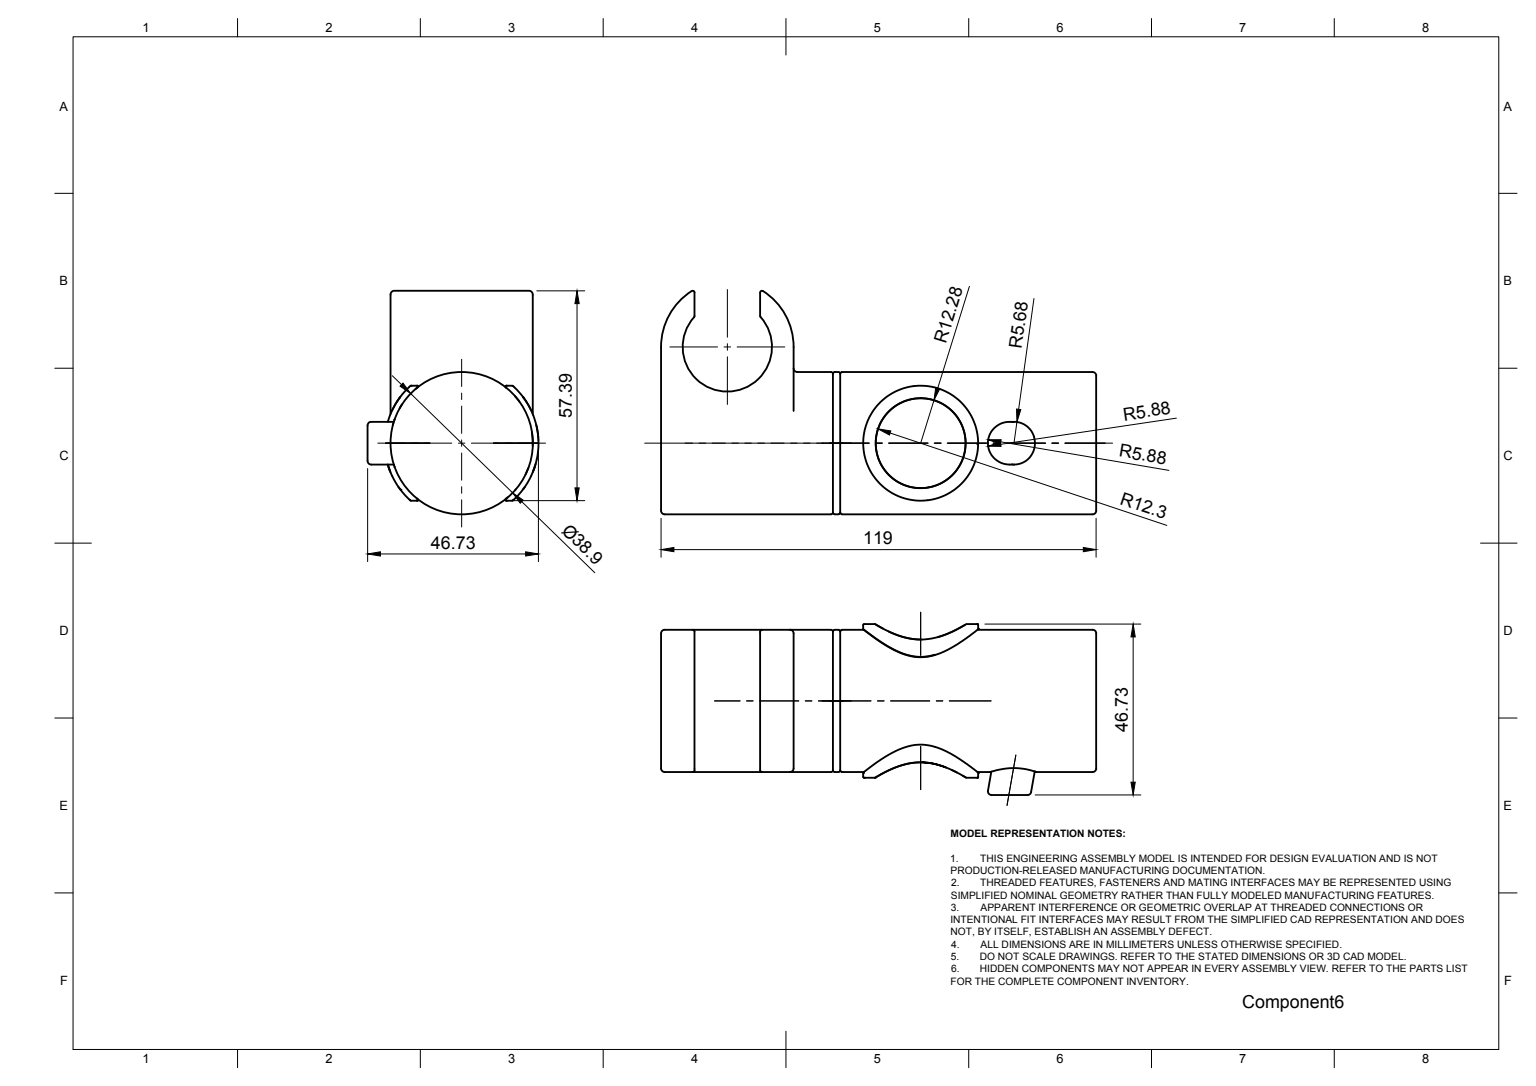
ISO-10303-21;
HEADER;
/* Generated by software containing ST-Developer
 * from STEP Tools, Inc. (www.steptools.com) 
 */

FILE_DESCRIPTION(
/* description */ ('STEP AP214'),
/* implementation_level */ '2;1');

FILE_NAME(
/* name */ 'Component6.step',
/* time_stamp */ '2026-10-06T11:02:40-07:00',
/* author */ (''),
/* organization */ (''),
/* preprocessor_version */ 'ST-DEVELOPER v20.2',
/* originating_system */ 'Autodesk Translation Framework v15.15.0.0',
/* authorisation */ '');

FILE_SCHEMA (('AUTOMOTIVE_DESIGN { 1 0 10303 214 3 1 1 }'));
ENDSEC;

DATA;
#10=MECHANICAL_DESIGN_GEOMETRIC_PRESENTATION_REPRESENTATION('',(#2941),#130910);
#43=(
BOUNDED_CURVE()
B_SPLINE_CURVE(3,(#103309,#103310,#103311,#103312,#103313,#103314,#103315,
#103316,#103317,#103318,#103319,#103320,#103321,#103322,#103323,#103324,
#103325,#103326),.UNSPECIFIED.,.F.,.F.)
B_SPLINE_CURVE_WITH_KNOTS((4,2,2,2,2,2,2,2,4),(0.,0.392699081698724,0.785398163397448,
1.17809724509617,1.5707963267949,1.96349540849362,2.35619449019234,2.74889357189107,
3.14159265358979),.UNSPECIFIED.)
CURVE()
GEOMETRIC_REPRESENTATION_ITEM()
RATIONAL_B_SPLINE_CURVE((1.,1.,1.,1.,1.,1.,1.,1.,1.,1.,1.,1.,1.,1.,1.,1.,
1.,1.))
REPRESENTATION_ITEM('')
);
#44=(
BOUNDED_CURVE()
B_SPLINE_CURVE(3,(#103476,#103477,#103478,#103479,#103480,#103481,#103482,
#103483,#103484,#103485,#103486,#103487,#103488,#103489,#103490,#103491,
#103492,#103493),.UNSPECIFIED.,.F.,.F.)
B_SPLINE_CURVE_WITH_KNOTS((4,2,2,2,2,2,2,2,4),(3.14159265358979,3.53429173528852,
3.92699081698724,4.31968989868597,4.71238898038469,5.10508806208341,5.49778714378214,
5.89048622548086,6.28318530717959),.UNSPECIFIED.)
CURVE()
GEOMETRIC_REPRESENTATION_ITEM()
RATIONAL_B_SPLINE_CURVE((1.,1.,1.,1.,1.,1.,1.,1.,1.,1.,1.,1.,1.,1.,1.,1.,
1.,1.))
REPRESENTATION_ITEM('')
);
#66=SPHERICAL_SURFACE('',#48870,0.5);
#67=SPHERICAL_SURFACE('',#48880,0.5);
#68=SPHERICAL_SURFACE('',#48882,0.5);
#69=SPHERICAL_SURFACE('',#48888,0.5);
#724=FACE_BOUND('',#15265,.T.);
#725=FACE_BOUND('',#15266,.T.);
#726=FACE_BOUND('',#15267,.T.);
#727=FACE_BOUND('',#15278,.T.);
#728=FACE_BOUND('',#15280,.T.);
#729=FACE_BOUND('',#15289,.T.);
#730=FACE_BOUND('',#15291,.T.);
#1660=(
BOUNDED_SURFACE()
B_SPLINE_SURFACE(3,2,((#97421,#97422,#97423),(#97424,#97425,#97426),(#97427,
#97428,#97429),(#97430,#97431,#97432),(#97433,#97434,#97435),(#97436,#97437,
#97438),(#97439,#97440,#97441),(#97442,#97443,#97444),(#97445,#97446,#97447),
(#97448,#97449,#97450),(#97451,#97452,#97453),(#97454,#97455,#97456),(#97457,
#97458,#97459),(#97460,#97461,#97462),(#97463,#97464,#97465),(#97466,#97467,
#97468),(#97469,#97470,#97471),(#97472,#97473,#97474),(#97475,#97476,#97477),
(#97478,#97479,#97480),(#97481,#97482,#97483),(#97484,#97485,#97486),(#97487,
#97488,#97489),(#97490,#97491,#97492),(#97493,#97494,#97495),(#97496,#97497,
#97498),(#97499,#97500,#97501),(#97502,#97503,#97504),(#97505,#97506,#97507),
(#97508,#97509,#97510),(#97511,#97512,#97513),(#97514,#97515,#97516),(#97517,
#97518,#97519),(#97520,#97521,#97522),(#97523,#97524,#97525),(#97526,#97527,
#97528),(#97529,#97530,#97531),(#97532,#97533,#97534),(#97535,#97536,#97537),
(#97538,#97539,#97540),(#97541,#97542,#97543),(#97544,#97545,#97546),(#97547,
#97548,#97549),(#97550,#97551,#97552),(#97553,#97554,#97555),(#97556,#97557,
#97558),(#97559,#97560,#97561),(#97562,#97563,#97564),(#97565,#97566,#97567),
(#97568,#97569,#97570),(#97571,#97572,#97573),(#97574,#97575,#97576),(#97577,
#97578,#97579),(#97580,#97581,#97582),(#97583,#97584,#97585),(#97586,#97587,
#97588),(#97589,#97590,#97591),(#97592,#97593,#97594),(#97595,#97596,#97597),
(#97598,#97599,#97600)),.UNSPECIFIED.,.F.,.F.,.F.)
B_SPLINE_SURFACE_WITH_KNOTS((4,2,2,2,2,2,2,2,2,2,2,2,2,2,2,2,2,2,2,2,2,
2,2,2,2,2,2,2,2,4),(3,3),(-0.00058262743669386,0.00319856320703094,0.00399820400878867,
0.00479784481054641,0.00639712641406187,0.00719676721581961,0.00799640801757734,
0.00959568962109281,0.0111949712246083,0.0127942528281237,0.0159928160351547,
0.0175920976386702,0.0191913792421856,0.0223899424492166,0.023989224052732,
0.0255885056562475,0.027187787259763,0.0279874280615207,0.0287870688632784,
0.0319856320703094,0.0335849136738248,0.0351841952773403,0.0367834768808558,
0.0383827584843712,0.0399820400878867,0.0415813216914022,0.0447798848984331,
0.0463791665019486,0.047978448105464,0.0517596387491888),(0.,1.00058262743669),
 .UNSPECIFIED.)
GEOMETRIC_REPRESENTATION_ITEM()
RATIONAL_B_SPLINE_SURFACE(((1.,0.372615622620617,1.00073106270323),(1.,
0.349888963005402,1.0007575450541),(1.,0.33336913321619,1.00077679486627),
(1.,0.327705676201969,1.00078339423716),(1.,0.327251477944985,1.00078392349389),
(1.,0.327438578938257,1.00078370547354),(1.,0.328073122498965,1.00078296606857),
(1.,0.331521383799571,1.00077894796528),(1.,0.335886927429418,1.00077386099429),
(1.,0.345028662937665,1.00076320854244),(1.,0.348522443164058,1.00075913739801),
(1.,0.356175477316151,1.00075021966266),(1.,0.360329629032238,1.00074537901713),
(1.,0.373578575616019,1.00072994061756),(1.,0.383450575672534,1.00071843722138),
(1.,0.404468341585455,1.00069394616722),(1.,0.415617057266219,1.00068095507195),
(1.,0.438646408868145,1.00065412000776),(1.,0.450439636237964,1.00064037789209),
(1.,0.485738524418637,1.00059924569062),(1.,0.509290450787533,1.00057180169364),
(1.,0.543406923368721,1.0005320473077),(1.,0.554585702870248,1.00051902118041),
(1.,0.576402400431413,1.00049359916725),(1.,0.586915261405066,1.00048134900477),
(1.,0.616896247011513,1.00044641351518),(1.,0.634916789357006,1.00042541499039),
(1.,0.658271057878159,1.00039820131519),(1.,0.665440397537911,1.00038984720721),
(1.,0.678364602785122,1.00037478721406),(1.,0.684003905064955,1.00036821598959),
(1.,0.693490447304963,1.00035716175002),(1.,0.697353099044676,1.00035266077625),
(1.,0.701751933579305,1.00034753501288),(1.,0.702985302217132,1.00034609782406),
(1.,0.704968511748717,1.00034378687949),(1.,0.705717903905829,1.00034291364662),
(1.,0.708180950178283,1.00034004356995),(1.,0.706146530160687,1.00034241418779),
(1.,0.69729017361677,1.00035273410042),(1.,0.693336856914947,1.00035734072197),
(1.,0.683762701080569,1.00036849705371),(1.,0.678128040418911,1.00037506286951),
(1.,0.665292401063798,1.00039001966082),(1.,0.658088068918505,1.00039841454396),
(1.,0.642209400675926,1.00041691723951),(1.,0.633656376746873,1.00042688369233),
(1.,0.615478575266067,1.00044806546409),(1.,0.605853070392858,1.00045928163056),
(1.,0.585652603574339,1.00048282032296),(1.,0.575043134289062,1.00049518305875),
(1.,0.542192039840224,1.00053346295665),(1.,0.519160353863195,1.00056030074098),
(1.,0.483909414581263,1.00060137706977),(1.,0.472043707472279,1.0006152036428),
(1.,0.448330324994361,1.0006428357773),(1.,0.43649600801918,1.00065662577283),
(1.,0.398029999848111,1.00070144847631),(1.,0.372846379395456,1.00073079381277),
(1.,0.353825408000619,1.00075295809239)))
REPRESENTATION_ITEM('')
SURFACE()
);
#1661=(
BOUNDED_SURFACE()
B_SPLINE_SURFACE(3,2,((#97849,#97850,#97851),(#97852,#97853,#97854),(#97855,
#97856,#97857),(#97858,#97859,#97860),(#97861,#97862,#97863),(#97864,#97865,
#97866),(#97867,#97868,#97869),(#97870,#97871,#97872),(#97873,#97874,#97875),
(#97876,#97877,#97878),(#97879,#97880,#97881),(#97882,#97883,#97884),(#97885,
#97886,#97887),(#97888,#97889,#97890),(#97891,#97892,#97893),(#97894,#97895,
#97896),(#97897,#97898,#97899),(#97900,#97901,#97902),(#97903,#97904,#97905),
(#97906,#97907,#97908),(#97909,#97910,#97911),(#97912,#97913,#97914),(#97915,
#97916,#97917),(#97918,#97919,#97920),(#97921,#97922,#97923),(#97924,#97925,
#97926),(#97927,#97928,#97929),(#97930,#97931,#97932),(#97933,#97934,#97935),
(#97936,#97937,#97938),(#97939,#97940,#97941),(#97942,#97943,#97944),(#97945,
#97946,#97947),(#97948,#97949,#97950),(#97951,#97952,#97953),(#97954,#97955,
#97956),(#97957,#97958,#97959),(#97960,#97961,#97962),(#97963,#97964,#97965),
(#97966,#97967,#97968),(#97969,#97970,#97971),(#97972,#97973,#97974),(#97975,
#97976,#97977),(#97978,#97979,#97980),(#97981,#97982,#97983),(#97984,#97985,
#97986),(#97987,#97988,#97989),(#97990,#97991,#97992),(#97993,#97994,#97995),
(#97996,#97997,#97998),(#97999,#98000,#98001),(#98002,#98003,#98004)),
 .UNSPECIFIED.,.F.,.F.,.F.)
B_SPLINE_SURFACE_WITH_KNOTS((4,2,2,2,2,2,2,2,2,2,2,2,2,2,2,2,2,2,2,2,2,
2,2,2,2,4),(3,3),(0.,0.00315886476497431,0.00473829714746146,0.00631772952994861,
0.00789716191243577,0.00947659429492292,0.0126354590598972,0.0142148914423844,
0.0157943238248715,0.0189531885898458,0.0221120533548201,0.0236914857373073,
0.0252709181197944,0.0268503505022816,0.0284297828847688,0.0315886476497431,
0.0331680800322302,0.0347475124147174,0.0363269447972045,0.0379063771796917,
0.041065241944666,0.0426446743271531,0.0442241067096403,0.0473829714746146,
0.0489624038571017,0.0509081571689574),(-0.000366320929394054,1.),
 .UNSPECIFIED.)
GEOMETRIC_REPRESENTATION_ITEM()
RATIONAL_B_SPLINE_SURFACE(((1.00005042977931,0.931167215319011,1.),(1.00004802363142,
0.934451422823265,1.),(1.00004766638974,0.934939030352376,1.),(1.00005016915153,
0.931522952280194,1.),(1.00005152792892,0.92966832525533,1.),(1.00005514272126,
0.924734410684191,1.),(1.00005739708062,0.921657382894737,1.),(1.00006270960761,
0.914406190616929,1.),(1.00006578664498,0.910206270369143,1.),(1.00007258454286,
0.900927660639692,1.),(1.00007629268405,0.89586633205052,1.),(1.0000882084061,
0.879602284474657,1.),(1.00009720731593,0.867319462069032,1.),(1.00011185421907,
0.847327561573564,1.),(1.00011692583641,0.840405192509689,1.),(1.00012717668813,
0.826413565365098,1.),(1.00013237821318,0.819313882232296,1.),(1.00014804138246,
0.797934856318314,1.),(1.00015859373613,0.783531702112416,1.),(1.00017861952009,
0.756198041441388,1.),(1.00018776819113,0.743710806479728,1.),(1.00019903767144,
0.728328829354908,1.),(1.00020239085733,0.723751987553838,1.),(1.00020800234017,
0.716092743446008,1.),(1.00021021837205,0.713068029719533,1.),(1.00021337561237,
0.708758638603594,1.),(1.00021431665381,0.707474189140747,1.),(1.00021485246247,
0.70674285137928,1.),(1.0002144426404,0.707302227096993,1.),(1.00021115809343,
0.711785382037871,1.),(1.00020631623579,0.718394146723749,1.),(1.00019606386371,
0.732387849048684,1.),(1.0001921234338,0.737766233939451,1.),(1.0001836019673,
0.74939738277055,1.),(1.00017901501663,0.755658218975225,1.),(1.00016939628292,
0.768787053474939,1.),(1.00016436417741,0.775655491921232,1.),(1.00015402891774,
0.789762329443024,1.),(1.00014872894768,0.796996382481174,1.),(1.00013293409498,
0.818555146164889,1.),(1.00012245640244,0.832856393646782,1.),(1.00010747739276,
0.853301594132862,1.),(1.0001025893796,0.859973357550685,1.),(1.00009330215817,
0.872649703192738,1.),(1.00008888539535,0.878678246012862,1.),(1.00007641546784,
0.895698741577217,1.),(1.00006912991505,0.905642962900587,1.),(1.00006026267051,
0.917746072269067,1.),(1.00005766031332,0.921298090426901,1.),(1.00005289421335,
0.927803451699111,1.),(1.00005093853036,0.930472809118457,1.),(1.00004972550474,
0.932128496152477,1.)))
REPRESENTATION_ITEM('')
SURFACE()
);
#1662=(
BOUNDED_SURFACE()
B_SPLINE_SURFACE(3,2,((#98299,#98300,#98301),(#98302,#98303,#98304),(#98305,
#98306,#98307),(#98308,#98309,#98310),(#98311,#98312,#98313),(#98314,#98315,
#98316),(#98317,#98318,#98319),(#98320,#98321,#98322),(#98323,#98324,#98325),
(#98326,#98327,#98328),(#98329,#98330,#98331),(#98332,#98333,#98334),(#98335,
#98336,#98337),(#98338,#98339,#98340),(#98341,#98342,#98343),(#98344,#98345,
#98346),(#98347,#98348,#98349),(#98350,#98351,#98352),(#98353,#98354,#98355),
(#98356,#98357,#98358),(#98359,#98360,#98361),(#98362,#98363,#98364),(#98365,
#98366,#98367),(#98368,#98369,#98370),(#98371,#98372,#98373),(#98374,#98375,
#98376),(#98377,#98378,#98379),(#98380,#98381,#98382),(#98383,#98384,#98385),
(#98386,#98387,#98388),(#98389,#98390,#98391),(#98392,#98393,#98394),(#98395,
#98396,#98397),(#98398,#98399,#98400),(#98401,#98402,#98403),(#98404,#98405,
#98406),(#98407,#98408,#98409),(#98410,#98411,#98412),(#98413,#98414,#98415),
(#98416,#98417,#98418),(#98419,#98420,#98421),(#98422,#98423,#98424),(#98425,
#98426,#98427),(#98428,#98429,#98430),(#98431,#98432,#98433),(#98434,#98435,
#98436),(#98437,#98438,#98439),(#98440,#98441,#98442),(#98443,#98444,#98445),
(#98446,#98447,#98448)),.UNSPECIFIED.,.F.,.F.,.F.)
B_SPLINE_SURFACE_WITH_KNOTS((4,2,2,2,2,2,2,2,2,2,2,2,2,2,2,2,2,2,2,2,2,
2,2,2,4),(3,3),(0.,0.0025187116162184,0.00377806742432761,0.00503742323243681,
0.00629677904054601,0.00755613484865521,0.0100748464648736,0.0113342022729828,
0.012593558081092,0.0151122696973104,0.0163716255054196,0.0176309813135288,
0.018890337121638,0.0201496929297472,0.0226684045459656,0.0239277603540748,
0.025187116162184,0.0264464719702932,0.0277058277784024,0.0302245393946208,
0.0327432510108392,0.0352619626270576,0.0365213184351669,0.0377806742432761,
0.0402993858594945),(0.,1.),.UNSPECIFIED.)
GEOMETRIC_REPRESENTATION_ITEM()
RATIONAL_B_SPLINE_SURFACE(((1.,0.444837807664136,1.),(1.,0.443889729175589,
1.),(1.,0.447748071183855,1.),(1.,0.459453142902776,1.),(1.,0.464367346379585,
1.),(1.,0.475717163519536,1.),(1.,0.48211295799902,1.),(1.,0.495944712524718,
1.),(1.,0.503380981743553,1.),(1.,0.518962657925113,1.),(1.,0.527139185789211,
1.),(1.,0.551895636149689,1.),(1.,0.568781778812327,1.),(1.,0.593444445481799,
1.),(1.,0.601597343431266,1.),(1.,0.61732836948322,1.),(1.,0.624889681210996,
1.),(1.,0.646485984307859,1.),(1.,0.659441840352202,1.),(1.,0.675982223306384,
1.),(1.,0.68102172685123,1.),(1.,0.689763664719054,1.),(1.,0.693504359158594,
1.),(1.,0.69968025928586,1.),(1.,0.702115682658639,1.),(1.,0.705612781075522,
1.),(1.,0.706675637348199,1.),(1.,0.707648224727786,1.),(1.,0.705356532405246,
1.),(1.,0.697802511437167,1.),(1.,0.69458157237586,1.),(1.,0.686829651284654,
1.),(1.,0.682347030399091,1.),(1.,0.672289714801745,1.),(1.,0.666714572428337,
1.),(1.,0.654569105179005,1.),(1.,0.647967838573232,1.),(1.,0.627025457575446,
1.),(1.,0.611679454062546,1.),(1.,0.579351199094756,1.),(1.,0.56222647842645,
1.),(1.,0.529022354961919,1.),(1.,0.512804015742491,1.),(1.,0.490778638607675,
1.),(1.,0.48379298434534,1.),(1.,0.471266214350623,1.),(1.,0.46570913806108,
1.),(1.,0.451670624760032,1.),(1.,0.445830006853561,1.),(1.,0.444857616465186,
1.)))
REPRESENTATION_ITEM('')
SURFACE()
);
#1663=(
BOUNDED_SURFACE()
B_SPLINE_SURFACE(3,2,((#99274,#99275,#99276),(#99277,#99278,#99279),(#99280,
#99281,#99282),(#99283,#99284,#99285),(#99286,#99287,#99288),(#99289,#99290,
#99291),(#99292,#99293,#99294),(#99295,#99296,#99297),(#99298,#99299,#99300),
(#99301,#99302,#99303),(#99304,#99305,#99306),(#99307,#99308,#99309),(#99310,
#99311,#99312),(#99313,#99314,#99315),(#99316,#99317,#99318),(#99319,#99320,
#99321),(#99322,#99323,#99324),(#99325,#99326,#99327),(#99328,#99329,#99330),
(#99331,#99332,#99333),(#99334,#99335,#99336),(#99337,#99338,#99339),(#99340,
#99341,#99342),(#99343,#99344,#99345),(#99346,#99347,#99348),(#99349,#99350,
#99351),(#99352,#99353,#99354),(#99355,#99356,#99357),(#99358,#99359,#99360),
(#99361,#99362,#99363),(#99364,#99365,#99366),(#99367,#99368,#99369),(#99370,
#99371,#99372),(#99373,#99374,#99375),(#99376,#99377,#99378),(#99379,#99380,
#99381),(#99382,#99383,#99384),(#99385,#99386,#99387),(#99388,#99389,#99390),
(#99391,#99392,#99393),(#99394,#99395,#99396),(#99397,#99398,#99399),(#99400,
#99401,#99402),(#99403,#99404,#99405),(#99406,#99407,#99408),(#99409,#99410,
#99411)),.UNSPECIFIED.,.F.,.F.,.F.)
B_SPLINE_SURFACE_WITH_KNOTS((4,2,2,2,2,2,2,2,2,2,2,2,2,2,2,2,2,2,2,2,2,
2,4),(3,3),(0.,0.00125459591840773,0.0018818938776116,0.00250919183681547,
0.0037637877552232,0.00439108571442707,0.00501838367363094,0.00564568163283481,
0.00627297959203867,0.00752757551044641,0.00878217142885414,0.0100367673472619,
0.0106640653064657,0.0112913632656696,0.0125459591840773,0.0138005551024851,
0.0144278530616889,0.0150551510208928,0.0163097469393006,0.0169370448985044,
0.0175643428577083,0.018818938776116,0.0200735346945238),(0.,1.),
 .UNSPECIFIED.)
GEOMETRIC_REPRESENTATION_ITEM()
RATIONAL_B_SPLINE_SURFACE(((1.,0.753501700966988,1.),(1.,0.758919966590289,
1.),(1.,0.762624474007346,1.),(1.,0.765493967892479,1.),(1.,0.766001864196328,
1.),(1.,0.766081899420437,1.),(1.,0.765645177532698,1.),(1.,0.762965796826428,
1.),(1.,0.75937217675435,1.),(1.,0.751475581705692,1.),(1.,0.748410443135639,
1.),(1.,0.741628592661977,1.),(1.,0.737899758372927,1.),(1.,0.729842420453465,
1.),(1.,0.725513701271151,1.),(1.,0.716322621401233,1.),(1.,0.71144077787533,
1.),(1.,0.696381444937169,1.),(1.,0.685722488457871,1.),(1.,0.663879284854164,
1.),(1.,0.652645530876282,1.),(1.,0.631293420609983,1.),(1.,0.621067849093089,
1.),(1.,0.607073245214128,1.),(1.,0.602619800288969,1.),(1.,0.594464909703987,
1.),(1.,0.590739984910806,1.),(1.,0.580731511515441,1.),(1.,0.575617470391927,
1.),(1.,0.569031517938587,1.),(1.,0.567674325666079,1.),(1.,0.568262977064503,
1.),(1.,0.568891116188093,1.),(1.,0.570935397635918,1.),(1.,0.572362568136071,
1.),(1.,0.577560685048605,1.),(1.,0.582247188120323,1.),(1.,0.59023516464793,
1.),(1.,0.593074756205356,1.),(1.,0.598856135494127,1.),(1.,0.601790038290455,
1.),(1.,0.610522818926502,1.),(1.,0.616249874441583,1.),(1.,0.626614400505202,
1.),(1.,0.631088239307343,1.),(1.,0.634563057406884,1.)))
REPRESENTATION_ITEM('')
SURFACE()
);
#1664=(
BOUNDED_SURFACE()
B_SPLINE_SURFACE(3,2,((#99754,#99755,#99756),(#99757,#99758,#99759),(#99760,
#99761,#99762),(#99763,#99764,#99765),(#99766,#99767,#99768),(#99769,#99770,
#99771),(#99772,#99773,#99774),(#99775,#99776,#99777),(#99778,#99779,#99780),
(#99781,#99782,#99783),(#99784,#99785,#99786),(#99787,#99788,#99789),(#99790,
#99791,#99792),(#99793,#99794,#99795),(#99796,#99797,#99798),(#99799,#99800,
#99801),(#99802,#99803,#99804),(#99805,#99806,#99807),(#99808,#99809,#99810),
(#99811,#99812,#99813),(#99814,#99815,#99816),(#99817,#99818,#99819),(#99820,
#99821,#99822),(#99823,#99824,#99825),(#99826,#99827,#99828),(#99829,#99830,
#99831),(#99832,#99833,#99834),(#99835,#99836,#99837),(#99838,#99839,#99840),
(#99841,#99842,#99843),(#99844,#99845,#99846),(#99847,#99848,#99849),(#99850,
#99851,#99852),(#99853,#99854,#99855),(#99856,#99857,#99858),(#99859,#99860,
#99861),(#99862,#99863,#99864),(#99865,#99866,#99867),(#99868,#99869,#99870),
(#99871,#99872,#99873),(#99874,#99875,#99876),(#99877,#99878,#99879),(#99880,
#99881,#99882),(#99883,#99884,#99885),(#99886,#99887,#99888),(#99889,#99890,
#99891),(#99892,#99893,#99894),(#99895,#99896,#99897),(#99898,#99899,#99900),
(#99901,#99902,#99903),(#99904,#99905,#99906),(#99907,#99908,#99909),(#99910,
#99911,#99912),(#99913,#99914,#99915)),.UNSPECIFIED.,.F.,.F.,.F.)
B_SPLINE_SURFACE_WITH_KNOTS((4,2,2,2,2,2,2,2,2,2,2,2,2,2,2,2,2,2,2,2,2,
2,2,2,2,2,4),(3,3),(-7.78153428745613E-5,0.00257554787859691,0.00386332181789536,
0.00515109575719382,0.00643886969649227,0.00772664363579073,0.0103021915143876,
0.0115899654536861,0.0128777393929845,0.0154532872715815,0.0167410612108799,
0.0180288351501784,0.0193166090894768,0.0206043830287753,0.0231799309073722,
0.0244677048466706,0.0257554787859691,0.0270432527252676,0.028331026664566,
0.0309065745431629,0.0321943484824614,0.0334821224217598,0.0347698963610583,
0.0360576703003567,0.0386332181789536,0.0399209921182521,0.0412865814003949),
(-5.57615391788296E-5,1.00007781534287),.UNSPECIFIED.)
GEOMETRIC_REPRESENTATION_ITEM()
RATIONAL_B_SPLINE_SURFACE(((1.00006499666788,0.417145519460541,1.00009070498426),
(1.00006613373744,0.406948903154154,1.00009229180215),(1.00006666002296,
0.402229463167758,1.00009302625088),(1.00006643124968,0.404280976494946,
1.00009270699026),(1.00006619616633,0.406389075066969,1.00009237892372),
(1.00006542207527,0.413330699283567,1.00009129865423),(1.00006489161556,
0.418087571101604,1.00009055838029),(1.00006360370812,0.429636818858515,
1.00008876106317),(1.00006284644101,0.436427575124811,1.00008770427205),
(1.00006116075035,0.451543924676617,1.00008535183539),(1.00006022957763,
0.459894171148586,1.00008405235327),(1.00005731845811,0.485999494820791,
1.0000799897904),(1.00005520865809,0.504919024658453,1.00007704549518),
(1.00005200598796,0.533638814326789,1.00007257606387),(1.00005092886496,
0.543297862838644,1.00007107290335),(1.00004879117353,0.562467507505169,
1.00006808968476),(1.00004774201681,0.571875769700711,1.00006662555212),
(1.00004468046442,0.599330092951599,1.00006235305522),(1.00004275366152,
0.616608604952205,1.0000596641385),(1.00004012772931,0.640156525218429,
1.00005599956388),(1.00003929341804,0.647638171228524,1.00005483525511),
(1.00003776153149,0.661375289848644,1.00005269745713),(1.00003706001501,
0.667666105061143,1.00005171846784),(1.00003579596344,0.679001426435143,
1.00004995444238),(1.00003523337831,0.684046381465567,1.00004916933635),
(1.00003426031965,0.692772237972241,1.00004781140104),(1.00003384837915,
0.696466294543873,1.00004723652454),(1.00003288787868,0.705079536093434,
1.0000458961146),(1.00003260121688,0.707650161916355,1.00004549606865),
(1.00003271698939,0.706611977550149,1.00004565763299),(1.0000328491286,
0.705427025561222,1.00004584203759),(1.0000332924415,0.701451638594737,
1.00004646069529),(1.00003360204356,0.6986752970103,1.00004689275514),(1.00003438648853,
0.691640824637982,1.00004798747386),(1.00003486136748,0.687382370582247,
1.00004865018302),(1.00003596953549,0.677444927484954,1.00005019666787),
(1.0000366053434,0.671743350745739,1.00005108395868),(1.00003869257694,
0.653026184786068,1.00005399676162),(1.00004033354564,0.638310877237478,
1.00005628678732),(1.00004309135935,0.613580315885842,1.00006013540692),
(1.00004405946053,0.604898915345222,1.0000614864239),(1.00004604481265,
0.587095366038472,1.00006425704798),(1.00004706626934,0.577935502541562,
1.00006568252433),(1.00004914915559,0.559257320686793,1.00006858926048),
(1.00005021068348,0.549738120586547,1.00007007065751),(1.00005235335541,
0.530523813480548,1.00007306082655),(1.00005343979317,0.520781235371959,
1.00007457698611),(1.00005663467271,0.492131307351429,1.00007903554542),
(1.00005869139382,0.4736877601911,1.00008190576725),(1.00006143077889,0.449122456788815,
1.00008572866908),(1.00006228506745,0.44146166545061,1.00008692085681),
(1.00006386334166,0.427308567599321,1.0000891233903),(1.00006457824779,
0.420897681437532,1.00009012106528),(1.00006512941961,0.415955074725545,
1.00009089024365)))
REPRESENTATION_ITEM('')
SURFACE()
);
#1665=(
BOUNDED_SURFACE()
B_SPLINE_SURFACE(3,2,((#100046,#100047,#100048),(#100049,#100050,#100051),
(#100052,#100053,#100054),(#100055,#100056,#100057),(#100058,#100059,#100060),
(#100061,#100062,#100063),(#100064,#100065,#100066),(#100067,#100068,#100069),
(#100070,#100071,#100072),(#100073,#100074,#100075),(#100076,#100077,#100078),
(#100079,#100080,#100081),(#100082,#100083,#100084),(#100085,#100086,#100087),
(#100088,#100089,#100090),(#100091,#100092,#100093),(#100094,#100095,#100096),
(#100097,#100098,#100099),(#100100,#100101,#100102),(#100103,#100104,#100105),
(#100106,#100107,#100108),(#100109,#100110,#100111),(#100112,#100113,#100114),
(#100115,#100116,#100117),(#100118,#100119,#100120),(#100121,#100122,#100123),
(#100124,#100125,#100126),(#100127,#100128,#100129),(#100130,#100131,#100132),
(#100133,#100134,#100135),(#100136,#100137,#100138),(#100139,#100140,#100141),
(#100142,#100143,#100144),(#100145,#100146,#100147),(#100148,#100149,#100150),
(#100151,#100152,#100153),(#100154,#100155,#100156),(#100157,#100158,#100159),
(#100160,#100161,#100162),(#100163,#100164,#100165),(#100166,#100167,#100168),
(#100169,#100170,#100171),(#100172,#100173,#100174),(#100175,#100176,#100177),
(#100178,#100179,#100180),(#100181,#100182,#100183),(#100184,#100185,#100186),
(#100187,#100188,#100189),(#100190,#100191,#100192),(#100193,#100194,#100195),
(#100196,#100197,#100198),(#100199,#100200,#100201),(#100202,#100203,#100204),
(#100205,#100206,#100207)),.UNSPECIFIED.,.F.,.F.,.F.)
B_SPLINE_SURFACE_WITH_KNOTS((4,2,2,2,2,2,2,2,2,2,2,2,2,2,2,2,2,2,2,2,2,
2,2,2,2,2,4),(3,3),(-7.78153430528562E-5,0.00257554787859691,0.00386332181789536,
0.00515109575719382,0.00643886969649227,0.00772664363579073,0.0103021915143876,
0.0115899654536861,0.0128777393929845,0.0154532872715815,0.0167410612108799,
0.0180288351501784,0.0193166090894768,0.0206043830287753,0.0231799309073722,
0.0244677048466706,0.0257554787859691,0.0270432527252676,0.028331026664566,
0.0309065745431629,0.0321943484824614,0.0334821224217598,0.0347698963610583,
0.0360576703003567,0.0386332181789536,0.0399209921182521,0.0412865814005733),
(-5.57615387946816E-5,1.00007781534305),.UNSPECIFIED.)
GEOMETRIC_REPRESENTATION_ITEM()
RATIONAL_B_SPLINE_SURFACE(((1.00006499666744,0.417145519462717,1.00009070498446),
(1.00006613373698,0.406948903154911,1.00009229180236),(1.0000666600225,
0.402229463167788,1.00009302625109),(1.00006643124922,0.404280976495069,
1.00009270699047),(1.00006619616587,0.406389075067091,1.00009237892394),
(1.00006542207482,0.413330699283688,1.00009129865444),(1.00006489161511,
0.418087571101724,1.0000905583805),(1.00006360370768,0.429636818858632,
1.00008876106337),(1.00006284644058,0.436427575124927,1.00008770427225),
(1.00006116074993,0.45154392467673,1.00008535183558),(1.00006022957721,
0.459894171148698,1.00008405235346),(1.00005731845772,0.485999494820897,
1.00007998979058),(1.00005520865771,0.504919024658555,1.00007704549536),
(1.0000520059876,0.533638814326885,1.00007257606403),(1.00005092886461,
0.543297862838738,1.00007107290351),(1.00004879117319,0.562467507505259,
1.00006808968492),(1.00004774201649,0.571875769700799,1.00006662555227),
(1.00004468046411,0.599330092951681,1.00006235305536),(1.00004275366122,
0.616608604952284,1.00005966413864),(1.00004012772903,0.640156525218503,
1.00005599956401),(1.00003929341777,0.647638171228596,1.00005483525523),
(1.00003776153123,0.661375289848713,1.00005269745725),(1.00003706001475,
0.667666105061211,1.00005171846796),(1.00003579596319,0.679001426435209,
1.00004995444249),(1.00003523337806,0.684046381465632,1.00004916933646),
(1.00003426031941,0.692772237972305,1.00004781140115),(1.00003384837891,
0.696466294543935,1.00004723652465),(1.00003288787845,0.705079536093495,
1.00004589611471),(1.00003260121666,0.707650161916415,1.00004549606876),
(1.00003271698917,0.706611977550209,1.00004565763309),(1.00003284912838,
0.705427025561283,1.0000458420377),(1.00003329244127,0.701451638594799,
1.0000464606954),(1.00003360204333,0.698675297010362,1.00004689275525),
(1.00003438648829,0.691640824638045,1.00004798747396),(1.00003486136724,
0.687382370582311,1.00004865018313),(1.00003596953524,0.677444927485021,
1.00005019666798),(1.00003660534315,0.671743350745806,1.0000510839588),
(1.00003869257667,0.653026184786139,1.00005399676175),(1.00004033354536,
0.638310877237552,1.00005628678745),(1.00004309135906,0.613580315885922,
1.00006013540706),(1.00004405946023,0.604898915345303,1.00006148642404),
(1.00004604481234,0.587095366038557,1.00006425704813),(1.00004706626902,
0.577935502541649,1.00006568252448),(1.00004914915525,0.559257320686884,
1.00006858926064),(1.00005021068313,0.54973812058664,1.00007007065767),
(1.00005235335505,0.530523813480645,1.00007306082672),(1.0000534397928,
0.520781235372058,1.00007457698628),(1.00005663467232,0.492131307351533,
1.0000790355456),(1.00005869139341,0.473687760191208,1.00008190576744),
(1.00006143077847,0.449122456788928,1.00008572866928),(1.00006228506702,
0.441461665450725,1.000086920857),(1.00006386334123,0.427308567598488,1.00008912339051),
(1.00006457824735,0.420897681435977,1.00009012106548),(1.00006512941917,
0.415955074723729,1.00009089024386)))
REPRESENTATION_ITEM('')
SURFACE()
);
#1666=(
BOUNDED_SURFACE()
B_SPLINE_SURFACE(3,2,((#101435,#101436,#101437),(#101438,#101439,#101440),
(#101441,#101442,#101443),(#101444,#101445,#101446),(#101447,#101448,#101449),
(#101450,#101451,#101452),(#101453,#101454,#101455),(#101456,#101457,#101458),
(#101459,#101460,#101461),(#101462,#101463,#101464),(#101465,#101466,#101467),
(#101468,#101469,#101470),(#101471,#101472,#101473),(#101474,#101475,#101476),
(#101477,#101478,#101479),(#101480,#101481,#101482),(#101483,#101484,#101485),
(#101486,#101487,#101488),(#101489,#101490,#101491),(#101492,#101493,#101494),
(#101495,#101496,#101497),(#101498,#101499,#101500),(#101501,#101502,#101503),
(#101504,#101505,#101506),(#101507,#101508,#101509),(#101510,#101511,#101512),
(#101513,#101514,#101515),(#101516,#101517,#101518),(#101519,#101520,#101521),
(#101522,#101523,#101524),(#101525,#101526,#101527),(#101528,#101529,#101530),
(#101531,#101532,#101533),(#101534,#101535,#101536),(#101537,#101538,#101539),
(#101540,#101541,#101542),(#101543,#101544,#101545),(#101546,#101547,#101548),
(#101549,#101550,#101551),(#101552,#101553,#101554),(#101555,#101556,#101557),
(#101558,#101559,#101560),(#101561,#101562,#101563),(#101564,#101565,#101566),
(#101567,#101568,#101569),(#101570,#101571,#101572),(#101573,#101574,#101575),
(#101576,#101577,#101578),(#101579,#101580,#101581),(#101582,#101583,#101584),
(#101585,#101586,#101587),(#101588,#101589,#101590),(#101591,#101592,#101593),
(#101594,#101595,#101596),(#101597,#101598,#101599),(#101600,#101601,#101602),
(#101603,#101604,#101605),(#101606,#101607,#101608),(#101609,#101610,#101611),
(#101612,#101613,#101614)),.UNSPECIFIED.,.F.,.F.,.F.)
B_SPLINE_SURFACE_WITH_KNOTS((4,2,2,2,2,2,2,2,2,2,2,2,2,2,2,2,2,2,2,2,2,
2,2,2,2,2,2,2,2,4),(3,3),(-0.000582627436703559,0.00319856320703094,0.00399820400878867,
0.00479784481054641,0.00639712641406187,0.00719676721581961,0.00799640801757734,
0.00959568962109281,0.0111949712246083,0.0127942528281237,0.0159928160351547,
0.0175920976386702,0.0191913792421856,0.0223899424492166,0.023989224052732,
0.0255885056562475,0.027187787259763,0.0279874280615207,0.0287870688632784,
0.0319856320703094,0.0335849136738248,0.0351841952773403,0.0367834768808558,
0.0383827584843712,0.0399820400878867,0.0415813216914022,0.0447798848984331,
0.0463791665019486,0.047978448105464,0.0517596387491986),(-0.000582627436703563,
1.),.UNSPECIFIED.)
GEOMETRIC_REPRESENTATION_ITEM()
RATIONAL_B_SPLINE_SURFACE(((1.00073106270324,0.372615622620786,1.),(1.00075754505411,
0.34988896300548,1.),(1.00077679486628,0.333369133216196,1.),(1.00078339423717,
0.327705676201963,1.),(1.0007839234939,0.327251477944978,1.),(1.00078370547356,
0.327438578938251,1.),(1.00078296606858,0.328073122498959,1.),(1.0007789479653,
0.331521383799564,1.),(1.00077386099431,0.335886927429411,1.),(1.00076320854245,
0.345028662937659,1.),(1.00075913739802,0.348522443164051,1.),(1.00075021966268,
0.356175477316145,1.),(1.00074537901714,0.360329629032232,1.),(1.00072994061757,
0.373578575616013,1.),(1.00071843722139,0.383450575672528,1.),(1.00069394616724,
0.404468341585449,1.),(1.00068095507196,0.415617057266214,1.),(1.00065412000777,
0.438646408868139,1.),(1.0006403778921,0.450439636237959,1.),(1.00059924569063,
0.485738524418632,1.),(1.00057180169365,0.509290450787528,1.),(1.00053204730771,
0.543406923368716,1.),(1.00051902118042,0.554585702870244,1.),(1.00049359916726,
0.576402400431409,1.),(1.00048134900478,0.586915261405062,1.),(1.00044641351519,
0.616896247011509,1.),(1.0004254149904,0.634916789357002,1.),(1.00039820131519,
0.658271057878156,1.),(1.00038984720721,0.665440397537908,1.),(1.00037478721406,
0.678364602785118,1.),(1.0003682159896,0.684003905064952,1.),(1.00035716175002,
0.69349044730496,1.),(1.00035266077626,0.697353099044673,1.),(1.00034753501288,
0.701751933579303,1.),(1.00034609782407,0.702985302217129,1.),(1.00034378687949,
0.704968511748714,1.),(1.00034291364663,0.705717903905826,1.),(1.00034004356996,
0.70818095017828,1.),(1.0003424141878,0.706146530160684,1.),(1.00035273410042,
0.697290173616767,1.),(1.00035734072197,0.693336856914944,1.),(1.00036849705372,
0.683762701080566,1.),(1.00037506286951,0.678128040418907,1.),(1.00039001966083,
0.665292401063795,1.),(1.00039841454397,0.658088068918501,1.),(1.00041691723952,
0.642209400675922,1.),(1.00042688369234,0.633656376746869,1.),(1.0004480654641,
0.615478575266063,1.),(1.00045928163056,0.605853070392854,1.),(1.00048282032297,
0.585652603574335,1.),(1.00049518305876,0.575043134289058,1.),(1.00053346295666,
0.542192039840219,1.),(1.00056030074099,0.51916035386319,1.),(1.00060137706978,
0.483909414581257,1.),(1.00061520364281,0.472043707472274,1.),(1.00064283577731,
0.448330324994356,1.),(1.00065662577284,0.436496008019175,1.),(1.00070144847632,
0.398029999848035,1.),(1.00073079381278,0.37284637939532,1.),(1.0007529580924,
0.353825408000466,1.)))
REPRESENTATION_ITEM('')
SURFACE()
);
#1667=(
BOUNDED_SURFACE()
B_SPLINE_SURFACE(3,2,((#101803,#101804,#101805),(#101806,#101807,#101808),
(#101809,#101810,#101811),(#101812,#101813,#101814),(#101815,#101816,#101817),
(#101818,#101819,#101820),(#101821,#101822,#101823),(#101824,#101825,#101826),
(#101827,#101828,#101829),(#101830,#101831,#101832),(#101833,#101834,#101835),
(#101836,#101837,#101838),(#101839,#101840,#101841),(#101842,#101843,#101844),
(#101845,#101846,#101847),(#101848,#101849,#101850),(#101851,#101852,#101853),
(#101854,#101855,#101856),(#101857,#101858,#101859),(#101860,#101861,#101862),
(#101863,#101864,#101865),(#101866,#101867,#101868),(#101869,#101870,#101871),
(#101872,#101873,#101874),(#101875,#101876,#101877),(#101878,#101879,#101880),
(#101881,#101882,#101883),(#101884,#101885,#101886),(#101887,#101888,#101889),
(#101890,#101891,#101892),(#101893,#101894,#101895),(#101896,#101897,#101898),
(#101899,#101900,#101901),(#101902,#101903,#101904),(#101905,#101906,#101907),
(#101908,#101909,#101910),(#101911,#101912,#101913),(#101914,#101915,#101916),
(#101917,#101918,#101919),(#101920,#101921,#101922),(#101923,#101924,#101925),
(#101926,#101927,#101928),(#101929,#101930,#101931),(#101932,#101933,#101934),
(#101935,#101936,#101937),(#101938,#101939,#101940),(#101941,#101942,#101943),
(#101944,#101945,#101946),(#101947,#101948,#101949),(#101950,#101951,#101952),
(#101953,#101954,#101955),(#101956,#101957,#101958)),.UNSPECIFIED.,.F.,
 .F.,.F.)
B_SPLINE_SURFACE_WITH_KNOTS((4,2,2,2,2,2,2,2,2,2,2,2,2,2,2,2,2,2,2,2,2,
2,2,2,2,4),(3,3),(0.,0.00315886476497431,0.00473829714746146,0.00631772952994861,
0.00789716191243577,0.00947659429492292,0.0126354590598972,0.0142148914423844,
0.0157943238248715,0.0189531885898458,0.0221120533548201,0.0236914857373073,
0.0252709181197944,0.0268503505022816,0.0284297828847688,0.0315886476497431,
0.0331680800322302,0.0347475124147174,0.0363269447972045,0.0379063771796917,
0.041065241944666,0.0426446743271531,0.0442241067096403,0.0473829714746146,
0.0489624038571017,0.0509081571686288),(0.,1.00036632092907),
 .UNSPECIFIED.)
GEOMETRIC_REPRESENTATION_ITEM()
RATIONAL_B_SPLINE_SURFACE(((1.,0.931167215319034,1.00005042977927),(1.,
0.934451422823286,1.00004802363138),(1.,0.934939030352398,1.00004766638969),
(1.,0.931522952280216,1.00005016915148),(1.,0.929668325255353,1.00005152792887),
(1.,0.924734410684215,1.00005514272121),(1.,0.921657382894763,1.00005739708057),
(1.,0.914406190616957,1.00006270960755),(1.,0.910206270369172,1.00006578664493),
(1.,0.900927660639724,1.0000725845428),(1.,0.895866332050554,1.00007629268398),
(1.,0.879602284474697,1.00008820840602),(1.,0.867319462069075,1.00009720731585),
(1.,0.847327561573614,1.00011185421897),(1.,0.840405192509742,1.00011692583631),
(1.,0.826413565365155,1.00012717668802),(1.,0.819313882232356,1.00013237821306),
(1.,0.797934856318381,1.00014804138233),(1.,0.783531702112487,1.00015859373599),
(1.,0.756198041441468,1.00017861951993),(1.,0.743710806479812,1.00018776819096),
(1.,0.728328829354997,1.00019903767126),(1.,0.723751987553928,1.00020239085714),
(1.,0.716092743446101,1.00020800233998),(1.,0.713068029719627,1.00021021837186),
(1.,0.708758638603689,1.00021337561218),(1.,0.707474189140843,1.00021431665362),
(1.,0.706742851379377,1.00021485246228),(1.,0.70730222709709,1.00021444264021),
(1.,0.711785382037965,1.00021115809324),(1.,0.718394146723841,1.0002063162356),
(1.,0.732387849048772,1.00019606386353),(1.,0.737766233939537,1.00019212343363),
(1.,0.749397382770632,1.00018360196714),(1.,0.755658218975305,1.00017901501647),
(1.,0.768787053475015,1.00016939628277),(1.,0.775655491921306,1.00016436417726),
(1.,0.789762329443093,1.00015402891761),(1.,0.79699638248124,1.00014872894755),
(1.,0.818555146164949,1.00013293409486),(1.,0.832856393646837,1.00012245640233),
(1.,0.85330159413291,1.00010747739266),(1.,0.859973357550731,1.00010258937951),
(1.,0.872649703192779,1.00009330215809),(1.,0.878678246012902,1.00008888539527),
(1.,0.895698741577251,1.00007641546778),(1.,0.905642962900618,1.00006912991499),
(1.,0.917746072269094,1.00006026267045),(1.,0.921298090426927,1.00005766031327),
(1.,0.927803451698529,1.0000528942133),(1.,0.930472809117578,1.00005093853032),
(1.,0.93212849615166,1.00004972550469)))
REPRESENTATION_ITEM('')
SURFACE()
);
#1668=(
BOUNDED_SURFACE()
B_SPLINE_SURFACE(3,2,((#102253,#102254,#102255),(#102256,#102257,#102258),
(#102259,#102260,#102261),(#102262,#102263,#102264),(#102265,#102266,#102267),
(#102268,#102269,#102270),(#102271,#102272,#102273),(#102274,#102275,#102276),
(#102277,#102278,#102279),(#102280,#102281,#102282),(#102283,#102284,#102285),
(#102286,#102287,#102288),(#102289,#102290,#102291),(#102292,#102293,#102294),
(#102295,#102296,#102297),(#102298,#102299,#102300),(#102301,#102302,#102303),
(#102304,#102305,#102306),(#102307,#102308,#102309),(#102310,#102311,#102312),
(#102313,#102314,#102315),(#102316,#102317,#102318),(#102319,#102320,#102321),
(#102322,#102323,#102324),(#102325,#102326,#102327),(#102328,#102329,#102330),
(#102331,#102332,#102333),(#102334,#102335,#102336),(#102337,#102338,#102339),
(#102340,#102341,#102342),(#102343,#102344,#102345),(#102346,#102347,#102348),
(#102349,#102350,#102351),(#102352,#102353,#102354),(#102355,#102356,#102357),
(#102358,#102359,#102360),(#102361,#102362,#102363),(#102364,#102365,#102366),
(#102367,#102368,#102369),(#102370,#102371,#102372),(#102373,#102374,#102375),
(#102376,#102377,#102378),(#102379,#102380,#102381),(#102382,#102383,#102384),
(#102385,#102386,#102387),(#102388,#102389,#102390),(#102391,#102392,#102393),
(#102394,#102395,#102396),(#102397,#102398,#102399),(#102400,#102401,#102402)),
 .UNSPECIFIED.,.F.,.F.,.F.)
B_SPLINE_SURFACE_WITH_KNOTS((4,2,2,2,2,2,2,2,2,2,2,2,2,2,2,2,2,2,2,2,2,
2,2,2,4),(3,3),(0.,0.0025187116162184,0.00377806742432761,0.00503742323243681,
0.00629677904054601,0.00755613484865521,0.0100748464648736,0.0113342022729828,
0.012593558081092,0.0151122696973104,0.0163716255054196,0.0176309813135288,
0.018890337121638,0.0201496929297472,0.0226684045459656,0.0239277603540748,
0.025187116162184,0.0264464719702932,0.0277058277784024,0.0302245393946208,
0.0327432510108392,0.0352619626270576,0.0365213184351669,0.0377806742432761,
0.0402993858594945),(0.,1.),.UNSPECIFIED.)
GEOMETRIC_REPRESENTATION_ITEM()
RATIONAL_B_SPLINE_SURFACE(((1.,0.444837807664136,1.),(1.,0.443889729175589,
1.),(1.,0.447748071183855,1.),(1.,0.459453142902776,1.),(1.,0.464367346379585,
1.),(1.,0.475717163519536,1.),(1.,0.48211295799902,1.),(1.,0.495944712524718,
1.),(1.,0.503380981743553,1.),(1.,0.518962657925113,1.),(1.,0.527139185789211,
1.),(1.,0.551895636149689,1.),(1.,0.568781778812327,1.),(1.,0.593444445481799,
1.),(1.,0.601597343431266,1.),(1.,0.61732836948322,1.),(1.,0.624889681210996,
1.),(1.,0.646485984307859,1.),(1.,0.659441840352202,1.),(1.,0.675982223306384,
1.),(1.,0.68102172685123,1.),(1.,0.689763664719054,1.),(1.,0.693504359158594,
1.),(1.,0.69968025928586,1.),(1.,0.702115682658639,1.),(1.,0.705612781075522,
1.),(1.,0.706675637348199,1.),(1.,0.707648224727786,1.),(1.,0.705356532405246,
1.),(1.,0.697802511437167,1.),(1.,0.69458157237586,1.),(1.,0.686829651284654,
1.),(1.,0.682347030399091,1.),(1.,0.672289714801745,1.),(1.,0.666714572428337,
1.),(1.,0.654569105179005,1.),(1.,0.647967838573232,1.),(1.,0.627025457575446,
1.),(1.,0.611679454062546,1.),(1.,0.579351199094756,1.),(1.,0.56222647842645,
1.),(1.,0.529022354961919,1.),(1.,0.512804015742491,1.),(1.,0.490778638607675,
1.),(1.,0.48379298434534,1.),(1.,0.471266214350623,1.),(1.,0.46570913806108,
1.),(1.,0.451670624760032,1.),(1.,0.445830006853561,1.),(1.,0.444857616465186,
1.)))
REPRESENTATION_ITEM('')
SURFACE()
);
#1669=(
BOUNDED_SURFACE()
B_SPLINE_SURFACE(3,2,((#103225,#103226,#103227),(#103228,#103229,#103230),
(#103231,#103232,#103233),(#103234,#103235,#103236),(#103237,#103238,#103239),
(#103240,#103241,#103242),(#103243,#103244,#103245),(#103246,#103247,#103248),
(#103249,#103250,#103251),(#103252,#103253,#103254),(#103255,#103256,#103257),
(#103258,#103259,#103260),(#103261,#103262,#103263),(#103264,#103265,#103266),
(#103267,#103268,#103269),(#103270,#103271,#103272),(#103273,#103274,#103275),
(#103276,#103277,#103278)),.UNSPECIFIED.,.F.,.F.,.F.)
B_SPLINE_SURFACE_WITH_KNOTS((4,2,2,2,2,2,2,2,4),(3,3),(0.,0.392699081698724,
0.785398163397448,1.17809724509617,1.5707963267949,1.96349540849362,2.35619449019234,
2.74889357189107,3.14159265358979),(0.,1.),.UNSPECIFIED.)
GEOMETRIC_REPRESENTATION_ITEM()
RATIONAL_B_SPLINE_SURFACE(((1.,0.766044443118988,1.),(1.,0.766049891332403,
1.),(1.,0.764573371724783,1.),(1.,0.758863530286151,1.),(1.,0.754625142483316,
1.),(1.,0.74389933443991,1.),(1.,0.737413012003865,1.),(1.,0.723033687231336,
1.),(1.,0.715143224098042,1.),(1.,0.699070338275054,1.),(1.,0.690892921248369,
1.),(1.,0.675524086364245,1.),(1.,0.668340746363067,1.),(1.,0.656206116553444,
1.),(1.,0.651264584058791,1.),(1.,0.644551763110563,1.),(1.,0.642777121345109,
1.),(1.,0.642787609686527,1.)))
REPRESENTATION_ITEM('')
SURFACE()
);
#1670=(
BOUNDED_SURFACE()
B_SPLINE_SURFACE(3,2,((#103526,#103527,#103528),(#103529,#103530,#103531),
(#103532,#103533,#103534),(#103535,#103536,#103537),(#103538,#103539,#103540),
(#103541,#103542,#103543),(#103544,#103545,#103546),(#103547,#103548,#103549),
(#103550,#103551,#103552),(#103553,#103554,#103555),(#103556,#103557,#103558),
(#103559,#103560,#103561),(#103562,#103563,#103564),(#103565,#103566,#103567),
(#103568,#103569,#103570),(#103571,#103572,#103573),(#103574,#103575,#103576),
(#103577,#103578,#103579)),.UNSPECIFIED.,.F.,.F.,.F.)
B_SPLINE_SURFACE_WITH_KNOTS((4,2,2,2,2,2,2,2,4),(3,3),(3.14159265358979,
3.53429173528852,3.92699081698724,4.31968989868597,4.71238898038469,5.10508806208341,
5.49778714378214,5.89048622548086,6.28318530717959),(0.,1.),
 .UNSPECIFIED.)
GEOMETRIC_REPRESENTATION_ITEM()
RATIONAL_B_SPLINE_SURFACE(((1.,0.642787609686527,1.),(1.,0.642777121345374,
1.),(1.,0.64455176311021,1.),(1.,0.651264584059143,1.),(1.,0.656206116553373,
1.),(1.,0.668340746363138,1.),(1.,0.675524086364297,1.),(1.,0.690892921248316,
1.),(1.,0.699070338275045,1.),(1.,0.71514322409805,1.),(1.,0.723033687231423,
1.),(1.,0.737413012003777,1.),(1.,0.74389933443967,1.),(1.,0.754625142483555,
1.),(1.,0.758863530286359,1.),(1.,0.764573371724574,1.),(1.,0.76604989133256,
1.),(1.,0.766044443118988,1.)))
REPRESENTATION_ITEM('')
SURFACE()
);
#1671=(
BOUNDED_SURFACE()
B_SPLINE_SURFACE(3,2,((#104053,#104054,#104055),(#104056,#104057,#104058),
(#104059,#104060,#104061),(#104062,#104063,#104064),(#104065,#104066,#104067),
(#104068,#104069,#104070),(#104071,#104072,#104073),(#104074,#104075,#104076),
(#104077,#104078,#104079),(#104080,#104081,#104082),(#104083,#104084,#104085),
(#104086,#104087,#104088),(#104089,#104090,#104091),(#104092,#104093,#104094),
(#104095,#104096,#104097),(#104098,#104099,#104100),(#104101,#104102,#104103),
(#104104,#104105,#104106),(#104107,#104108,#104109),(#104110,#104111,#104112),
(#104113,#104114,#104115),(#104116,#104117,#104118),(#104119,#104120,#104121),
(#104122,#104123,#104124),(#104125,#104126,#104127),(#104128,#104129,#104130),
(#104131,#104132,#104133),(#104134,#104135,#104136),(#104137,#104138,#104139),
(#104140,#104141,#104142),(#104143,#104144,#104145),(#104146,#104147,#104148),
(#104149,#104150,#104151),(#104152,#104153,#104154),(#104155,#104156,#104157),
(#104158,#104159,#104160),(#104161,#104162,#104163),(#104164,#104165,#104166),
(#104167,#104168,#104169),(#104170,#104171,#104172),(#104173,#104174,#104175),
(#104176,#104177,#104178),(#104179,#104180,#104181),(#104182,#104183,#104184),
(#104185,#104186,#104187),(#104188,#104189,#104190),(#104191,#104192,#104193),
(#104194,#104195,#104196),(#104197,#104198,#104199),(#104200,#104201,#104202)),
 .UNSPECIFIED.,.F.,.F.,.F.)
B_SPLINE_SURFACE_WITH_KNOTS((4,2,2,2,2,2,2,2,2,2,2,2,2,2,2,2,2,2,2,2,2,
2,2,2,4),(3,3),(0.0401498964591801,0.0428180974757128,0.044077453283822,
0.0453368090919312,0.0478555207081496,0.0503742323243681,0.0516335881324773,
0.0528929439405865,0.0554116555568049,0.0566710113649141,0.0579303671730233,
0.0604490787892417,0.0617084345973509,0.0629677904054601,0.0642271462135693,
0.0654865020216785,0.0680052136378969,0.0692645694460061,0.0705239252541153,
0.0717832810622245,0.0730426368703337,0.0755613484865521,0.0768207042946613,
0.0780800601027705,0.0807482611193032),(-0.000149489400314319,1.00005043309073),
 .UNSPECIFIED.)
GEOMETRIC_REPRESENTATION_ITEM()
RATIONAL_B_SPLINE_SURFACE(((1.00016593113143,0.444979039486126,1.00005597447691),
(1.00016643634691,0.443289150557816,1.00005614490407),(1.00016529660589,
0.447101455982151,1.00005576042886),(1.00016168673046,0.459176083043693,
1.00005454268938),(1.00016023845558,0.464020399532478,1.00005405413471),
(1.0001568480558,0.475360905223927,1.00005291043219),(1.00015492735237,
0.481785442045407,1.00005226251055),(1.00014872412617,0.502534535585041,
1.00005016994155),(1.00014399003011,0.518369554110557,1.00004857296244),
(1.00013406108711,0.551580751016643,1.00004522357655),(1.00012899351324,
0.568531215324515,1.00004351410351),(1.00012163222129,0.593153908442809,
1.00004103087771),(1.00011921529229,0.601238263928208,1.00004021556153),
(1.00011450349337,0.616998701048742,1.00003862610404),(1.00011220865661,
0.624674671757922,1.00003785197391),(1.00010570995292,0.646412104231448,
1.00003565972984),(1.00010183928869,0.659359040447713,1.00003435401702),
(1.00009691980327,0.675814165548792,1.00003269449948),(1.00009542797567,
0.680804160975152,1.00003219125293),(1.0000927816452,0.689655838565047,
1.00003129855147),(1.00009164983775,0.693441607130467,1.00003091675252),
(1.0000888664481,0.702751732254162,1.00002997781612),(1.00008780970836,
0.706286407750837,1.00002962134019),(1.000087517189,0.707264852088577,1.000029522663),
(1.00008764050632,0.706852369539625,1.00002956426232),(1.00008831781664,
0.704586842745149,1.0000297927432),(1.00008886935843,0.702741997522547,
1.00002997879788),(1.00009037928611,0.697691459383048,1.00003048815023),
(1.00009133772998,0.694485572475585,1.00003081146747),(1.00009365026412,
0.686750406029988,1.00003159156755),(1.00009500848198,0.682207320168808,
1.00003204974277),(1.00009954618833,0.667029203085519,1.00003358047265),
(1.0001032112903,0.654769849490324,1.000034816842),(1.00010947933538,0.633803944091153,
1.00003693127671),(1.00011169564763,0.626390629056982,1.00003767891772),
(1.0001162633142,0.61111229843889,1.00003921975424),(1.00011862464285,0.603213919841106,
1.00004001631445),(1.00012345746406,0.587048676802423,1.00004164659706),
(1.00012592916457,0.578781116742047,1.00004248038963),(1.00013093264633,
0.562045033359206,1.00004416824212),(1.00013347588336,0.553538191714369,
1.0000450261665),(1.00014096760153,0.528479237548492,1.0000475533897),(1.00014581500858,
0.512265206506655,1.00004918859264),(1.00015235765643,0.490380785760463,
1.00005139566065),(1.00015441501403,0.483499156141063,1.0000520896806),
(1.00015816391477,0.470959505082299,1.00005335431825),(1.00015984343524,
0.465341698114523,1.00005392088029),(1.00016419732593,0.450778423751254,
1.0000553896026),(1.00016593013437,0.44498237454662,1.00005597414056),(1.00016604025919,
0.444614019388471,1.00005601128959)))
REPRESENTATION_ITEM('')
SURFACE()
);
#1672=(
BOUNDED_SURFACE()
B_SPLINE_SURFACE(3,2,((#104203,#104204,#104205),(#104206,#104207,#104208),
(#104209,#104210,#104211),(#104212,#104213,#104214),(#104215,#104216,#104217),
(#104218,#104219,#104220),(#104221,#104222,#104223),(#104224,#104225,#104226),
(#104227,#104228,#104229),(#104230,#104231,#104232),(#104233,#104234,#104235),
(#104236,#104237,#104238),(#104239,#104240,#104241),(#104242,#104243,#104244),
(#104245,#104246,#104247),(#104248,#104249,#104250),(#104251,#104252,#104253),
(#104254,#104255,#104256),(#104257,#104258,#104259),(#104260,#104261,#104262),
(#104263,#104264,#104265),(#104266,#104267,#104268),(#104269,#104270,#104271),
(#104272,#104273,#104274),(#104275,#104276,#104277),(#104278,#104279,#104280),
(#104281,#104282,#104283),(#104284,#104285,#104286),(#104287,#104288,#104289),
(#104290,#104291,#104292),(#104293,#104294,#104295),(#104296,#104297,#104298),
(#104299,#104300,#104301),(#104302,#104303,#104304),(#104305,#104306,#104307),
(#104308,#104309,#104310),(#104311,#104312,#104313),(#104314,#104315,#104316),
(#104317,#104318,#104319),(#104320,#104321,#104322),(#104323,#104324,#104325),
(#104326,#104327,#104328),(#104329,#104330,#104331),(#104332,#104333,#104334),
(#104335,#104336,#104337),(#104338,#104339,#104340),(#104341,#104342,#104343),
(#104344,#104345,#104346),(#104347,#104348,#104349),(#104350,#104351,#104352),
(#104353,#104354,#104355),(#104356,#104357,#104358),(#104359,#104360,#104361),
(#104362,#104363,#104364),(#104365,#104366,#104367),(#104368,#104369,#104370),
(#104371,#104372,#104373),(#104374,#104375,#104376)),.UNSPECIFIED.,.F.,
 .F.,.F.)
B_SPLINE_SURFACE_WITH_KNOTS((4,2,2,2,2,2,2,2,2,2,2,2,2,2,2,2,2,2,2,2,2,
2,2,2,2,2,2,2,4),(3,3),(0.0492257416356437,0.05212126862205,0.0537007010045366,
0.0568595657695099,0.0576492819607532,0.0584389981519965,0.0600184305344832,
0.0615978629169698,0.0631772952994565,0.0663361600644298,0.0679155924469164,
0.0694950248294031,0.0726538895943764,0.0734436057856197,0.074233321976863,
0.0758127543593496,0.0773921867418363,0.0781819029330796,0.0789716191243229,
0.0821304838892962,0.0852893486542695,0.0868687810367562,0.0884482134192428,
0.0900276458017295,0.0916070781842161,0.0947659429491894,0.096345375331676,
0.0979248077141627,0.102399767083081),(-0.00131609460394527,1.),
 .UNSPECIFIED.)
GEOMETRIC_REPRESENTATION_ITEM()
RATIONAL_B_SPLINE_SURFACE(((1.00019594420023,0.925558466828159,1.),(1.00018290788058,
0.930511119781782,1.),(1.0001751814063,0.933446499297356,1.),(1.00017321277706,
0.934194404970496,1.),(1.0001744476356,0.933725267517896,1.),(1.00018352032596,
0.930278444495986,1.),(1.00019661401617,0.925303995782883,1.),(1.00022056253643,
0.916205667977813,1.),(1.00022574524419,0.914236695630683,1.),(1.00023669726237,
0.910075893610628,1.),(1.00024248153479,0.907878379693053,1.),(1.00026068949453,
0.90096095913229,1.),(1.00027396619521,0.89591698256937,1.),(1.00030249814301,
0.885077356102603,1.),(1.00031775500613,0.879281092265426,1.),(1.0003500033902,
0.867029547437474,1.),(1.00036707393448,0.860544244548642,1.),(1.00041973886326,
0.840536211453396,1.),(1.00045688450781,0.826424139102216,1.),(1.00051343672853,
0.804939277545135,1.),(1.00053242174643,0.797726643344391,1.),(1.00057017087807,
0.783385299064109,1.),(1.00058872431045,0.776336629339777,1.),(1.00064219262702,
0.756023379667273,1.),(1.00067513352966,0.743508738794324,1.),(1.00070920004036,
0.730566466029059,1.),(1.00071565293189,0.728114935756786,1.),(1.00072756192772,
0.723590566538064,1.),(1.0007330434182,0.721508083078691,1.),(1.00074797494598,
0.715835418009637,1.),(1.00075591036059,0.712820659575825,1.),(1.000767275578,
0.708502878251978,1.),(1.00077070476305,0.707200090045197,1.),(1.00077216358358,
0.706645866767436,1.),(1.00077203127614,0.706696131940276,1.),(1.00077052239234,
0.707269374848357,1.),(1.00076915238989,0.707789855080943,1.),(1.00075935410316,
0.711512340799273,1.),(1.00074204927767,0.718086649909378,1.),(1.00069241079651,
0.736944899541594,1.),(1.00066105961441,0.748855586662284,1.),(1.00060901661395,
0.768627341787248,1.),(1.00059072235101,0.77557754995927,1.),(1.00055350269926,
0.789717738526475,1.),(1.00053461513014,0.796893350775199,1.),(1.00049682155246,
0.81125158063532,1.),(1.00047791391785,0.818434816002099,1.),(1.00044051452833,
0.832643289086462,1.),(1.00042195785068,0.839693191730224,1.),(1.0003679404696,
0.860215037543297,1.),(1.00033443596869,0.87294379610312,1.),(1.00028952640061,
0.890005475388769,1.),(1.00027544616487,0.895354724483665,1.),(1.00024937271555,
0.905260338122725,1.),(1.00023733657422,0.909833011429418,1.),(1.00019681928589,
0.925226011375529,1.),(1.00017807148057,0.932348525694257,1.),(1.00017411585802,
0.93385131376765,1.)))
REPRESENTATION_ITEM('')
SURFACE()
);
#1673=(
BOUNDED_SURFACE()
B_SPLINE_SURFACE(3,2,((#104377,#104378,#104379),(#104380,#104381,#104382),
(#104383,#104384,#104385),(#104386,#104387,#104388),(#104389,#104390,#104391),
(#104392,#104393,#104394),(#104395,#104396,#104397),(#104398,#104399,#104400),
(#104401,#104402,#104403),(#104404,#104405,#104406),(#104407,#104408,#104409),
(#104410,#104411,#104412),(#104413,#104414,#104415),(#104416,#104417,#104418),
(#104419,#104420,#104421),(#104422,#104423,#104424),(#104425,#104426,#104427),
(#104428,#104429,#104430),(#104431,#104432,#104433),(#104434,#104435,#104436),
(#104437,#104438,#104439),(#104440,#104441,#104442),(#104443,#104444,#104445),
(#104446,#104447,#104448),(#104449,#104450,#104451),(#104452,#104453,#104454),
(#104455,#104456,#104457),(#104458,#104459,#104460),(#104461,#104462,#104463),
(#104464,#104465,#104466),(#104467,#104468,#104469),(#104470,#104471,#104472),
(#104473,#104474,#104475),(#104476,#104477,#104478),(#104479,#104480,#104481),
(#104482,#104483,#104484),(#104485,#104486,#104487),(#104488,#104489,#104490),
(#104491,#104492,#104493),(#104494,#104495,#104496),(#104497,#104498,#104499),
(#104500,#104501,#104502),(#104503,#104504,#104505),(#104506,#104507,#104508),
(#104509,#104510,#104511),(#104512,#104513,#104514),(#104515,#104516,#104517),
(#104518,#104519,#104520),(#104521,#104522,#104523),(#104524,#104525,#104526),
(#104527,#104528,#104529),(#104530,#104531,#104532),(#104533,#104534,#104535),
(#104536,#104537,#104538),(#104539,#104540,#104541),(#104542,#104543,#104544)),
 .UNSPECIFIED.,.F.,.F.,.F.)
B_SPLINE_SURFACE_WITH_KNOTS((4,2,2,2,2,2,2,2,2,2,2,2,2,2,2,2,2,2,2,2,2,
2,2,2,2,2,2,4),(3,3),(0.0511475161399861,0.0543755745194946,0.0559748561230095,
0.0575741377265244,0.0591734193300392,0.0607727009335541,0.062371982537069,
0.0639712641405839,0.0671698273476136,0.0687691089511285,0.0703683905546434,
0.0735669537616731,0.0743665945634306,0.075166235365188,0.0767655169687029,
0.0783647985722178,0.0799640801757326,0.0831626433827624,0.0839622841845198,
0.0847619249862773,0.0863612065897922,0.087960488193307,0.0895597697968219,
0.0911590514003368,0.0927583330038517,0.0959568962108814,0.0991554594179112,
0.102525861223953),(0.,1.00017183859901),.UNSPECIFIED.)
GEOMETRIC_REPRESENTATION_ITEM()
RATIONAL_B_SPLINE_SURFACE(((0.999999999999999,0.363791624139497,1.00021865031197),
(1.,0.345907098152807,1.00022479681575),(1.,0.333093359896291,1.00022920060541),
(1.,0.326997783970327,1.00023129551587),(1.,0.327177805749954,1.00023123364649),
(1.,0.331655133124558,1.00022969489116),(1.,0.33594526264938,1.00022822047147),
(1.,0.347973250814003,1.0002240867262),(1.,0.355767139651311,1.00022140814432),
(1.,0.373420234385515,1.00021534117819),(1.,0.383300909504948,1.00021194541545),
(1.,0.404353607436141,1.00020471008321),(1.,0.415539518961281,1.00020086574048),
(1.,0.438608462395935,1.00019293747064),(1.,0.450347915466347,1.0001889028883),
(1.,0.48562633119133,1.00017677850123),(1.,0.509203616458581,1.0001686755259),
(1.,0.543403436110305,1.00015692182771),(1.,0.554652013302503,1.00015305594821),
(1.,0.576466905683596,1.00014555866713),(1.,0.58694153284502,1.00014195877661),
(1.,0.616911695858428,1.00013165871496),(1.,0.634969557244847,1.00012545263976),
(1.,0.654503005935658,1.00011873943885),(1.,0.65825654007911,1.00011744943475),
(1.,0.665435063621704,1.00011498233989),(1.,0.668871309120368,1.00011380138067),
(1.,0.678546034793369,1.00011047639806),(1.,0.684157382338495,1.00010854790585),
(1.,0.693634268435882,1.00010529091619),(1.,0.697500232426135,1.00010396227252),
(1.,0.703370534929454,1.00010194478341),(1.,0.705371444929301,1.00010125711626),
(1.,0.708290812429381,1.00010025379622),(1.,0.706260755280861,1.00010095148057),
(1.,0.69882470043928,1.00010350708307),(1.,0.697084750890873,1.00010410506405),
(1.,0.693165330790786,1.00010545207937),(1.,0.690982356485942,1.00010620231786),
(1.,0.68379338348011,1.00010867300396),(1.,0.678148780393404,1.00011061292534),
(1.,0.665272843129722,1.00011503809138),(1.,0.658004130630274,1.00011753618212),
(1.,0.642133827810631,1.00012299044333),(1.,0.6335794985508,1.00012593037124),
(1.,0.615382081200458,1.00013218440864),(1.,0.605738300581893,1.00013549875614),
(1.,0.585480053220422,1.00014246105383),(1.,0.57481870187419,1.00014612511719),
(1.,0.54200218601379,1.00015740340541),(1.,0.51896068005778,1.00016532224562),
(1.,0.471865311436787,1.00018150784994),(1.,0.447600125261933,1.00018984724114),
(1.,0.400739305781053,1.00020595223628),(1.,0.378121326325834,1.00021372552008),
(1.,0.360032870100529,1.00021994211003)))
REPRESENTATION_ITEM('')
SURFACE()
);
#1674=(
BOUNDED_SURFACE()
B_SPLINE_SURFACE(3,2,((#104546,#104547,#104548),(#104549,#104550,#104551),
(#104552,#104553,#104554),(#104555,#104556,#104557),(#104558,#104559,#104560),
(#104561,#104562,#104563),(#104564,#104565,#104566),(#104567,#104568,#104569),
(#104570,#104571,#104572),(#104573,#104574,#104575),(#104576,#104577,#104578),
(#104579,#104580,#104581),(#104582,#104583,#104584),(#104585,#104586,#104587),
(#104588,#104589,#104590),(#104591,#104592,#104593),(#104594,#104595,#104596),
(#104597,#104598,#104599),(#104600,#104601,#104602),(#104603,#104604,#104605),
(#104606,#104607,#104608),(#104609,#104610,#104611),(#104612,#104613,#104614),
(#104615,#104616,#104617),(#104618,#104619,#104620),(#104621,#104622,#104623),
(#104624,#104625,#104626),(#104627,#104628,#104629),(#104630,#104631,#104632),
(#104633,#104634,#104635),(#104636,#104637,#104638),(#104639,#104640,#104641),
(#104642,#104643,#104644),(#104645,#104646,#104647),(#104648,#104649,#104650),
(#104651,#104652,#104653),(#104654,#104655,#104656),(#104657,#104658,#104659),
(#104660,#104661,#104662),(#104663,#104664,#104665),(#104666,#104667,#104668),
(#104669,#104670,#104671),(#104672,#104673,#104674),(#104675,#104676,#104677),
(#104678,#104679,#104680),(#104681,#104682,#104683),(#104684,#104685,#104686),
(#104687,#104688,#104689),(#104690,#104691,#104692),(#104693,#104694,#104695)),
 .UNSPECIFIED.,.F.,.F.,.F.)
B_SPLINE_SURFACE_WITH_KNOTS((4,2,2,2,2,2,2,2,2,2,2,2,2,2,2,2,2,2,2,2,2,
2,2,2,4),(3,3),(0.0411832956025613,0.0424965399968198,0.0437843139361192,
0.0463598618147179,0.0476476357540172,0.0489354096933166,0.0515109575719153,
0.054086505450514,0.0553742793898133,0.0566620533291127,0.0592376012077114,
0.0618131490863101,0.0631009230256095,0.0643886969649088,0.0656764709042082,
0.0669642448435075,0.0695397927221063,0.0708275666614056,0.072115340600705,
0.0734031145400043,0.0746908884793037,0.0772664363579024,0.0785542102972017,
0.0798419842365011,0.0824175321150998),(-2.54704549892859E-5,1.),
 .UNSPECIFIED.)
GEOMETRIC_REPRESENTATION_ITEM()
RATIONAL_B_SPLINE_SURFACE(((1.00002969011113,0.41716567016007,1.),(1.00002994384796,
0.412184667121395,1.),(1.0000301347314,0.408437513003748,1.),(1.00003036746518,
0.403868812055419,1.),(1.00003041084928,0.403017156769614,1.),(1.00003031596223,
0.404879845196922,1.),(1.00002995641597,0.411937949549854,1.),(1.00002907725759,
0.42919634528864,1.),(1.0000287281148,0.436050223421914,1.),(1.0000279625118,
0.45107946022051,1.),(1.00002754420566,0.459291055676708,1.),(1.00002621873246,
0.485310873574663,1.),(1.00002523535442,0.504615162293121,1.),(1.00002327853494,
0.543028678709834,1.),(1.00002229863343,0.562264721202267,1.),(1.00002088610616,
0.58999346174123,1.),(1.00002042575008,0.599030522075286,1.),(1.00001954857755,
0.616249934281681,1.),(1.00001912948864,0.624476895847254,1.),(1.00001793948785,
0.647837310828753,1.),(1.0000172350414,0.661666008506602,1.),(1.00001606044591,
0.68472400830539,1.),(1.00001561170694,0.693533018117966,1.),(1.00001517175011,
0.702169629233436,1.),(1.00001506362195,0.704292248448626,1.),(1.00001493152404,
0.706885408022375,1.),(1.0000149083449,0.70734042817065,1.),(1.00001494501072,
0.706620656543938,1.),(1.00001500486264,0.705445728351282,1.),(1.00001520669394,
0.701483661229885,1.),(1.00001534974885,0.698675409330837,1.),(1.00001589553929,
0.687961222177015,1.),(1.0000164072945,0.677915166725478,1.),(1.00001736385409,
0.659137339788157,1.),(1.00001771630397,0.652218541517549,1.),(1.00001846671731,
0.637487486635047,1.),(1.00001886535688,0.629661957539986,1.),(1.00001970257416,
0.613226890341952,1.),(1.0000201411837,0.604616727276649,1.),(1.00002105184036,
0.586740001976879,1.),(1.00002152598384,0.577432286849769,1.),(1.00002296522561,
0.549179124901904,1.),(1.00002395181897,0.529811717588144,1.),(1.00002540634078,
0.501258599676148,1.),(1.00002588670869,0.491828695166698,1.),(1.00002682175625,
0.473473162191487,1.),(1.000027272038,0.464633866720484,1.),(1.0000285273913,
0.439990543645249,1.),(1.00002924391365,0.425924788916652,1.),(1.00002973290203,
0.416325659622527,1.)))
REPRESENTATION_ITEM('')
SURFACE()
);
#1675=(
BOUNDED_SURFACE()
B_SPLINE_SURFACE(3,2,((#104696,#104697,#104698),(#104699,#104700,#104701),
(#104702,#104703,#104704),(#104705,#104706,#104707),(#104708,#104709,#104710),
(#104711,#104712,#104713),(#104714,#104715,#104716),(#104717,#104718,#104719),
(#104720,#104721,#104722),(#104723,#104724,#104725),(#104726,#104727,#104728),
(#104729,#104730,#104731),(#104732,#104733,#104734),(#104735,#104736,#104737),
(#104738,#104739,#104740),(#104741,#104742,#104743),(#104744,#104745,#104746),
(#104747,#104748,#104749),(#104750,#104751,#104752),(#104753,#104754,#104755),
(#104756,#104757,#104758),(#104759,#104760,#104761),(#104762,#104763,#104764),
(#104765,#104766,#104767),(#104768,#104769,#104770),(#104771,#104772,#104773),
(#104774,#104775,#104776),(#104777,#104778,#104779),(#104780,#104781,#104782),
(#104783,#104784,#104785),(#104786,#104787,#104788),(#104789,#104790,#104791),
(#104792,#104793,#104794),(#104795,#104796,#104797),(#104798,#104799,#104800),
(#104801,#104802,#104803),(#104804,#104805,#104806),(#104807,#104808,#104809),
(#104810,#104811,#104812),(#104813,#104814,#104815),(#104816,#104817,#104818),
(#104819,#104820,#104821),(#104822,#104823,#104824),(#104825,#104826,#104827),
(#104828,#104829,#104830),(#104831,#104832,#104833),(#104834,#104835,#104836),
(#104837,#104838,#104839),(#104840,#104841,#104842),(#104843,#104844,#104845)),
 .UNSPECIFIED.,.F.,.F.,.F.)
B_SPLINE_SURFACE_WITH_KNOTS((4,2,2,2,2,2,2,2,2,2,2,2,2,2,2,2,2,2,2,2,2,
2,2,2,4),(3,3),(0.0411832956025262,0.0424965399968198,0.0437843139361192,
0.0463598618147179,0.0476476357540172,0.0489354096933166,0.0515109575719153,
0.054086505450514,0.0553742793898133,0.0566620533291127,0.0592376012077114,
0.0618131490863101,0.0631009230256095,0.0643886969649088,0.0656764709042082,
0.0669642448435075,0.0695397927221063,0.0708275666614056,0.072115340600705,
0.0734031145400043,0.0746908884793037,0.0772664363579024,0.0785542102972017,
0.0798419842365011,0.0824175321150998),(-2.54704550244023E-5,1.),
 .UNSPECIFIED.)
GEOMETRIC_REPRESENTATION_ITEM()
RATIONAL_B_SPLINE_SURFACE(((1.00002969011117,0.417165670160449,1.),(1.000029943848,
0.412184667121575,1.),(1.00003013473144,0.408437513003789,1.),(1.00003036746522,
0.403868812055398,1.),(1.00003041084932,0.403017156769593,1.),(1.00003031596227,
0.404879845196902,1.),(1.00002995641602,0.411937949549833,1.),(1.00002907725763,
0.42919634528862,1.),(1.00002872811484,0.436050223421894,1.),(1.00002796251184,
0.451079460220491,1.),(1.0000275442057,0.459291055676689,1.),(1.00002621873249,
0.485310873574645,1.),(1.00002523535446,0.504615162293104,1.),(1.00002327853497,
0.543028678709818,1.),(1.00002229863346,0.562264721202251,1.),(1.00002088610619,
0.589993461741216,1.),(1.00002042575011,0.599030522075271,1.),(1.00001954857758,
0.616249934281668,1.),(1.00001912948867,0.624476895847241,1.),(1.00001793948787,
0.64783731082874,1.),(1.00001723504143,0.66166600850659,1.),(1.00001606044593,
0.684724008305379,1.),(1.00001561170696,0.693533018117955,1.),(1.00001517175013,
0.702169629233425,1.),(1.00001506362197,0.704292248448615,1.),(1.00001493152406,
0.706885408022364,1.),(1.00001490834492,0.70734042817064,1.),(1.00001494501075,
0.706620656543927,1.),(1.00001500486266,0.705445728351272,1.),(1.00001520669396,
0.701483661229874,1.),(1.00001534974887,0.698675409330827,1.),(1.00001589553931,
0.687961222177005,1.),(1.00001640729452,0.677915166725467,1.),(1.00001736385411,
0.659137339788145,1.),(1.00001771630399,0.652218541517537,1.),(1.00001846671733,
0.637487486635034,1.),(1.00001886535691,0.629661957539973,1.),(1.00001970257419,
0.613226890341938,1.),(1.00002014118373,0.604616727276635,1.),(1.00002105184039,
0.586740001976865,1.),(1.00002152598387,0.577432286849754,1.),(1.00002296522565,
0.549179124901888,1.),(1.000023951819,0.529811717588127,1.),(1.00002540634081,
0.50125859967613,1.),(1.00002588670873,0.49182869516668,1.),(1.00002682175628,
0.473473162191469,1.),(1.00002727203804,0.464633866720466,1.),(1.00002852739134,
0.439990543645229,1.),(1.00002924391369,0.425924788916632,1.),(1.00002973290207,
0.416325659622506,1.)))
REPRESENTATION_ITEM('')
SURFACE()
);
#1676=(
BOUNDED_SURFACE()
B_SPLINE_SURFACE(3,2,((#105057,#105058,#105059),(#105060,#105061,#105062),
(#105063,#105064,#105065),(#105066,#105067,#105068),(#105069,#105070,#105071),
(#105072,#105073,#105074),(#105075,#105076,#105077),(#105078,#105079,#105080),
(#105081,#105082,#105083),(#105084,#105085,#105086),(#105087,#105088,#105089),
(#105090,#105091,#105092),(#105093,#105094,#105095),(#105096,#105097,#105098),
(#105099,#105100,#105101),(#105102,#105103,#105104),(#105105,#105106,#105107),
(#105108,#105109,#105110),(#105111,#105112,#105113),(#105114,#105115,#105116),
(#105117,#105118,#105119),(#105120,#105121,#105122),(#105123,#105124,#105125),
(#105126,#105127,#105128),(#105129,#105130,#105131),(#105132,#105133,#105134),
(#105135,#105136,#105137),(#105138,#105139,#105140),(#105141,#105142,#105143),
(#105144,#105145,#105146),(#105147,#105148,#105149),(#105150,#105151,#105152),
(#105153,#105154,#105155),(#105156,#105157,#105158),(#105159,#105160,#105161),
(#105162,#105163,#105164),(#105165,#105166,#105167),(#105168,#105169,#105170),
(#105171,#105172,#105173),(#105174,#105175,#105176),(#105177,#105178,#105179),
(#105180,#105181,#105182)),.UNSPECIFIED.,.F.,.F.,.F.)
B_SPLINE_SURFACE_WITH_KNOTS((4,2,2,2,2,2,2,2,2,2,2,2,2,2,2,2,2,2,2,2,4),
(3,3),(0.0200568639003605,0.0213281306129126,0.0225827265313192,0.0232100244905226,
0.0238373224497259,0.0250919183681325,0.0263465142865391,0.0269738122457424,
0.0276011102049457,0.0288557061233524,0.030110302041759,0.0313648979601656,
0.0326194938785723,0.0332467918377756,0.0338740897969789,0.0351286857153855,
0.0363832816337921,0.0376378775521988,0.0382651755114021,0.0388924734706054,
0.040147069389012),(-1.6670794163376E-5,1.),.UNSPECIFIED.)
GEOMETRIC_REPRESENTATION_ITEM()
RATIONAL_B_SPLINE_SURFACE(((1.00001218909147,0.634417792362364,1.),(1.00001207070658,
0.637968459699978,1.),(1.00001198539686,0.640527117559773,1.),(1.00001190087293,
0.643062207776934,1.),(1.00001189940874,0.643106122556049,1.),(1.00001195795143,
0.641350276625085,1.),(1.00001198783686,0.640453935716271,1.),(1.0000120665277,
0.638093795110533,1.),(1.00001211511354,0.636636580788178,1.),(1.00001228558705,
0.631523641684606,1.),(1.0000124323333,0.627122344191632,1.),(1.00001277455001,
0.616858384702073,1.),(1.00001296504766,0.611144870017612,1.),(1.00001325563189,
0.602429501679159,1.),(1.00001335337752,0.599497858598228,1.),(1.00001354628551,
0.593712051753561,1.),(1.0000136417071,0.590850112792402,1.),(1.00001391054031,
0.582787113346938,1.),(1.00001406873562,0.578042429230547,1.),(1.00001430529436,
0.570947423996434,1.),(1.00001438238684,0.568635222351684,1.),(1.00001441730522,
0.56758793028365,1.),(1.00001437708325,0.568794290657144,1.),(1.00001416717897,
0.575089859693509,1.),(1.0000139997862,0.580110399619696,1.),(1.00001367027674,
0.589993235888577,1.),(1.00001354728695,0.593682016041953,1.),(1.00001327743302,
0.601775629678951,1.),(1.0000131303487,0.606187066817002,1.),(1.00001266743157,
0.620071142126849,1.),(1.00001232742341,0.630268861450101,1.),(1.00001161384565,
0.6516708939964,1.),(1.0000112397551,0.662890831923292,1.),(1.00001051322695,
0.684681280272715,1.),(1.0000101570569,0.69536373622251,1.),(1.00000965159222,
0.710523921999963,1.),(1.00000948811148,0.715427130046569,1.),(1.00000918068499,
0.724647641305723,1.),(1.00000903576729,0.728994095987094,1.),(1.00000863062084,
0.741145479997482,1.),(1.00000839984957,0.748066904027392,1.),(1.00000821878182,
0.753497591644584,1.)))
REPRESENTATION_ITEM('')
SURFACE()
);
#1677=(
BOUNDED_SURFACE()
B_SPLINE_SURFACE(3,2,((#105445,#105446,#105447),(#105448,#105449,#105450),
(#105451,#105452,#105453),(#105454,#105455,#105456),(#105457,#105458,#105459),
(#105460,#105461,#105462),(#105463,#105464,#105465),(#105466,#105467,#105468),
(#105469,#105470,#105471),(#105472,#105473,#105474),(#105475,#105476,#105477),
(#105478,#105479,#105480),(#105481,#105482,#105483),(#105484,#105485,#105486),
(#105487,#105488,#105489),(#105490,#105491,#105492),(#105493,#105494,#105495),
(#105496,#105497,#105498),(#105499,#105500,#105501),(#105502,#105503,#105504),
(#105505,#105506,#105507),(#105508,#105509,#105510),(#105511,#105512,#105513),
(#105514,#105515,#105516),(#105517,#105518,#105519),(#105520,#105521,#105522),
(#105523,#105524,#105525),(#105526,#105527,#105528),(#105529,#105530,#105531),
(#105532,#105533,#105534),(#105535,#105536,#105537),(#105538,#105539,#105540),
(#105541,#105542,#105543),(#105544,#105545,#105546),(#105547,#105548,#105549),
(#105550,#105551,#105552),(#105553,#105554,#105555),(#105556,#105557,#105558),
(#105559,#105560,#105561),(#105562,#105563,#105564),(#105565,#105566,#105567),
(#105568,#105569,#105570),(#105571,#105572,#105573),(#105574,#105575,#105576),
(#105577,#105578,#105579),(#105580,#105581,#105582),(#105583,#105584,#105585),
(#105586,#105587,#105588),(#105589,#105590,#105591),(#105592,#105593,#105594)),
 .UNSPECIFIED.,.F.,.F.,.F.)
B_SPLINE_SURFACE_WITH_KNOTS((4,2,2,2,2,2,2,2,2,2,2,2,2,2,2,2,2,2,2,2,2,
2,2,2,4),(3,3),(0.0401498964592781,0.0428180974757128,0.044077453283822,
0.0453368090919312,0.0478555207081496,0.0503742323243681,0.0516335881324773,
0.0528929439405865,0.0554116555568049,0.0566710113649141,0.0579303671730233,
0.0604490787892417,0.0617084345973509,0.0629677904054601,0.0642271462135693,
0.0654865020216785,0.0680052136378969,0.0692645694460061,0.0705239252541153,
0.0717832810622245,0.0730426368703337,0.0755613484865521,0.0768207042946613,
0.0780800601027705,0.0807482611192052),(-5.04330907357126E-5,1.00014948940022),
 .UNSPECIFIED.)
GEOMETRIC_REPRESENTATION_ITEM()
RATIONAL_B_SPLINE_SURFACE(((1.00005597447691,0.444979039485992,1.00016593113132),
(1.00005614490408,0.443289150558148,1.0001664363468),(1.00005576042886,
0.447101455982505,1.00016529660579),(1.00005454268939,0.459176083043744,
1.00016168673036),(1.00005405413472,0.464020399532528,1.00016023845548),
(1.00005291043219,0.475360905223976,1.0001568480557),(1.00005226251056,
0.481785442045456,1.00015492735227),(1.00005016994156,0.502534535585088,
1.00014872412607),(1.00004857296245,0.518369554110602,1.00014399003002),
(1.00004522357656,0.551580751016686,1.00013406108703),(1.00004351410351,
0.568531215324555,1.00012899351315),(1.00004103087771,0.593153908442847,
1.00012163222121),(1.00004021556153,0.601238263928246,1.00011921529221),
(1.00003862610404,0.616998701048778,1.0001145034933),(1.00003785197391,
0.624674671757957,1.00011220865653),(1.00003565972984,0.646412104231481,
1.00010570995285),(1.00003435401702,0.659359040447745,1.00010183928863),
(1.00003269449948,0.675814165548823,1.00009691980321),(1.00003219125293,
0.680804160975182,1.00009542797561),(1.00003129855147,0.689655838565076,
1.00009278164514),(1.00003091675253,0.693441607130496,1.00009164983769),
(1.00002997781612,0.70275173225419,1.00008886644804),(1.0000296213402,0.706286407750865,
1.0000878097083),(1.000029522663,0.707264852088604,1.00008751718895),(1.00002956426232,
0.706852369539653,1.00008764050626),(1.0000297927432,0.704586842745177,
1.00008831781658),(1.00002997879788,0.702741997522575,1.00008886935837),
(1.00003048815023,0.697691459383076,1.00009037928605),(1.00003081146747,
0.694485572475614,1.00009133772992),(1.00003159156755,0.686750406030017,
1.00009365026406),(1.00003204974278,0.682207320168837,1.00009500848191),
(1.00003358047265,0.66702920308555,1.00009954618827),(1.000034816842,0.654769849490357,
1.00010321129023),(1.00003693127672,0.633803944091187,1.00010947933531),
(1.00003767891773,0.626390629057017,1.00011169564756),(1.00003921975424,
0.611112298438927,1.00011626331412),(1.00004001631445,0.603213919841143,
1.00011862464277),(1.00004164659707,0.587048676802461,1.00012345746397),
(1.00004248038963,0.578781116742087,1.00012592916449),(1.00004416824212,
0.562045033359247,1.00013093264624),(1.0000450261665,0.553538191714411,
1.00013347588327),(1.00004755338971,0.528479237548537,1.00014096760144),
(1.00004918859265,0.512265206506701,1.00014581500849),(1.00005139566065,
0.490380785760511,1.00015235765633),(1.0000520896806,0.483499156141111,
1.00015441501393),(1.00005335431826,0.470959505082348,1.00015816391466),
(1.0000539208803,0.465341698114573,1.00015984343514),(1.0000553896026,0.450778423751669,
1.00016419732582),(1.00005597414057,0.444982374547099,1.00016593013426),
(1.00005601128959,0.444614019388563,1.00016604025909)))
REPRESENTATION_ITEM('')
SURFACE()
);
#1678=(
BOUNDED_SURFACE()
B_SPLINE_SURFACE(3,2,((#105595,#105596,#105597),(#105598,#105599,#105600),
(#105601,#105602,#105603),(#105604,#105605,#105606),(#105607,#105608,#105609),
(#105610,#105611,#105612),(#105613,#105614,#105615),(#105616,#105617,#105618),
(#105619,#105620,#105621),(#105622,#105623,#105624),(#105625,#105626,#105627),
(#105628,#105629,#105630),(#105631,#105632,#105633),(#105634,#105635,#105636),
(#105637,#105638,#105639),(#105640,#105641,#105642),(#105643,#105644,#105645),
(#105646,#105647,#105648),(#105649,#105650,#105651),(#105652,#105653,#105654),
(#105655,#105656,#105657),(#105658,#105659,#105660),(#105661,#105662,#105663),
(#105664,#105665,#105666),(#105667,#105668,#105669),(#105670,#105671,#105672),
(#105673,#105674,#105675),(#105676,#105677,#105678),(#105679,#105680,#105681),
(#105682,#105683,#105684),(#105685,#105686,#105687),(#105688,#105689,#105690),
(#105691,#105692,#105693),(#105694,#105695,#105696),(#105697,#105698,#105699),
(#105700,#105701,#105702),(#105703,#105704,#105705),(#105706,#105707,#105708),
(#105709,#105710,#105711),(#105712,#105713,#105714),(#105715,#105716,#105717),
(#105718,#105719,#105720),(#105721,#105722,#105723),(#105724,#105725,#105726),
(#105727,#105728,#105729),(#105730,#105731,#105732),(#105733,#105734,#105735),
(#105736,#105737,#105738),(#105739,#105740,#105741),(#105742,#105743,#105744),
(#105745,#105746,#105747),(#105748,#105749,#105750),(#105751,#105752,#105753),
(#105754,#105755,#105756),(#105757,#105758,#105759),(#105760,#105761,#105762),
(#105763,#105764,#105765),(#105766,#105767,#105768)),.UNSPECIFIED.,.F.,
 .F.,.F.)
B_SPLINE_SURFACE_WITH_KNOTS((4,2,2,2,2,2,2,2,2,2,2,2,2,2,2,2,2,2,2,2,2,
2,2,2,2,2,2,2,4),(3,3),(0.0492257416375651,0.05212126862205,0.0537007010045366,
0.0568595657695099,0.0576492819607532,0.0584389981519965,0.0600184305344832,
0.0615978629169698,0.0631772952994565,0.0663361600644298,0.0679155924469164,
0.0694950248294031,0.0726538895943764,0.0734436057856197,0.074233321976863,
0.0758127543593496,0.0773921867418363,0.0781819029330796,0.0789716191243229,
0.0821304838892962,0.0852893486542695,0.0868687810367562,0.0884482134192428,
0.0900276458017295,0.0916070781842161,0.0947659429491894,0.096345375331676,
0.0979248077141627,0.10239976708116),(0.,1.00131609460202),
 .UNSPECIFIED.)
GEOMETRIC_REPRESENTATION_ITEM()
RATIONAL_B_SPLINE_SURFACE(((1.,0.925558466838161,1.00019594419992),(1.,
0.930511119785811,1.0001829078803),(1.,0.933446499297804,1.00017518140604),
(1.,0.934194404970622,1.0001732127768),(1.,0.933725267518023,1.00017444763534),
(1.,0.93027844449612,1.00018352032569),(1.,0.925303995783027,1.00019661401589),
(1.,0.916205667977974,1.00022056253611),(1.,0.914236695630848,1.00022574524386),
(1.,0.910075893610801,1.00023669726202),(1.,0.907878379693229,1.00024248153443),
(1.,0.90096095913248,1.00026068949415),(1.,0.895916982569569,1.00027396619481),
(1.,0.885077356102823,1.00030249814257),(1.,0.879281092265658,1.00031775500566),
(1.,0.867029547437729,1.00035000338969),(1.,0.86054424454891,1.00036707393394),
(1.,0.840536211453702,1.00041973886265),(1.,0.826424139102549,1.00045688450714),
(1.,0.804939277545509,1.00051343672778),(1.,0.797726643344779,1.00053242174565),
(1.,0.783385299064525,1.00057017087724),(1.,0.776336629340206,1.00058872430959),
(1.,0.756023379667741,1.00064219262608),(1.,0.743508738794816,1.00067513352868),
(1.,0.730566466029576,1.00070920003933),(1.,0.728114935757307,1.00071565293084),
(1.,0.723590566538595,1.00072756192665),(1.,0.721508083079225,1.00073304341713),
(1.,0.715835418010182,1.00074797494489),(1.,0.712820659576376,1.00075591035949),
(1.,0.708502878252537,1.00076727557687),(1.,0.707200090045759,1.00077070476193),
(1.,0.706645866767999,1.00077216358246),(1.,0.706696131940839,1.00077203127501),
(1.,0.707269374848919,1.00077052239122),(1.,0.707789855081503,1.00076915238877),
(1.,0.711512340799826,1.00075935410205),(1.,0.718086649909919,1.00074204927658),
(1.,0.736944899542099,1.0006924107955),(1.,0.748855586662766,1.00066105961344),
(1.,0.768627341787692,1.00060901661306),(1.,0.7755775499597,1.00059072235014),
(1.,0.789717738526879,1.00055350269845),(1.,0.796893350775588,1.00053461512936),
(1.,0.811251580635682,1.00049682155173),(1.,0.818434816002448,1.00047791391715),
(1.,0.832643289086783,1.00044051452769),(1.,0.839693191730531,1.00042195785006),
(1.,0.860215037543565,1.00036794046907),(1.,0.872943796103364,1.0003344359682),
(1.,0.89000547538898,1.00028952640019),(1.,0.895354724483866,1.00027544616447),
(1.,0.905260338122907,1.00024937271519),(1.,0.909833011429591,1.00023733657388),
(1.,0.925226011370787,1.00019681928561),(1.,0.93234852568827,1.00017807148032),
(1.,0.933851313765841,1.00017411585777)))
REPRESENTATION_ITEM('')
SURFACE()
);
#1679=(
BOUNDED_SURFACE()
B_SPLINE_SURFACE(3,2,((#105769,#105770,#105771),(#105772,#105773,#105774),
(#105775,#105776,#105777),(#105778,#105779,#105780),(#105781,#105782,#105783),
(#105784,#105785,#105786),(#105787,#105788,#105789),(#105790,#105791,#105792),
(#105793,#105794,#105795),(#105796,#105797,#105798),(#105799,#105800,#105801),
(#105802,#105803,#105804),(#105805,#105806,#105807),(#105808,#105809,#105810),
(#105811,#105812,#105813),(#105814,#105815,#105816),(#105817,#105818,#105819),
(#105820,#105821,#105822),(#105823,#105824,#105825),(#105826,#105827,#105828),
(#105829,#105830,#105831),(#105832,#105833,#105834),(#105835,#105836,#105837),
(#105838,#105839,#105840),(#105841,#105842,#105843),(#105844,#105845,#105846),
(#105847,#105848,#105849),(#105850,#105851,#105852),(#105853,#105854,#105855),
(#105856,#105857,#105858),(#105859,#105860,#105861),(#105862,#105863,#105864),
(#105865,#105866,#105867),(#105868,#105869,#105870),(#105871,#105872,#105873),
(#105874,#105875,#105876),(#105877,#105878,#105879),(#105880,#105881,#105882),
(#105883,#105884,#105885),(#105886,#105887,#105888),(#105889,#105890,#105891),
(#105892,#105893,#105894),(#105895,#105896,#105897),(#105898,#105899,#105900),
(#105901,#105902,#105903),(#105904,#105905,#105906),(#105907,#105908,#105909),
(#105910,#105911,#105912),(#105913,#105914,#105915),(#105916,#105917,#105918),
(#105919,#105920,#105921),(#105922,#105923,#105924),(#105925,#105926,#105927),
(#105928,#105929,#105930),(#105931,#105932,#105933),(#105934,#105935,#105936)),
 .UNSPECIFIED.,.F.,.F.,.F.)
B_SPLINE_SURFACE_WITH_KNOTS((4,2,2,2,2,2,2,2,2,2,2,2,2,2,2,2,2,2,2,2,2,
2,2,2,2,2,2,4),(3,3),(0.0511475161397767,0.0543755745194946,0.0559748561230095,
0.0575741377265244,0.0591734193300392,0.0607727009335541,0.062371982537069,
0.0639712641405839,0.0671698273476136,0.0687691089511285,0.0703683905546434,
0.0735669537616731,0.0743665945634306,0.075166235365188,0.0767655169687029,
0.0783647985722178,0.0799640801757326,0.0831626433827624,0.0839622841845198,
0.0847619249862773,0.0863612065897922,0.087960488193307,0.0895597697968219,
0.0911590514003368,0.0927583330038517,0.0959568962108814,0.0991554594179112,
0.102525861223878),(-0.000171838598937368,1.),.UNSPECIFIED.)
GEOMETRIC_REPRESENTATION_ITEM()
RATIONAL_B_SPLINE_SURFACE(((1.00021865031188,0.363791624143024,1.),(1.00022479681566,
0.345907098154518,1.),(1.00022920060531,0.333093359896605,1.),(1.00023129551577,
0.326997783970377,1.),(1.00023123364639,0.327177805750004,1.),(1.00022969489106,
0.331655133124608,1.),(1.00022822047137,0.33594526264943,1.),(1.0002240867261,
0.347973250814052,1.),(1.00022140814422,0.35576713965136,1.),(1.00021534117809,
0.373420234385561,1.),(1.00021194541535,0.383300909504994,1.),(1.00020471008312,
0.404353607436186,1.),(1.00020086574039,0.415539518961325,1.),(1.00019293747055,
0.438608462395977,1.),(1.00018890288822,0.450347915466388,1.),(1.00017677850116,
0.485626331191368,1.),(1.00016867552582,0.509203616458618,1.),(1.00015692182764,
0.543403436110339,1.),(1.00015305594815,0.554652013302536,1.),(1.00014555866706,
0.576466905683628,1.),(1.00014195877655,0.586941532845051,1.),(1.00013165871491,
0.616911695858456,1.),(1.0001254526397,0.634969557244874,1.),(1.00011873943879,
0.654503005935684,1.),(1.0001174494347,0.658256540079135,1.),(1.00011498233984,
0.665435063621729,1.),(1.00011380138062,0.668871309120393,1.),(1.00011047639801,
0.678546034793393,1.),(1.00010854790581,0.684157382338519,1.),(1.00010529091615,
0.693634268435905,1.),(1.00010396227248,0.697500232426158,1.),(1.00010194478336,
0.703370534929476,1.),(1.00010125711622,0.705371444929324,1.),(1.00010025379618,
0.708290812429403,1.),(1.00010095148053,0.706260755280883,1.),(1.00010350708302,
0.698824700439302,1.),(1.00010410506401,0.697084750890896,1.),(1.00010545207932,
0.693165330790809,1.),(1.00010620231782,0.690982356485965,1.),(1.00010867300391,
0.683793383480134,1.),(1.00011061292529,0.678148780393428,1.),(1.00011503809133,
0.665272843129747,1.),(1.00011753618207,0.658004130630299,1.),(1.00012299044327,
0.642133827810658,1.),(1.00012593037118,0.633579498550827,1.),(1.00013218440859,
0.615382081200487,1.),(1.00013549875609,0.605738300581923,1.),(1.00014246105377,
0.585480053220453,1.),(1.00014612511713,0.574818701874222,1.),(1.00015740340534,
0.542002186013824,1.),(1.00016532224555,0.518960680057816,1.),(1.00018150784987,
0.471865311436827,1.),(1.00018984724106,0.447600125261974,1.),(1.00020595223619,
0.400739305781631,1.),(1.00021372551999,0.378121326326883,1.),(1.00021994210994,
0.36003287010178,1.)))
REPRESENTATION_ITEM('')
SURFACE()
);
#1680=(
BOUNDED_SURFACE()
B_SPLINE_SURFACE(3,2,((#106162,#106163,#106164),(#106165,#106166,#106167),
(#106168,#106169,#106170),(#106171,#106172,#106173),(#106174,#106175,#106176),
(#106177,#106178,#106179),(#106180,#106181,#106182),(#106183,#106184,#106185),
(#106186,#106187,#106188),(#106189,#106190,#106191),(#106192,#106193,#106194),
(#106195,#106196,#106197)),.UNSPECIFIED.,.F.,.F.,.F.)
B_SPLINE_SURFACE_WITH_KNOTS((4,2,2,2,2,4),(3,3),(0.0020168056312046,0.00318801267491835,
0.00435921971863209,0.00670163380605957,0.00904404789348706,0.0113864619809145),
(0.,1.),.UNSPECIFIED.)
GEOMETRIC_REPRESENTATION_ITEM()
RATIONAL_B_SPLINE_SURFACE(((1.,0.707106781186548,1.),(1.,0.734176096219266,
1.),(1.,0.758590233751572,1.),(1.,0.803187254291515,1.),(1.,0.823368840149339,
1.),(1.,0.878495386168538,1.),(1.,0.908178291941153,1.),(1.,0.954777204682283,
1.),(1.,0.971753344320815,1.),(1.,0.994387335841996,1.),(1.,0.999999540046553,
1.),(1.,1.,1.)))
REPRESENTATION_ITEM('')
SURFACE()
);
#1681=(
BOUNDED_SURFACE()
B_SPLINE_SURFACE(3,2,((#106201,#106202,#106203),(#106204,#106205,#106206),
(#106207,#106208,#106209),(#106210,#106211,#106212),(#106213,#106214,#106215),
(#106216,#106217,#106218),(#106219,#106220,#106221),(#106222,#106223,#106224),
(#106225,#106226,#106227),(#106228,#106229,#106230),(#106231,#106232,#106233),
(#106234,#106235,#106236)),.UNSPECIFIED.,.F.,.F.,.F.)
B_SPLINE_SURFACE_WITH_KNOTS((4,2,2,2,2,4),(3,3),(0.00201680563120466,0.00318801267491843,
0.00435921971863221,0.00670163380605975,0.0090440478934873,0.0113864619809148),
(0.,1.),.UNSPECIFIED.)
GEOMETRIC_REPRESENTATION_ITEM()
RATIONAL_B_SPLINE_SURFACE(((1.,0.707106781186548,1.),(1.,0.734176096219302,
1.),(1.,0.758590233751572,1.),(1.,0.803187254291516,1.),(1.,0.823368840149552,
1.),(1.,0.878495386168105,1.),(1.,0.908178291940607,1.),(1.,0.954777204682866,
1.),(1.,0.971753344320825,1.),(1.,0.994387335842007,1.),(1.,0.999999540046577,
1.),(1.,1.,1.)))
REPRESENTATION_ITEM('')
SURFACE()
);
#1682=(
BOUNDED_SURFACE()
B_SPLINE_SURFACE(3,2,((#106403,#106404,#106405),(#106406,#106407,#106408),
(#106409,#106410,#106411),(#106412,#106413,#106414),(#106415,#106416,#106417),
(#106418,#106419,#106420),(#106421,#106422,#106423),(#106424,#106425,#106426),
(#106427,#106428,#106429),(#106430,#106431,#106432)),.UNSPECIFIED.,.F.,
 .F.,.F.)
B_SPLINE_SURFACE_WITH_KNOTS((4,2,2,2,4),(3,3),(0.,0.000214020122328381,
0.000428040244656761,0.000642060366985142,0.000856080489313522),(0.,1.),
 .UNSPECIFIED.)
GEOMETRIC_REPRESENTATION_ITEM()
RATIONAL_B_SPLINE_SURFACE(((1.,0.707106781186548,1.),(1.,0.68347722662262,
1.),(1.,0.659481175544654,1.),(1.,0.610508879439021,1.),(1.,0.585996172067873,
1.),(1.,0.540858044367121,1.),(1.,0.519989927806179,1.),(1.,0.489650895143399,
1.),(1.,0.480786371092266,1.),(1.,0.480804881866771,1.)))
REPRESENTATION_ITEM('')
SURFACE()
);
#1683=(
BOUNDED_SURFACE()
B_SPLINE_SURFACE(3,2,((#106441,#106442,#106443),(#106444,#106445,#106446),
(#106447,#106448,#106449),(#106450,#106451,#106452),(#106453,#106454,#106455),
(#106456,#106457,#106458),(#106459,#106460,#106461),(#106462,#106463,#106464),
(#106465,#106466,#106467),(#106468,#106469,#106470),(#106471,#106472,#106473),
(#106474,#106475,#106476),(#106477,#106478,#106479),(#106480,#106481,#106482)),
 .UNSPECIFIED.,.F.,.F.,.F.)
B_SPLINE_SURFACE_WITH_KNOTS((4,2,2,2,2,2,4),(3,3),(-8.59074174355445E-5,
0.000107384271794359,0.000214768543588717,0.000322152815383076,0.000429537087177435,
0.000644305630766152,0.000944981591790375),(-0.00127279735662637,1.),
 .UNSPECIFIED.)
GEOMETRIC_REPRESENTATION_ITEM()
RATIONAL_B_SPLINE_SURFACE(((1.0013127144284,0.484319156713673,1.),(1.00132886473298,
0.477974743557733,1.),(1.0013261987696,0.47902202864576,1.),(1.00129711892767,
0.490445623210585,1.),(1.00128159687351,0.496543237288905,1.),(1.00124353256439,
0.511496249612038,1.),(1.00122061910444,0.520497470359364,1.),(1.00117008762078,
0.540348031566809,1.),(1.0011427053451,0.551104761827022,1.),(1.00105582580784,
0.585234129241031,1.),(1.00099333442134,0.609782964990972,1.),(1.00084281910852,
0.668910724817792,1.),(1.00075790617431,0.70226754071777,1.),(1.00067489566942,
0.734877014827455,1.)))
REPRESENTATION_ITEM('')
SURFACE()
);
#1684=(
BOUNDED_SURFACE()
B_SPLINE_SURFACE(3,2,((#106494,#106495,#106496),(#106497,#106498,#106499),
(#106500,#106501,#106502),(#106503,#106504,#106505),(#106506,#106507,#106508),
(#106509,#106510,#106511),(#106512,#106513,#106514),(#106515,#106516,#106517),
(#106518,#106519,#106520),(#106521,#106522,#106523)),.UNSPECIFIED.,.F.,
 .F.,.F.)
B_SPLINE_SURFACE_WITH_KNOTS((4,2,2,2,4),(3,3),(0.,0.000214020122328381,
0.000428040244656761,0.000642060366985142,0.000856080489313522),(0.,1.),
 .UNSPECIFIED.)
GEOMETRIC_REPRESENTATION_ITEM()
RATIONAL_B_SPLINE_SURFACE(((1.,0.707106781186548,1.),(1.,0.68347722662262,
1.),(1.,0.659481175544654,1.),(1.,0.610508879439021,1.),(1.,0.585996172067677,
1.),(1.,0.540858044367307,1.),(1.,0.519989927806563,1.),(1.,0.489650895143026,
1.),(1.,0.480786371092547,1.),(1.,0.480804881866766,1.)))
REPRESENTATION_ITEM('')
SURFACE()
);
#1685=(
BOUNDED_SURFACE()
B_SPLINE_SURFACE(3,2,((#106531,#106532,#106533),(#106534,#106535,#106536),
(#106537,#106538,#106539),(#106540,#106541,#106542),(#106543,#106544,#106545),
(#106546,#106547,#106548),(#106549,#106550,#106551),(#106552,#106553,#106554),
(#106555,#106556,#106557),(#106558,#106559,#106560),(#106561,#106562,#106563),
(#106564,#106565,#106566),(#106567,#106568,#106569),(#106570,#106571,#106572)),
 .UNSPECIFIED.,.F.,.F.,.F.)
B_SPLINE_SURFACE_WITH_KNOTS((4,2,2,2,2,2,4),(3,3),(-8.59074174354856E-5,
0.000107384271794357,0.000214768543588714,0.000322152815383071,0.000429537087177428,
0.000644305630766142,0.00094498159179036),(0.,1.00128352994005),
 .UNSPECIFIED.)
GEOMETRIC_REPRESENTATION_ITEM()
RATIONAL_B_SPLINE_SURFACE(((1.,0.484313629162157,1.00132379779329),(1.,
0.477969147999695,1.00134008445634),(1.,0.47901644431411,1.00133739598399),
(1.,0.490440161327499,1.00130807061837),(1.,0.496537840765783,1.00129241751012),
(1.,0.511491013369546,1.00125403182065),(1.,0.520492330600339,1.00123092490032),
(1.,0.540343104584769,1.00117996677483),(1.,0.551099950145726,1.00115235330815),
(1.,0.585229683390388,1.00106474023922),(1.,0.609778782278141,1.00100172123238),
(1.,0.668907175891151,1.00084993510536),(1.,0.702264349342087,1.00076430524368),
(1.,0.734874172989235,1.0006805938737)))
REPRESENTATION_ITEM('')
SURFACE()
);
#2294=B_SPLINE_CURVE_WITH_KNOTS('',3,(#97323,#97324,#97325,#97326,#97327,
#97328,#97329,#97330,#97331,#97332,#97333,#97334,#97335,#97336,#97337,#97338,
#97339,#97340,#97341,#97342,#97343,#97344,#97345,#97346,#97347,#97348,#97349,
#97350,#97351,#97352,#97353,#97354,#97355,#97356,#97357,#97358,#97359),
 .UNSPECIFIED.,.F.,.F.,(4,3,3,3,3,3,3,3,3,3,3,3,4),(-2.78934132800095E-5,
0.00121588438262122,0.00221227975556897,0.00221609308686091,0.00384184723093993,
0.00445245292441795,0.00445837553689522,0.00611808335700871,0.00669262609326693,
0.00669744820440185,0.00781574891708038,0.00880510804235627,0.00893279926211591),
 .UNSPECIFIED.);
#2295=B_SPLINE_CURVE_WITH_KNOTS('',3,(#97363,#97364,#97365,#97366,#97367,
#97368,#97369,#97370,#97371,#97372,#97373,#97374,#97375,#97376,#97377,#97378,
#97379,#97380,#97381,#97382,#97383,#97384,#97385,#97386,#97387,#97388,#97389,
#97390,#97391,#97392,#97393,#97394,#97395,#97396,#97397,#97398,#97399,#97400,
#97401,#97402,#97403,#97404,#97405),.UNSPECIFIED.,.F.,.F.,(4,3,3,3,3,3,
3,3,3,3,3,3,3,3,4),(0.,0.000981863058810054,0.00110848267565544,0.00221820625791767,
0.00222304486987606,0.00387027745216958,0.00444010558372466,0.00444608973975211,
0.00605994093001663,0.00666519007157424,0.00666913460962817,0.00778065704456617,
0.00833641826203515,0.00866716277185096,0.00889217947950412),
 .UNSPECIFIED.);
#2296=B_SPLINE_CURVE_WITH_KNOTS('',3,(#97603,#97604,#97605,#97606,#97607,
#97608,#97609,#97610,#97611,#97612,#97613,#97614,#97615,#97616,#97617,#97618,
#97619,#97620,#97621,#97622,#97623,#97624,#97625,#97626,#97627,#97628,#97629,
#97630,#97631,#97632,#97633,#97634,#97635,#97636,#97637,#97638,#97639,#97640,
#97641,#97642,#97643,#97644,#97645,#97646,#97647,#97648,#97649,#97650,#97651,
#97652,#97653,#97654,#97655,#97656,#97657,#97658,#97659,#97660,#97661,#97662,
#97663,#97664,#97665,#97666,#97667,#97668,#97669,#97670,#97671,#97672,#97673,
#97674,#97675,#97676,#97677,#97678,#97679,#97680,#97681,#97682,#97683,#97684,
#97685,#97686,#97687,#97688,#97689,#97690,#97691,#97692,#97693,#97694,#97695,
#97696,#97697,#97698,#97699,#97700,#97701,#97702,#97703,#97704,#97705,#97706,
#97707,#97708,#97709,#97710,#97711,#97712,#97713,#97714,#97715,#97716,#97717,
#97718,#97719,#97720,#97721,#97722,#97723,#97724,#97725,#97726,#97727,#97728,
#97729,#97730,#97731,#97732,#97733,#97734,#97735,#97736,#97737,#97738,#97739,
#97740,#97741,#97742,#97743,#97744,#97745,#97746,#97747,#97748,#97749,#97750,
#97751,#97752,#97753,#97754,#97755,#97756,#97757,#97758,#97759,#97760,#97761,
#97762,#97763,#97764,#97765,#97766,#97767,#97768,#97769,#97770,#97771,#97772,
#97773,#97774,#97775,#97776,#97777),.UNSPECIFIED.,.F.,.F.,(4,3,3,3,3,3,
3,3,3,3,3,3,3,3,3,3,3,3,3,3,3,3,3,3,3,3,3,3,3,3,3,3,3,3,3,3,3,3,3,3,3,3,
3,3,3,3,3,3,3,3,3,3,3,3,3,3,3,3,4),(0.,7.00136229228457E-5,0.000880271419196664,
0.0019798005518509,0.00250406869828295,0.00300266268960072,0.00331712911283043,
0.00413059578319972,0.00532772256795508,0.0057574742158991,0.00600532537920143,
0.00738304200408563,0.00900794430850163,0.00900798806880215,0.0112899391799351,
0.0120106507584029,0.012257034623011,0.0135119821032032,0.0138815868497288,
0.0147250110536992,0.0150133134480036,0.0155067088258864,0.0168452146168024,
0.0180159761376041,0.0187586550708965,0.0195173074824044,0.0203855296680284,
0.0210186388272047,0.0220135800001955,0.0236425023713016,0.0240213015168053,
0.0244570699511878,0.0252717472664166,0.0255226328616056,0.0270239642064059,
0.0285252955512062,0.0285300848199135,0.0293428874314649,0.0300266268960065,
0.0301588925271162,0.0313458910919412,0.0317871551652159,0.033029289585607,
0.0334140923804464,0.0345306209304072,0.0350404780787164,0.0360319522752075,
0.0366663282699642,0.0375332836200077,0.0382915981957547,0.039034614964808,
0.0412861444649818,0.0415405183457811,0.0420372776544085,0.0431651404778179,
0.0447901356468785,0.045039940344009,0.0470573761230531,0.0480426030336095),
 .UNSPECIFIED.);
#2297=B_SPLINE_CURVE_WITH_KNOTS('',3,(#97781,#97782,#97783,#97784,#97785,
#97786,#97787,#97788,#97789,#97790,#97791,#97792,#97793,#97794,#97795,#97796,
#97797,#97798,#97799,#97800,#97801,#97802,#97803,#97804,#97805,#97806,#97807,
#97808,#97809,#97810,#97811,#97812,#97813,#97814,#97815,#97816,#97817,#97818,
#97819,#97820,#97821,#97822,#97823,#97824,#97825,#97826,#97827,#97828,#97829,
#97830,#97831,#97832,#97833,#97834,#97835,#97836,#97837,#97838),
 .UNSPECIFIED.,.F.,.F.,(4,2,2,2,2,2,2,2,2,2,2,2,2,2,2,2,2,2,2,2,2,2,2,2,
2,2,2,2,4),(0.0557463281926296,0.0589772878231815,0.0605927676384573,0.0622082474537332,
0.0654392070842851,0.067054686899561,0.068670166714837,0.0702856465301129,
0.0719011263453888,0.0735166061606648,0.0751320859759407,0.0783630456064926,
0.0791707855141306,0.0799785254217686,0.0815940052370446,0.0832094850523206,
0.0848249648675966,0.0880559244981484,0.0896714043134243,0.0912868841287003,
0.0945178437592521,0.096133323574528,0.0977488033898038,0.0993642832050797,
0.100979763020356,0.102595242835631,0.103402982743269,0.104210722650907,
0.107441682281459),.UNSPECIFIED.);
#2298=B_SPLINE_CURVE_WITH_KNOTS('',3,(#97841,#97842,#97843,#97844,#97845,
#97846,#97847,#97848),.UNSPECIFIED.,.F.,.F.,(4,2,2,4),(0.100097362857501,
0.102091718402555,0.103088896175082,0.104086073947609),.UNSPECIFIED.);
#2299=B_SPLINE_CURVE_WITH_KNOTS('',3,(#98007,#98008,#98009,#98010,#98011,
#98012,#98013,#98014,#98015,#98016,#98017,#98018,#98019,#98020,#98021,#98022,
#98023,#98024,#98025,#98026,#98027,#98028,#98029,#98030,#98031,#98032,#98033,
#98034,#98035,#98036,#98037,#98038,#98039,#98040,#98041,#98042,#98043,#98044,
#98045,#98046,#98047,#98048,#98049,#98050,#98051,#98052,#98053,#98054,#98055,
#98056,#98057,#98058,#98059,#98060),.UNSPECIFIED.,.F.,.F.,(4,2,2,2,2,2,
2,2,2,2,2,2,2,2,2,2,2,2,2,2,2,2,2,2,2,2,4),(0.,0.00156341081501294,0.00312682163002588,
0.00469023244503882,0.00625364326005176,0.00938046489007764,0.0109438757050905,
0.0125072865201034,0.0156341081501293,0.0171975189651422,0.0187609297801551,
0.021887751410181,0.0226694568176875,0.023451162225194,0.0250145730402071,
0.0265779838552202,0.0281413946702332,0.0312682163002594,0.0328316271152726,
0.0343950379302857,0.037521859560312,0.0406486811903383,0.0422120920053514,
0.0437755028203645,0.0469023244503908,0.0484657352654039,0.050029146080417),
 .UNSPECIFIED.);
#2300=B_SPLINE_CURVE_WITH_KNOTS('',3,(#98064,#98065,#98066,#98067,#98068,
#98069,#98070,#98071,#98072,#98073,#98074,#98075,#98076,#98077,#98078,#98079,
#98080,#98081,#98082,#98083,#98084,#98085,#98086,#98087,#98088,#98089,#98090,
#98091,#98092,#98093,#98094,#98095,#98096,#98097,#98098,#98099,#98100,#98101,
#98102,#98103,#98104,#98105,#98106,#98107,#98108,#98109,#98110,#98111,#98112,
#98113,#98114,#98115,#98116,#98117,#98118,#98119,#98120,#98121,#98122,#98123,
#98124,#98125,#98126,#98127,#98128,#98129,#98130,#98131,#98132,#98133,#98134,
#98135,#98136,#98137,#98138,#98139,#98140,#98141,#98142,#98143,#98144,#98145,
#98146,#98147,#98148,#98149,#98150,#98151,#98152,#98153,#98154,#98155,#98156,
#98157,#98158,#98159,#98160,#98161,#98162,#98163,#98164,#98165,#98166,#98167,
#98168,#98169,#98170,#98171,#98172,#98173,#98174,#98175,#98176,#98177,#98178,
#98179,#98180,#98181,#98182,#98183,#98184,#98185,#98186,#98187,#98188,#98189,
#98190,#98191,#98192,#98193,#98194,#98195,#98196,#98197,#98198,#98199,#98200,
#98201,#98202,#98203,#98204,#98205,#98206,#98207,#98208,#98209,#98210,#98211,
#98212,#98213,#98214,#98215,#98216,#98217,#98218,#98219,#98220,#98221,#98222,
#98223,#98224,#98225,#98226,#98227,#98228,#98229,#98230,#98231,#98232,#98233,
#98234,#98235,#98236,#98237,#98238,#98239,#98240,#98241,#98242,#98243,#98244,
#98245,#98246,#98247,#98248,#98249,#98250,#98251,#98252,#98253,#98254,#98255,
#98256,#98257,#98258,#98259,#98260,#98261,#98262,#98263,#98264,#98265,#98266,
#98267,#98268,#98269,#98270,#98271,#98272,#98273,#98274,#98275,#98276,#98277,
#98278,#98279,#98280,#98281,#98282,#98283,#98284,#98285,#98286),
 .UNSPECIFIED.,.F.,.F.,(4,3,3,3,3,3,3,3,3,3,3,3,3,3,3,3,3,3,3,3,3,3,3,3,
3,3,3,3,3,3,3,3,3,3,3,3,3,3,3,3,3,3,3,3,3,3,3,3,3,3,3,3,3,3,3,3,3,3,3,3,
3,3,3,3,3,3,3,3,3,3,3,3,3,3,4),(0.0536197899396224,0.0552276244004005,0.0552355709876449,
0.0564636360418572,0.056836730186764,0.0568513520356673,0.0585010989847782,
0.0600604289236084,0.0600829141317123,0.0616747375677009,0.0616986951797348,
0.0631694062564205,0.0632905117196436,0.0633144762277572,0.0653332916269836,
0.0665264501713466,0.0665460383238021,0.0680226211562579,0.0681465613676236,
0.0681618193718244,0.06976797630888,0.0697776004198467,0.0713906714255839,
0.0713933814678691,0.0730091625158914,0.0730146093723317,0.0752607556615613,
0.0762407246119361,0.0762648548190899,0.0777231476585644,0.0778565056599585,
0.0778906973850273,0.0791924472927823,0.0794722867079808,0.0795162256569394,
0.0810880677560031,0.0811414459847621,0.0823878645715334,0.0827038488040255,
0.082765970222281,0.0844200933214001,0.0859354109000701,0.0860114915248442,
0.0868961672851169,0.0875511919480923,0.0887466775681185,0.0891669729961145,
0.0892519026800105,0.0907827540441368,0.090869989342466,0.0922381233776412,
0.092398535092159,0.0924866314778508,0.0942502320947687,0.0956300971882036,
0.0957154955381664,0.0971616980108514,0.0972458782362259,0.0973274461005371,
0.0983010085687395,0.0988616592842482,0.0989376222126474,0.0999829246183408,
0.10047744033227,0.100546243852972,0.101152494922683,0.101724341209355,
0.102093221380293,0.102150357244739,0.102702522250809,0.102901111904304,
0.103522312960999,0.103709002428315,0.104937728080031,0.105324783476337),
 .UNSPECIFIED.);
#2301=B_SPLINE_CURVE_WITH_KNOTS('',3,(#98289,#98290,#98291,#98292,#98293,
#98294,#98295,#98296,#98297,#98298),.UNSPECIFIED.,.F.,.F.,(4,3,3,4),(0.101994009991496,
0.102941137438368,0.103427904624697,0.103888264885239),.UNSPECIFIED.);
#2302=B_SPLINE_CURVE_WITH_KNOTS('',3,(#98451,#98452,#98453,#98454,#98455,
#98456,#98457,#98458,#98459,#98460,#98461,#98462,#98463,#98464,#98465,#98466,
#98467,#98468,#98469,#98470,#98471,#98472,#98473,#98474,#98475,#98476,#98477,
#98478,#98479,#98480,#98481,#98482,#98483,#98484,#98485,#98486,#98487,#98488,
#98489,#98490,#98491,#98492,#98493,#98494,#98495,#98496,#98497,#98498,#98499,
#98500,#98501,#98502,#98503,#98504,#98505,#98506,#98507,#98508,#98509,#98510,
#98511,#98512,#98513,#98514,#98515,#98516,#98517,#98518,#98519,#98520,#98521,
#98522,#98523,#98524,#98525,#98526,#98527,#98528,#98529,#98530,#98531,#98532,
#98533,#98534,#98535,#98536,#98537,#98538,#98539,#98540,#98541,#98542,#98543,
#98544,#98545,#98546,#98547,#98548,#98549,#98550,#98551,#98552,#98553,#98554,
#98555,#98556,#98557,#98558,#98559,#98560,#98561,#98562,#98563,#98564,#98565,
#98566,#98567,#98568,#98569,#98570,#98571,#98572,#98573,#98574,#98575,#98576,
#98577,#98578,#98579,#98580,#98581,#98582,#98583,#98584,#98585,#98586,#98587,
#98588,#98589,#98590,#98591,#98592,#98593,#98594,#98595,#98596,#98597,#98598,
#98599,#98600,#98601,#98602,#98603,#98604,#98605,#98606,#98607,#98608,#98609,
#98610,#98611,#98612,#98613,#98614,#98615,#98616,#98617,#98618,#98619,#98620,
#98621,#98622,#98623,#98624,#98625,#98626,#98627,#98628,#98629,#98630,#98631,
#98632,#98633,#98634,#98635,#98636,#98637,#98638,#98639,#98640,#98641,#98642,
#98643,#98644,#98645,#98646,#98647,#98648,#98649,#98650,#98651,#98652,#98653,
#98654,#98655,#98656,#98657,#98658,#98659,#98660,#98661,#98662,#98663,#98664),
 .UNSPECIFIED.,.F.,.F.,(4,3,3,3,3,3,3,3,3,3,3,3,3,3,3,3,3,3,3,3,3,3,3,3,
3,3,3,3,3,3,3,3,3,3,3,3,3,3,3,3,3,3,3,3,3,3,3,3,3,3,3,3,3,3,3,3,3,3,3,3,
3,3,3,3,3,3,3,3,3,3,3,4),(0.,0.000919480979115724,0.00186665391132834,0.00222303890370072,
0.00246023501007185,0.00308006741790905,0.00345996891983424,0.00369035251510777,
0.00469778641362988,0.00492047002014368,0.00577875096527111,0.00593619564291903,
0.0061505875251796,0.00691217011934619,0.00717505541494653,0.00738070503021552,
0.00841742521904112,0.00946182449544975,0.00965322408999175,0.00984094004028725,
0.0105271968013281,0.0108924604402717,0.0110710575453231,0.0121313588744037,
0.012301175050359,0.0135614282722711,0.014608084951402,0.0147614100604307,
0.0155427428163806,0.0158457881834858,0.0159915275654665,0.0170831200839182,
0.0172216450705023,0.0180163683085217,0.0183201098374356,0.0184517625755382,
0.0191739816007994,0.0195568018131331,0.019681880080574,0.0208560722381215,
0.022030264395669,0.0221421150906457,0.0229078739324747,0.0232673524625759,
0.0233722325956815,0.0245048134750372,0.0246023501007174,0.0254360756730852,
0.0257427490373535,0.0258324676057532,0.026634352472142,0.0269811460780055,
0.027062585110789,0.0284787188530985,0.0294588729843419,0.0295228201208608,
0.0310014861472265,0.0319371442892161,0.0319830551309325,0.0335148785821422,
0.0344145418676413,0.0344432901410042,0.0353749506244627,0.0356525636344977,
0.0356734076460401,0.0368901184213511,0.036903525151076,0.0375185839035939,
0.0381336426561119,0.0385671407304436,0.0389938437394034,0.0393637601611478),
 .UNSPECIFIED.);
#2303=B_SPLINE_CURVE_WITH_KNOTS('',3,(#98668,#98669,#98670,#98671,#98672,
#98673,#98674,#98675,#98676,#98677,#98678,#98679,#98680,#98681,#98682,#98683,
#98684,#98685,#98686,#98687,#98688,#98689,#98690,#98691,#98692,#98693,#98694,
#98695,#98696,#98697,#98698,#98699,#98700,#98701,#98702,#98703,#98704,#98705,
#98706,#98707,#98708,#98709,#98710,#98711,#98712,#98713,#98714,#98715,#98716,
#98717,#98718,#98719,#98720,#98721,#98722,#98723,#98724,#98725,#98726,#98727,
#98728,#98729,#98730,#98731,#98732,#98733,#98734,#98735,#98736,#98737,#98738,
#98739,#98740,#98741,#98742,#98743,#98744,#98745,#98746,#98747,#98748,#98749,
#98750,#98751,#98752,#98753,#98754,#98755,#98756,#98757,#98758,#98759,#98760,
#98761,#98762,#98763,#98764,#98765,#98766,#98767,#98768,#98769,#98770,#98771,
#98772,#98773,#98774,#98775,#98776,#98777,#98778,#98779,#98780,#98781,#98782,
#98783,#98784,#98785,#98786,#98787,#98788,#98789,#98790,#98791,#98792,#98793,
#98794,#98795,#98796,#98797,#98798,#98799,#98800,#98801,#98802,#98803,#98804,
#98805,#98806,#98807,#98808,#98809,#98810,#98811,#98812,#98813,#98814,#98815,
#98816,#98817,#98818,#98819,#98820,#98821,#98822,#98823,#98824,#98825,#98826,
#98827,#98828,#98829,#98830,#98831,#98832,#98833,#98834,#98835,#98836,#98837,
#98838,#98839,#98840,#98841,#98842,#98843,#98844,#98845,#98846,#98847,#98848,
#98849,#98850,#98851,#98852,#98853,#98854,#98855,#98856,#98857,#98858,#98859,
#98860,#98861,#98862,#98863,#98864,#98865,#98866),.UNSPECIFIED.,.F.,.F.,
(4,3,3,3,3,3,3,3,3,3,3,3,3,3,3,3,3,3,3,3,3,3,3,3,3,3,3,3,3,3,3,3,3,3,3,
3,3,3,3,3,3,3,3,3,3,3,3,3,3,3,3,3,3,3,3,3,3,3,3,3,3,3,3,3,3,3,4),(0.0415609574076441,
0.0419999079181991,0.0424456108255438,0.0428514400237989,0.0434891733075762,
0.0441269065913535,0.0441419226399537,0.0454112381061315,0.0454324052561084,
0.0465323604471359,0.0466965822688831,0.0467228878722632,0.0484820040278885,
0.0492715033675918,0.0493038531045728,0.0507359116685006,0.0518516607057079,
0.0518848183368824,0.0535408116929441,0.0544369446773842,0.054465783569192,
0.0555110612925173,0.0557314168323167,0.0557562661853469,0.0570268987744937,
0.0570467488015017,0.0580899941195753,0.0583234009749456,0.0583372314176566,
0.0593028016533825,0.0596206777396424,0.0596277140338114,0.0622086792661211,
0.0622163187211141,0.063499161882276,0.0635142754825525,0.0647896444984309,
0.0648116296745799,0.0660801271145858,0.0661083966471777,0.0673706097307407,
0.0674045134523431,0.0688635319843868,0.0699515749630503,0.0699933139595394,
0.0712420575792051,0.0712859635838355,0.0722808578694621,0.0725325401953599,
0.0725774037566074,0.0740349703453863,0.0751135054276695,0.0751563211290189,
0.0761837854504516,0.0764039880438243,0.0764437283836802,0.07758048125962,
0.0776944706599792,0.0777298862469095,0.078984953276134,0.0790147568862244,
0.0801773798799933,0.0802754358922888,0.0802979121042526,0.0811942832430352,
0.082067096754397,0.0828564011245984),.UNSPECIFIED.);
#2304=B_SPLINE_CURVE_WITH_KNOTS('',3,(#98873,#98874,#98875,#98876,#98877,
#98878,#98879,#98880,#98881,#98882,#98883,#98884,#98885,#98886,#98887,#98888,
#98889,#98890,#98891,#98892,#98893,#98894,#98895,#98896,#98897,#98898),
 .UNSPECIFIED.,.F.,.F.,(4,2,2,2,2,2,2,2,2,2,2,2,4),(0.,0.24105520274149,
0.482110405482979,0.964220810965958,1.44228868010388,1.68132261467284,1.9203565492418,
2.15939048381076,2.39842441837972,2.87649228751764,3.35860269300062,3.59965789574211,
3.8407130984836),.UNSPECIFIED.);
#2305=B_SPLINE_CURVE_WITH_KNOTS('',3,(#98902,#98903,#98904,#98905,#98906,
#98907,#98908,#98909,#98910,#98911,#98912,#98913,#98914,#98915,#98916,#98917,
#98918,#98919,#98920,#98921,#98922,#98923,#98924,#98925,#98926,#98927,#98928,
#98929,#98930,#98931,#98932,#98933,#98934,#98935,#98936,#98937,#98938,#98939,
#98940,#98941,#98942,#98943,#98944,#98945,#98946,#98947,#98948,#98949,#98950,
#98951,#98952,#98953),.UNSPECIFIED.,.F.,.F.,(4,2,2,2,2,2,2,2,2,2,2,2,2,
2,2,2,2,2,2,2,2,2,2,2,2,4),(0.0396248818917768,0.0420848252462827,0.0433147969235357,
0.0445447686007886,0.0457747402780416,0.0470047119552946,0.0494646553098004,
0.0506946269870533,0.0519245986643062,0.0543845420188121,0.055614513696065,
0.0568444853733179,0.0593044287278237,0.0605344004050766,0.0617643720823295,
0.0629943437595824,0.0642243154368353,0.0666842587913412,0.0679142304685941,
0.069144202145847,0.0703741738231,0.0716041455003529,0.0740640888548589,
0.075294060532112,0.076524032209365,0.078983975563871),.UNSPECIFIED.);
#2306=B_SPLINE_CURVE_WITH_KNOTS('',3,(#98954,#98955,#98956,#98957,#98958,
#98959,#98960,#98961,#98962,#98963,#98964,#98965,#98966,#98967,#98968,#98969,
#98970,#98971,#98972,#98973,#98974,#98975,#98976,#98977,#98978,#98979),
 .UNSPECIFIED.,.F.,.F.,(4,2,2,2,2,2,2,2,2,2,2,2,4),(3.8407130984836,4.08176830122509,
4.32282350396658,4.80493390944956,5.28300177858748,5.52203571315644,5.7610696477254,
6.00010358229436,6.23913751686332,6.71720538600124,7.19931579148422,7.4403709942257,
7.68142619696719),.UNSPECIFIED.);
#2307=B_SPLINE_CURVE_WITH_KNOTS('',3,(#98982,#98983,#98984,#98985,#98986,
#98987,#98988,#98989,#98990,#98991,#98992,#98993,#98994,#98995,#98996,#98997,
#98998,#98999,#99000,#99001,#99002,#99003,#99004,#99005,#99006,#99007,#99008,
#99009,#99010,#99011,#99012,#99013,#99014,#99015,#99016,#99017,#99018,#99019,
#99020,#99021,#99022,#99023,#99024,#99025,#99026,#99027,#99028,#99029,#99030,
#99031,#99032,#99033,#99034,#99035,#99036,#99037,#99038,#99039,#99040,#99041,
#99042,#99043,#99044,#99045,#99046,#99047,#99048,#99049,#99050,#99051,#99052,
#99053,#99054,#99055,#99056,#99057,#99058,#99059,#99060,#99061,#99062,#99063,
#99064,#99065,#99066,#99067,#99068,#99069,#99070,#99071,#99072,#99073,#99074,
#99075,#99076,#99077,#99078,#99079,#99080,#99081,#99082,#99083,#99084,#99085,
#99086,#99087,#99088,#99089,#99090,#99091,#99092,#99093,#99094,#99095,#99096,
#99097,#99098,#99099,#99100,#99101,#99102,#99103,#99104,#99105,#99106,#99107,
#99108,#99109,#99110,#99111,#99112,#99113,#99114,#99115,#99116,#99117,#99118,
#99119,#99120,#99121,#99122,#99123,#99124,#99125,#99126,#99127,#99128,#99129,
#99130,#99131,#99132,#99133,#99134,#99135,#99136,#99137,#99138,#99139,#99140,
#99141,#99142,#99143,#99144,#99145,#99146,#99147,#99148,#99149,#99150,#99151,
#99152,#99153,#99154,#99155,#99156,#99157,#99158,#99159,#99160,#99161,#99162,
#99163,#99164,#99165,#99166,#99167,#99168,#99169,#99170,#99171,#99172,#99173,
#99174,#99175,#99176,#99177,#99178,#99179,#99180,#99181,#99182,#99183,#99184,
#99185,#99186),.UNSPECIFIED.,.F.,.F.,(4,3,3,3,3,3,3,3,3,3,3,3,3,3,3,3,3,
3,3,3,3,3,3,3,3,3,3,3,3,3,3,3,3,3,3,3,3,3,3,3,3,3,3,3,3,3,3,3,3,3,3,3,3,
3,3,3,3,3,3,3,3,3,3,3,3,3,3,3,4),(0.051952788832463,0.0523437358727679,
0.0530396348010571,0.0532815940436916,0.0535165769936827,0.0550803651549024,
0.0565315459304904,0.0566441533161221,0.0573435791058262,0.0581553062489573,
0.0582079414773418,0.0597781972481067,0.0613355177997813,0.0614004919138027,
0.0627595431985349,0.0628993059610011,0.0630224461823626,0.0644630941222208,
0.0662665572770309,0.0675906704446604,0.0678890579253496,0.0688036127964488,
0.0691544586058802,0.0695121857757964,0.0705623247810647,0.0707182467671,
0.0722820349283198,0.0727603963114584,0.0735729358548261,0.0738458230895395,
0.0743855823551034,0.0760111644019605,0.0769733994119791,0.0775954188217194,
0.0776371348320698,0.077755293492589,0.0783329590758319,0.0784502993253913,
0.078537187573199,0.079263366729678,0.0801009757344188,0.0816647638956387,
0.0825143971297319,0.0832285520568585,0.0853698372313069,0.0857634780397393,
0.0863561283792982,0.0870860429658391,0.087387128745137,0.087919916540518,
0.0890096229688163,0.0894837047017378,0.0904433744731794,0.0906319233369377,
0.0910474928629577,0.0918522904268007,0.0922540308854936,0.0926112810241775,
0.0947257451244876,0.0954981621844028,0.095738857346617,0.0966800930537362,
0.0971208482525779,0.0973026455078367,0.0981728563859435,0.0987443411160432,
0.0988664336690564,0.100855253342667,0.101994009991496),.UNSPECIFIED.);
#2308=B_SPLINE_CURVE_WITH_KNOTS('',3,(#99189,#99190,#99191,#99192,#99193,
#99194,#99195,#99196,#99197,#99198),.UNSPECIFIED.,.F.,.F.,(4,2,2,2,4),(0.0480426030336095,
0.0490467205767583,0.050050838119907,0.0510549556630558,0.0520590732062046),
 .UNSPECIFIED.);
#2309=B_SPLINE_CURVE_WITH_KNOTS('',3,(#99199,#99200,#99201,#99202,#99203,
#99204,#99205,#99206,#99207,#99208,#99209,#99210,#99211,#99212,#99213,#99214,
#99215,#99216,#99217,#99218,#99219,#99220,#99221,#99222,#99223,#99224,#99225,
#99226,#99227,#99228,#99229,#99230,#99231,#99232,#99233,#99234,#99235,#99236,
#99237,#99238,#99239,#99240,#99241,#99242,#99243,#99244,#99245,#99246,#99247,
#99248),.UNSPECIFIED.,.F.,.F.,(4,2,2,2,2,2,2,2,2,2,2,2,2,2,2,2,2,2,2,2,
2,2,2,2,4),(0.0520590732062046,0.0550614663094106,0.0558120645852121,0.0565626628610136,
0.0580638594126164,0.0595650559642193,0.0610662525158222,0.0640686456190281,
0.0655698421706311,0.0670710387222342,0.0700734318254403,0.0715746283770435,
0.0730758249286465,0.0760782180318527,0.0775794145834557,0.0790806111350588,
0.0805818076866618,0.0820830042382648,0.0850853973414709,0.0880877904446769,
0.0910901835478829,0.094092576651089,0.095593773202692,0.097094969754295,
0.100097362857501),.UNSPECIFIED.);
#2310=B_SPLINE_CURVE_WITH_KNOTS('',3,(#99249,#99250,#99251,#99252,#99253,
#99254,#99255,#99256,#99257,#99258,#99259,#99260,#99261,#99262,#99263,#99264,
#99265,#99266,#99267,#99268,#99269,#99270,#99271,#99272,#99273),
 .UNSPECIFIED.,.F.,.F.,(4,3,3,3,3,3,3,3,4),(0.050029146080417,0.0504604958563201,
0.0505100567684285,0.0509435518624639,0.05099096745644,0.0514718781444515,
0.0516554513507709,0.0517123334884572,0.0519527888232233),.UNSPECIFIED.);
#2311=B_SPLINE_CURVE_WITH_KNOTS('',3,(#99414,#99415,#99416,#99417,#99418,
#99419,#99420,#99421,#99422,#99423,#99424,#99425,#99426,#99427,#99428,#99429,
#99430,#99431,#99432,#99433,#99434,#99435,#99436,#99437,#99438,#99439,#99440,
#99441,#99442,#99443,#99444,#99445,#99446,#99447,#99448,#99449,#99450,#99451,
#99452,#99453,#99454,#99455,#99456,#99457,#99458,#99459,#99460,#99461,#99462,
#99463,#99464,#99465,#99466,#99467,#99468,#99469,#99470,#99471,#99472,#99473,
#99474,#99475,#99476,#99477,#99478,#99479,#99480,#99481,#99482,#99483,#99484,
#99485,#99486,#99487,#99488,#99489,#99490,#99491,#99492,#99493,#99494,#99495,
#99496,#99497,#99498,#99499,#99500,#99501,#99502,#99503,#99504,#99505,#99506,
#99507,#99508,#99509,#99510,#99511,#99512,#99513,#99514,#99515,#99516,#99517,
#99518,#99519,#99520,#99521,#99522,#99523,#99524,#99525,#99526,#99527,#99528,
#99529,#99530,#99531,#99532,#99533,#99534,#99535,#99536,#99537,#99538,#99539,
#99540,#99541,#99542,#99543,#99544,#99545,#99546,#99547,#99548,#99549,#99550,
#99551,#99552,#99553,#99554,#99555,#99556,#99557,#99558),.UNSPECIFIED.,
 .F.,.F.,(4,3,3,3,3,3,3,3,3,3,3,3,3,3,3,3,3,3,3,3,3,3,3,3,3,3,3,3,3,3,3,
3,3,3,3,3,3,3,3,3,3,3,3,3,3,3,3,3,4),(0.0203612017522921,0.0208877325613553,
0.0214142633704186,0.0215214199490211,0.0222272019780885,0.022467324988545,
0.0226816347878761,0.0232615135447818,0.0235203866066714,0.0238415310374913,
0.0244196285836592,0.0245734482247979,0.0250017753684234,0.0250999790338611,
0.0254745069658603,0.0255817617933977,0.0256265098429244,0.0261621061518675,
0.0266795714610508,0.027093539205275,0.0273236651342074,0.0277326330791773,
0.0284867951362316,0.0287856946973038,0.0290694919072253,0.0296527825000932,
0.0298387563154302,0.030424002716454,0.0308207212525154,0.0308918179335567,
0.0314448180467838,0.0319448795516832,0.0319897325623951,0.0328989778740624,
0.0329979411698097,0.033158038557521,0.0337415514971665,0.0340510027879362,
0.0343244349253117,0.034906676680582,0.0351040644060626,0.0354884218747967,
0.0359549037492386,0.0361571260241891,0.0364421515354402,0.0366539939248379,
0.0369320907835768,0.0371958940818509,0.0372101876423156),.UNSPECIFIED.);
#2312=B_SPLINE_CURVE_WITH_KNOTS('',3,(#99562,#99563,#99564,#99565,#99566,
#99567,#99568,#99569,#99570,#99571,#99572,#99573,#99574,#99575,#99576,#99577,
#99578,#99579,#99580,#99581,#99582,#99583,#99584,#99585,#99586,#99587,#99588,
#99589,#99590,#99591,#99592,#99593,#99594,#99595,#99596,#99597,#99598,#99599,
#99600,#99601,#99602,#99603,#99604,#99605,#99606,#99607,#99608,#99609,#99610,
#99611,#99612,#99613,#99614,#99615,#99616,#99617,#99618,#99619,#99620,#99621,
#99622,#99623,#99624,#99625,#99626,#99627,#99628,#99629,#99630,#99631,#99632,
#99633,#99634,#99635,#99636,#99637,#99638,#99639,#99640,#99641,#99642,#99643,
#99644,#99645,#99646,#99647,#99648,#99649,#99650,#99651,#99652,#99653,#99654,
#99655,#99656,#99657,#99658,#99659,#99660,#99661,#99662,#99663,#99664,#99665,
#99666,#99667,#99668,#99669,#99670,#99671,#99672,#99673,#99674,#99675,#99676,
#99677,#99678,#99679,#99680,#99681,#99682,#99683,#99684,#99685,#99686,#99687,
#99688,#99689,#99690,#99691,#99692,#99693,#99694,#99695,#99696,#99697,#99698,
#99699,#99700,#99701,#99702,#99703,#99704,#99705,#99706,#99707,#99708,#99709,
#99710,#99711,#99712,#99713,#99714,#99715,#99716,#99717,#99718,#99719,#99720,
#99721,#99722,#99723,#99724,#99725,#99726,#99727,#99728,#99729,#99730,#99731,
#99732,#99733,#99734,#99735,#99736,#99737,#99738,#99739,#99740,#99741,#99742,
#99743,#99744,#99745),.UNSPECIFIED.,.F.,.F.,(4,3,3,3,3,3,3,3,3,3,3,3,3,
3,3,3,3,3,3,3,3,3,3,3,3,3,3,3,3,3,3,3,3,3,3,3,3,3,3,3,3,3,3,3,3,3,3,3,3,
3,3,3,3,3,3,3,3,3,3,3,3,4),(0.0393915580945953,0.0406020192817889,0.0406842633633433,
0.0406958727203922,0.0411897366401807,0.041347511295112,0.0417997522419474,
0.0419769686320912,0.042001060508596,0.0427295402264934,0.0432696739008392,
0.0433092324285996,0.0438450851123192,0.0439160265352132,0.043962195669524,
0.0444511285765506,0.0445623791695872,0.044613777558144,0.0452087318039612,
0.0452639875668987,0.0457762976609016,0.0458550844383352,0.0459128163539046,
0.0466311140589519,0.0471477897070833,0.047205819393466,0.047825754424214,
0.0484404949758313,0.0484929313137353,0.0492161864185054,0.0497332002445794,
0.0497750420548443,0.0502299672427955,0.0503795528789534,0.0504143578583252,
0.0509624748546795,0.0510259055133274,0.0510532316307843,0.0523186107820755,
0.0523300368138618,0.053160842001516,0.0536076953320472,0.0536113160508235,
0.0542478903539933,0.0542576686851976,0.0547677584017706,0.0548891050414737,
0.0549040213195716,0.0557559568875907,0.0561762838139536,0.0561967265883197,
0.0567415483777051,0.0568222920920382,0.0568430792226938,0.0574699119703464,
0.0574894318570679,0.0582050150642818,0.0587698423842959,0.058782137125816,
0.0593635404971942,0.0599514576204697,0.0600748423945641),.UNSPECIFIED.);
#2313=B_SPLINE_CURVE_WITH_KNOTS('',3,(#99748,#99749,#99750,#99751,#99752,
#99753),.UNSPECIFIED.,.F.,.F.,(4,2,4),(1.4304896245382E-17,0.000879674198175861,
0.00175934839635171),.UNSPECIFIED.);
#2314=B_SPLINE_CURVE_WITH_KNOTS('',3,(#99918,#99919,#99920,#99921,#99922,
#99923,#99924,#99925,#99926,#99927,#99928,#99929,#99930,#99931,#99932,#99933,
#99934,#99935,#99936,#99937,#99938,#99939,#99940,#99941,#99942,#99943,#99944,
#99945,#99946,#99947,#99948,#99949,#99950,#99951,#99952,#99953,#99954,#99955,
#99956,#99957,#99958,#99959,#99960,#99961,#99962,#99963,#99964,#99965,#99966,
#99967,#99968,#99969,#99970,#99971),.UNSPECIFIED.,.F.,.F.,(4,2,2,2,2,2,
2,2,2,2,2,2,2,2,2,2,2,2,2,2,2,2,2,2,2,2,4),(0.0425666836577637,0.0437586716581344,
0.0449506596585051,0.0473346356592465,0.0485266236596173,0.0497186116599881,
0.0521025876607297,0.0532945756611006,0.0544865636614714,0.0556785516618422,
0.056870539662213,0.0592545156629546,0.0604465036633254,0.0616384916636961,
0.0628304796640669,0.0640224676644376,0.066406443665179,0.0675984316655497,
0.0687904196659204,0.0711743956666619,0.0723663836670326,0.0735583716674033,
0.0759423476681446,0.0771343356685152,0.0783263236688858,0.0795183116692565,
0.0807102996696271),.UNSPECIFIED.);
#2315=B_SPLINE_CURVE_WITH_KNOTS('',3,(#99975,#99976,#99977,#99978,#99979,
#99980,#99981,#99982,#99983,#99984,#99985,#99986,#99987,#99988,#99989,#99990,
#99991,#99992,#99993,#99994,#99995,#99996,#99997,#99998,#99999,#100000,
#100001,#100002,#100003,#100004,#100005,#100006,#100007,#100008,#100009,
#100010,#100011,#100012,#100013,#100014,#100015,#100016,#100017,#100018,
#100019,#100020,#100021,#100022,#100023,#100024,#100025,#100026,#100027,
#100028,#100029,#100030),.UNSPECIFIED.,.F.,.F.,(4,2,2,2,2,2,2,2,2,2,2,2,
2,2,2,2,2,2,2,2,2,2,2,2,2,2,2,4),(0.0826968326824961,0.0840239767822064,
0.0853511208819168,0.0866782649816271,0.0880054090813374,0.0893325531810478,
0.0906596972807581,0.0933139854801787,0.0946411295798889,0.0959682736795991,
0.0986225618790196,0.0999497059787299,0.10127685007844,0.10260399417815,
0.103931138277861,0.106585426477281,0.107912570576991,0.109239714676702,
0.110566858776412,0.111894002876122,0.114548291075542,0.115875435175253,
0.117202579274963,0.118529723374673,0.119856867474383,0.122511155673804,
0.123838299773514,0.125165443873224),.UNSPECIFIED.);
#2316=B_SPLINE_CURVE_WITH_KNOTS('',3,(#100033,#100034,#100035,#100036,#100037,
#100038,#100039,#100040,#100041,#100042,#100043,#100044,#100045),
 .UNSPECIFIED.,.F.,.F.,(4,3,3,3,4),(5.74602846774033E-18,0.00103091965574787,
0.00109496199515262,0.00213421079951866,0.00218992399030524),
 .UNSPECIFIED.);
#2317=B_SPLINE_CURVE_WITH_KNOTS('',3,(#100210,#100211,#100212,#100213,#100214,
#100215,#100216,#100217,#100218,#100219,#100220,#100221,#100222,#100223,
#100224,#100225,#100226,#100227,#100228,#100229,#100230,#100231,#100232,
#100233,#100234,#100235,#100236,#100237,#100238,#100239,#100240,#100241,
#100242,#100243,#100244,#100245,#100246,#100247,#100248,#100249,#100250,
#100251,#100252,#100253,#100254,#100255,#100256,#100257,#100258,#100259,
#100260,#100261,#100262,#100263),.UNSPECIFIED.,.F.,.F.,(4,2,2,2,2,2,2,2,
2,2,2,2,2,2,2,2,2,2,2,2,2,2,2,2,2,2,4),(0.0425666836577637,0.0437586716581344,
0.0449506596585051,0.0473346356592465,0.0485266236596173,0.0497186116599881,
0.0521025876607297,0.0532945756611006,0.0544865636614714,0.0556785516618422,
0.056870539662213,0.0592545156629546,0.0604465036633254,0.0616384916636961,
0.0628304796640669,0.0640224676644376,0.066406443665179,0.0675984316655497,
0.0687904196659204,0.0711743956666619,0.0723663836670326,0.0735583716674033,
0.0759423476681446,0.0771343356685152,0.0783263236688858,0.0795183116692565,
0.0807102996696271),.UNSPECIFIED.);
#2318=B_SPLINE_CURVE_WITH_KNOTS('',3,(#100267,#100268,#100269,#100270,#100271,
#100272,#100273,#100274,#100275,#100276,#100277,#100278,#100279,#100280,
#100281,#100282,#100283,#100284,#100285,#100286,#100287,#100288,#100289,
#100290,#100291,#100292,#100293,#100294,#100295,#100296,#100297,#100298,
#100299,#100300,#100301,#100302,#100303,#100304,#100305,#100306,#100307,
#100308,#100309,#100310,#100311,#100312,#100313,#100314,#100315,#100316,
#100317,#100318,#100319,#100320,#100321,#100322),.UNSPECIFIED.,.F.,.F.,
(4,2,2,2,2,2,2,2,2,2,2,2,2,2,2,2,2,2,2,2,2,2,2,2,2,2,2,4),(0.0826968326824961,
0.0840239767822064,0.0853511208819168,0.0866782649816271,0.0880054090813374,
0.0893325531810478,0.0906596972807581,0.0933139854801787,0.0946411295798889,
0.0959682736795991,0.0986225618790196,0.0999497059787299,0.10127685007844,
0.10260399417815,0.103931138277861,0.106585426477281,0.107912570576991,
0.109239714676702,0.110566858776412,0.111894002876122,0.114548291075542,
0.115875435175253,0.117202579274963,0.118529723374673,0.119856867474383,
0.122511155673804,0.123838299773514,0.125165443873224),.UNSPECIFIED.);
#2319=B_SPLINE_CURVE_WITH_KNOTS('',3,(#100325,#100326,#100327,#100328,#100329,
#100330,#100331,#100332,#100333,#100334,#100335,#100336,#100337),
 .UNSPECIFIED.,.F.,.F.,(4,3,3,3,4),(5.74602846774033E-18,0.00103091965584011,
0.00109496199515262,0.00213421079971333,0.00218992399030524),
 .UNSPECIFIED.);
#2320=B_SPLINE_CURVE_WITH_KNOTS('',3,(#100352,#100353,#100354,#100355,#100356,
#100357,#100358,#100359,#100360,#100361,#100362,#100363,#100364,#100365,
#100366,#100367,#100368,#100369,#100370,#100371,#100372,#100373,#100374,
#100375,#100376,#100377,#100378,#100379,#100380,#100381,#100382,#100383,
#100384,#100385,#100386,#100387,#100388,#100389,#100390,#100391,#100392,
#100393,#100394,#100395,#100396,#100397,#100398,#100399,#100400,#100401,
#100402,#100403,#100404,#100405,#100406,#100407,#100408,#100409,#100410,
#100411,#100412,#100413,#100414,#100415,#100416,#100417,#100418,#100419,
#100420,#100421,#100422,#100423,#100424,#100425,#100426,#100427,#100428,
#100429,#100430,#100431,#100432,#100433,#100434,#100435,#100436,#100437,
#100438,#100439,#100440,#100441,#100442,#100443,#100444,#100445,#100446,
#100447,#100448,#100449,#100450,#100451,#100452,#100453,#100454,#100455,
#100456,#100457,#100458,#100459,#100460,#100461,#100462,#100463,#100464,
#100465,#100466,#100467,#100468,#100469,#100470,#100471,#100472,#100473,
#100474,#100475,#100476,#100477,#100478,#100479,#100480,#100481,#100482,
#100483,#100484,#100485,#100486,#100487,#100488,#100489,#100490,#100491,
#100492,#100493,#100494,#100495,#100496,#100497,#100498,#100499,#100500,
#100501,#100502,#100503,#100504,#100505,#100506,#100507,#100508,#100509,
#100510,#100511,#100512,#100513,#100514,#100515,#100516,#100517,#100518,
#100519,#100520,#100521,#100522,#100523,#100524,#100525,#100526,#100527,
#100528,#100529,#100530,#100531,#100532,#100533,#100534,#100535,#100536,
#100537,#100538,#100539,#100540,#100541,#100542,#100543,#100544),
 .UNSPECIFIED.,.F.,.F.,(4,3,3,3,3,3,3,3,3,3,3,3,3,3,3,3,3,3,3,3,3,3,3,3,
3,3,3,3,3,3,3,3,3,3,3,3,3,3,3,3,3,3,3,3,3,3,3,3,3,3,3,3,3,3,3,3,3,3,3,3,
3,3,3,3,4),(0.00218992399030524,0.00308955832189556,0.004018478740376,0.00457303964936322,
0.00471820601332814,0.00528919436517401,0.00576459747889221,0.00599015957137656,
0.0064977592807818,0.00695615530842121,0.00724973709061845,0.00855234536231135,
0.0093392709674792,0.00977080820653486,0.0105308287970081,0.0110350977515803,
0.0117223866265371,0.012299424271805,0.0131312412090355,0.0135628412595257,
0.0141055022855951,0.0148235883463824,0.0156561031455178,0.0164886179446531,
0.0171451126945242,0.0173447902188242,0.0176801757741821,0.0181792030037352,
0.0186034896216875,0.0188717336037111,0.0196753837693712,0.0198625075997739,
0.0206539618856476,0.0211202966732222,0.0212548492627691,0.0219966235055716,
0.0223781033376274,0.0231455767622806,0.0236379649218272,0.0245470980206528,
0.0248989158279885,0.0258457255439288,0.0260210805808852,0.0274226554767584,
0.0284041962399432,0.0286863596781406,0.0299508419517926,0.0307873118990013,
0.0320722689041744,0.0324806915917337,0.0331704275580593,0.0337099622359248,
0.0342395035047979,0.0343619853875884,0.0350082143941416,0.0355535432171174,
0.0362707981721182,0.0367451010466465,0.0372671387162966,0.0375316513660662,
0.0379366588761756,0.0389074701956465,0.0398687342463795,0.0400497152061118,
0.0403197745314809),.UNSPECIFIED.);
#2321=B_SPLINE_CURVE_WITH_KNOTS('',3,(#100547,#100548,#100549,#100550,#100551,
#100552),.UNSPECIFIED.,.F.,.F.,(4,2,4),(0.0403197745352163,0.04144322909649,
0.0425666836577637),.UNSPECIFIED.);
#2322=B_SPLINE_CURVE_WITH_KNOTS('',3,(#100553,#100554,#100555,#100556,#100557,
#100558,#100559,#100560,#100561,#100562,#100563,#100564,#100565,#100566,
#100567,#100568,#100569,#100570,#100571,#100572,#100573,#100574,#100575,
#100576,#100577,#100578,#100579,#100580,#100581,#100582,#100583,#100584,
#100585,#100586,#100587,#100588,#100589,#100590,#100591,#100592,#100593,
#100594,#100595,#100596,#100597,#100598,#100599,#100600,#100601,#100602,
#100603,#100604,#100605,#100606,#100607,#100608,#100609,#100610,#100611,
#100612,#100613,#100614,#100615,#100616,#100617,#100618,#100619,#100620,
#100621,#100622,#100623,#100624,#100625,#100626,#100627,#100628,#100629,
#100630,#100631,#100632,#100633,#100634,#100635,#100636,#100637,#100638,
#100639,#100640,#100641,#100642,#100643,#100644,#100645,#100646,#100647,
#100648,#100649,#100650,#100651,#100652,#100653,#100654,#100655,#100656,
#100657,#100658,#100659,#100660,#100661,#100662,#100663,#100664,#100665,
#100666,#100667,#100668,#100669,#100670,#100671,#100672,#100673,#100674,
#100675,#100676,#100677,#100678,#100679,#100680,#100681,#100682,#100683,
#100684,#100685,#100686,#100687,#100688,#100689,#100690,#100691,#100692,
#100693,#100694,#100695,#100696,#100697,#100698,#100699,#100700,#100701,
#100702,#100703,#100704,#100705,#100706,#100707,#100708,#100709,#100710,
#100711,#100712,#100713,#100714,#100715,#100716,#100717,#100718,#100719,
#100720,#100721,#100722,#100723,#100724,#100725,#100726,#100727,#100728,
#100729,#100730,#100731,#100732,#100733,#100734,#100735,#100736,#100737,
#100738,#100739,#100740,#100741,#100742,#100743,#100744,#100745),
 .UNSPECIFIED.,.F.,.F.,(4,3,3,3,3,3,3,3,3,3,3,3,3,3,3,3,3,3,3,3,3,3,3,3,
3,3,3,3,3,3,3,3,3,3,3,3,3,3,3,3,3,3,3,3,3,3,3,3,3,3,3,3,3,3,3,3,3,3,3,3,
3,3,3,3,4),(0.00218992399030524,0.00308955832192262,0.00401847874043237,
0.0045730396493621,0.00471820601332802,0.00528919436515712,0.00576459747889057,
0.00599015957137656,0.00649775928078463,0.00695615530841904,0.00724973709061851,
0.00855234536240134,0.00933927096747599,0.00977080820653491,0.0105308287970044,
0.0110350977515804,0.0117223866265329,0.0122994242718053,0.0131312412090609,
0.0135628412595259,0.0141055022855899,0.0148235883463828,0.0156561031455148,
0.0164886179446468,0.0171451126945234,0.0173447902188245,0.0176801757741753,
0.0181792030037235,0.0186034896216878,0.0188717336037037,0.0196753837693461,
0.0198625075997741,0.0206539618856354,0.0211202966732224,0.0212548492627606,
0.0219966235055572,0.0223781033376276,0.0231455767622747,0.0236379649218175,
0.0245470980206775,0.0248989158279887,0.0258457255439675,0.0260210805808744,
0.0274226554767585,0.0284041962399313,0.0286863596781406,0.0299508419517927,
0.0307873118989883,0.0320722689041961,0.0324806915917337,0.0331704275580452,
0.0337099622359205,0.0342395035047928,0.0343619853875737,0.0350082143941417,
0.0355535432171022,0.0362707981721182,0.0367451010466307,0.0372671387162828,
0.0375316513660662,0.0379366588761592,0.0389074701956399,0.0398687342463254,
0.0400497152061118,0.0403197745314634),.UNSPECIFIED.);
#2323=B_SPLINE_CURVE_WITH_KNOTS('',3,(#100746,#100747,#100748,#100749,#100750,
#100751),.UNSPECIFIED.,.F.,.F.,(4,2,4),(0.0403197745352337,0.0414432290964987,
0.0425666836577637),.UNSPECIFIED.);
#2324=B_SPLINE_CURVE_WITH_KNOTS('',3,(#100754,#100755,#100756,#100757,#100758,
#100759,#100760,#100761,#100762,#100763,#100764,#100765,#100766,#100767,
#100768,#100769,#100770,#100771,#100772,#100773,#100774,#100775,#100776,
#100777,#100778,#100779,#100780,#100781,#100782,#100783,#100784,#100785,
#100786,#100787,#100788,#100789,#100790,#100791,#100792,#100793,#100794,
#100795,#100796,#100797,#100798,#100799,#100800,#100801,#100802,#100803,
#100804,#100805,#100806,#100807,#100808,#100809,#100810,#100811,#100812,
#100813,#100814,#100815,#100816,#100817,#100818,#100819,#100820,#100821,
#100822,#100823,#100824,#100825,#100826,#100827,#100828,#100829,#100830,
#100831,#100832,#100833,#100834,#100835,#100836,#100837,#100838,#100839,
#100840,#100841,#100842,#100843,#100844,#100845,#100846,#100847,#100848,
#100849,#100850,#100851,#100852,#100853,#100854,#100855,#100856,#100857,
#100858,#100859,#100860,#100861,#100862,#100863,#100864,#100865,#100866,
#100867,#100868,#100869,#100870,#100871,#100872,#100873,#100874,#100875,
#100876,#100877,#100878,#100879,#100880,#100881,#100882,#100883,#100884,
#100885,#100886,#100887,#100888,#100889,#100890,#100891,#100892,#100893,
#100894,#100895,#100896,#100897,#100898,#100899,#100900,#100901,#100902,
#100903,#100904,#100905,#100906,#100907,#100908,#100909,#100910,#100911,
#100912,#100913,#100914,#100915,#100916,#100917,#100918,#100919,#100920,
#100921,#100922,#100923,#100924,#100925,#100926,#100927,#100928,#100929,
#100930,#100931,#100932,#100933,#100934,#100935,#100936,#100937,#100938,
#100939,#100940,#100941,#100942,#100943,#100944,#100945,#100946,#100947,
#100948,#100949,#100950,#100951,#100952,#100953,#100954,#100955,#100956,
#100957,#100958,#100959,#100960,#100961,#100962,#100963,#100964,#100965,
#100966,#100967,#100968,#100969,#100970,#100971,#100972,#100973),
 .UNSPECIFIED.,.F.,.F.,(4,3,3,3,3,3,3,3,3,3,3,3,3,3,3,3,3,3,3,3,3,3,3,3,
3,3,3,3,3,3,3,3,3,3,3,3,3,3,3,3,3,3,3,3,3,3,3,3,3,3,3,3,3,3,3,3,3,3,3,3,
3,3,3,3,3,3,3,3,3,3,3,3,3,4),(0.00398066249725657,0.00520970825651315,0.00650636077682542,
0.00721601660321733,0.00723521461508359,0.00790676989862768,0.00859462407436548,
0.0088336936561977,0.00953736387305569,0.010259563370406,0.0104513707091781,
0.0104840369026883,0.0122603887891099,0.0136867248151388,0.0137089680572726,
0.0147832361856882,0.0153044018681193,0.0153241614395351,0.0169220789210998,
0.0169382407877385,0.0185397559740803,0.0185508989686889,0.0201574330270607,
0.0201622062086101,0.0217724235733863,0.0217751100800412,0.0225771129414008,
0.0225839486065314,0.0233815379211718,0.0233927871330216,0.0251680184799019,
0.0265986566873695,0.0266281412389824,0.0276739747417877,0.0282071183667835,
0.0282458182919628,0.0298163947543849,0.0298634953449433,0.0314265764578142,
0.0314811723979237,0.0322320258870935,0.033037874608938,0.0330988494509041,
0.0353209486500281,0.0362648283008095,0.0363342035568649,0.0372867356601343,
0.0378804048033753,0.0379518806098454,0.0388901500916239,0.0394973460129241,
0.0395695576628258,0.0417194838636053,0.0427357414432794,0.0428049117687866,
0.0443574142826654,0.0459808396568091,0.0460402658747474,0.0470431195999113,
0.0476060477279055,0.0476579429277278,0.0487984511437497,0.0492332173564472,
0.0492756199807082,0.0505099933557396,0.0508616218729735,0.0520424580018409,
0.0524903086159866,0.0525109740866689,0.0535033159543337,0.0541286511396493,
0.0546624608776011,0.0552149480467196,0.0557463281926296),.UNSPECIFIED.);
#2325=B_SPLINE_CURVE_WITH_KNOTS('',3,(#100976,#100977,#100978,#100979,#100980,
#100981,#100982,#100983,#100984,#100985,#100986,#100987,#100988,#100989,
#100990,#100991,#100992,#100993,#100994,#100995,#100996,#100997,#100998,
#100999,#101000,#101001,#101002,#101003,#101004,#101005,#101006,#101007,
#101008,#101009,#101010,#101011,#101012,#101013,#101014,#101015,#101016,
#101017,#101018,#101019,#101020,#101021,#101022,#101023,#101024,#101025,
#101026,#101027,#101028,#101029,#101030,#101031,#101032,#101033,#101034,
#101035,#101036,#101037,#101038,#101039,#101040,#101041,#101042,#101043,
#101044,#101045,#101046,#101047,#101048,#101049,#101050,#101051,#101052,
#101053,#101054,#101055,#101056,#101057,#101058,#101059,#101060,#101061,
#101062,#101063,#101064,#101065,#101066,#101067,#101068,#101069,#101070,
#101071,#101072,#101073,#101074,#101075,#101076,#101077,#101078,#101079,
#101080,#101081,#101082,#101083,#101084,#101085,#101086,#101087,#101088,
#101089,#101090,#101091,#101092,#101093,#101094,#101095,#101096,#101097,
#101098,#101099,#101100,#101101,#101102,#101103,#101104,#101105,#101106,
#101107,#101108,#101109,#101110,#101111,#101112,#101113,#101114,#101115,
#101116,#101117,#101118,#101119,#101120,#101121,#101122,#101123,#101124,
#101125,#101126,#101127,#101128,#101129,#101130,#101131,#101132,#101133,
#101134,#101135,#101136,#101137,#101138,#101139,#101140,#101141,#101142,
#101143,#101144,#101145,#101146,#101147,#101148,#101149,#101150,#101151,
#101152,#101153,#101154,#101155,#101156,#101157,#101158,#101159,#101160,
#101161,#101162,#101163,#101164,#101165,#101166,#101167,#101168,#101169,
#101170,#101171,#101172,#101173,#101174,#101175,#101176,#101177,#101178,
#101179,#101180,#101181,#101182,#101183,#101184,#101185,#101186,#101187,
#101188,#101189,#101190,#101191,#101192,#101193,#101194,#101195),
 .UNSPECIFIED.,.F.,.F.,(4,3,3,3,3,3,3,3,3,3,3,3,3,3,3,3,3,3,3,3,3,3,3,3,
3,3,3,3,3,3,3,3,3,3,3,3,3,3,3,3,3,3,3,3,3,3,3,3,3,3,3,3,3,3,3,3,3,3,3,3,
3,3,3,3,3,3,3,3,3,3,3,3,3,4),(0.00398066249725657,0.00520970825644499,0.00650636077671913,
0.00721601660321733,0.00723521461508372,0.00790676989864398,0.00859462407441027,
0.0088336936561977,0.00953736387311957,0.0102595633704823,0.0104513707091781,
0.0104840369026883,0.0122603887890039,0.0136867248151388,0.0137089680572725,
0.0147832361856785,0.0153044018681193,0.015324161439535,0.0169220789210998,
0.0169382407877384,0.0185397559740803,0.0185508989686889,0.0201574330270607,
0.0201622062086101,0.0217724235733863,0.0217751100800412,0.0225771129414007,
0.0225839486065314,0.0233815379211717,0.0233927871330216,0.0251680184799104,
0.0265986566873695,0.0266281412389824,0.027673974741794,0.0282071183667836,
0.0282458182919628,0.0298163947543848,0.0298634953449433,0.0314265764578142,
0.0314811723979237,0.0322320258870934,0.0330378746089379,0.0330988494509041,
0.0353209486498751,0.0362648283008094,0.0363342035568649,0.0372867356600656,
0.0378804048033753,0.0379518806098454,0.0388901500916096,0.0394973460129241,
0.0395695576628258,0.0417194838637361,0.0427357414432794,0.0428049117687866,
0.0443574142826654,0.045980839656809,0.0460402658747474,0.0470431195998788,
0.0476060477279055,0.0476579429277278,0.0487984511436461,0.0492332173564472,
0.0492756199807082,0.0505099933557137,0.0508616218729735,0.0520424580018639,
0.0524903086159865,0.0525109740866689,0.0535033159542304,0.0541286511396493,
0.0546624608775954,0.0552149480467123,0.0557463281926296),.UNSPECIFIED.);
#2326=B_SPLINE_CURVE_WITH_KNOTS('',3,(#101196,#101197,#101198,#101199,#101200,
#101201,#101202,#101203,#101204,#101205,#101206,#101207,#101208,#101209,
#101210,#101211,#101212,#101213,#101214,#101215,#101216,#101217,#101218,
#101219,#101220,#101221,#101222,#101223,#101224,#101225,#101226,#101227,
#101228,#101229,#101230,#101231,#101232,#101233,#101234,#101235,#101236,
#101237,#101238,#101239,#101240,#101241,#101242,#101243,#101244,#101245,
#101246,#101247,#101248,#101249,#101250,#101251,#101252,#101253),
 .UNSPECIFIED.,.F.,.F.,(4,2,2,2,2,2,2,2,2,2,2,2,2,2,2,2,2,2,2,2,2,2,2,2,
2,2,2,2,4),(0.0557463281926296,0.0589772878231815,0.0605927676384573,0.0622082474537332,
0.0654392070842851,0.067054686899561,0.068670166714837,0.0702856465301129,
0.0719011263453888,0.0735166061606648,0.0751320859759407,0.0783630456064926,
0.0791707855141306,0.0799785254217686,0.0815940052370446,0.0832094850523206,
0.0848249648675966,0.0880559244981484,0.0896714043134243,0.0912868841287003,
0.0945178437592521,0.096133323574528,0.0977488033898038,0.0993642832050797,
0.100979763020356,0.102595242835631,0.103402982743269,0.104210722650907,
0.107441682281459),.UNSPECIFIED.);
#2327=B_SPLINE_CURVE_WITH_KNOTS('',3,(#101254,#101255,#101256,#101257,#101258,
#101259,#101260,#101261,#101262,#101263,#101264,#101265,#101266,#101267,
#101268,#101269,#101270,#101271,#101272,#101273,#101274,#101275,#101276,
#101277,#101278,#101279,#101280,#101281,#101282,#101283,#101284,#101285,
#101286,#101287,#101288,#101289,#101290,#101291,#101292,#101293,#101294,
#101295,#101296,#101297,#101298,#101299,#101300,#101301,#101302,#101303,
#101304,#101305,#101306,#101307,#101308,#101309,#101310,#101311,#101312,
#101313,#101314,#101315,#101316,#101317,#101318,#101319,#101320,#101321,
#101322,#101323,#101324,#101325,#101326,#101327,#101328,#101329,#101330,
#101331,#101332,#101333,#101334,#101335,#101336,#101337,#101338,#101339,
#101340,#101341,#101342,#101343,#101344,#101345,#101346,#101347,#101348,
#101349,#101350,#101351,#101352,#101353,#101354,#101355,#101356,#101357,
#101358,#101359,#101360,#101361,#101362,#101363,#101364,#101365,#101366,
#101367,#101368,#101369,#101370,#101371,#101372,#101373,#101374,#101375,
#101376,#101377,#101378,#101379,#101380,#101381,#101382,#101383,#101384,
#101385,#101386,#101387,#101388,#101389,#101390,#101391,#101392,#101393,
#101394,#101395,#101396,#101397,#101398,#101399,#101400,#101401,#101402,
#101403,#101404,#101405,#101406,#101407,#101408,#101409,#101410,#101411,
#101412,#101413,#101414,#101415,#101416,#101417,#101418,#101419,#101420,
#101421,#101422,#101423,#101424,#101425,#101426,#101427,#101428,#101429,
#101430,#101431,#101432,#101433,#101434),.UNSPECIFIED.,.F.,.F.,(4,3,3,3,
3,3,3,3,3,3,3,3,3,3,3,3,3,3,3,3,3,3,3,3,3,3,3,3,3,3,3,3,3,3,3,3,3,3,3,3,
3,3,3,3,3,3,3,3,3,3,3,3,3,3,3,3,3,3,3,3,4),(0.0187002242979963,0.0189846710771926,
0.0192766768141431,0.01934682847914,0.0196838394086382,0.0199934326602836,
0.0200088365092078,0.0211598636679579,0.021286641022571,0.0213183403852421,
0.0219730079604549,0.0225798493848584,0.0226270459403006,0.0237548263912282,
0.0238730577471458,0.0239321804060318,0.0248848375890449,0.0251662661094332,
0.0252323362288836,0.0258128702905769,0.0258800535176497,0.0263231529799011,
0.0264594744717206,0.0265261910961018,0.0271926230304998,0.0277526828340081,
0.0278136196686285,0.0283474366902465,0.0288971381406126,0.0290458911962956,
0.0290951190771367,0.0297446067327393,0.0303390995585831,0.0303729190324874,
0.0306881476849833,0.0309857037397268,0.0313980451165654,0.0316323079208706,
0.0316493951147151,0.0322789121020143,0.0322880973836838,0.0328405965385594,
0.0329255162831581,0.0329273016035652,0.0340932297430462,0.034209139758673,
0.0342187246454456,0.0345492922426382,0.0348653288265893,0.0351986616609935,
0.0354959079175446,0.035511933007733,0.0365799882698762,0.0367886773665346,
0.0368051413700205,0.0374373369862022,0.0374517455511642,0.0380873647343798,
0.0380983497323079,0.0391442500642898,0.0393915580945953),.UNSPECIFIED.);
#2328=B_SPLINE_CURVE_WITH_KNOTS('',3,(#101618,#101619,#101620,#101621,#101622,
#101623,#101624,#101625,#101626,#101627,#101628,#101629,#101630,#101631,
#101632,#101633,#101634,#101635,#101636,#101637,#101638,#101639,#101640,
#101641,#101642,#101643,#101644,#101645,#101646,#101647,#101648,#101649,
#101650,#101651,#101652,#101653,#101654,#101655,#101656,#101657,#101658,
#101659,#101660,#101661,#101662,#101663,#101664,#101665,#101666,#101667,
#101668,#101669,#101670,#101671,#101672,#101673,#101674,#101675,#101676,
#101677,#101678,#101679,#101680,#101681,#101682,#101683,#101684,#101685,
#101686,#101687,#101688,#101689,#101690,#101691,#101692,#101693,#101694,
#101695,#101696,#101697,#101698,#101699,#101700,#101701,#101702,#101703,
#101704,#101705,#101706,#101707,#101708,#101709,#101710,#101711,#101712,
#101713,#101714,#101715,#101716,#101717,#101718,#101719,#101720,#101721,
#101722,#101723,#101724,#101725,#101726,#101727,#101728,#101729,#101730,
#101731,#101732,#101733,#101734,#101735,#101736,#101737,#101738,#101739,
#101740,#101741,#101742,#101743,#101744,#101745,#101746,#101747,#101748,
#101749,#101750,#101751,#101752,#101753,#101754,#101755,#101756,#101757,
#101758,#101759,#101760,#101761,#101762,#101763,#101764,#101765,#101766,
#101767,#101768,#101769,#101770,#101771,#101772,#101773,#101774,#101775,
#101776,#101777,#101778,#101779,#101780,#101781,#101782,#101783,#101784,
#101785,#101786,#101787,#101788,#101789,#101790,#101791,#101792),
 .UNSPECIFIED.,.F.,.F.,(4,3,3,3,3,3,3,3,3,3,3,3,3,3,3,3,3,3,3,3,3,3,3,3,
3,3,3,3,3,3,3,3,3,3,3,3,3,3,3,3,3,3,3,3,3,3,3,3,3,3,3,3,3,3,3,3,3,3,4),
(0.,7.00136229228461E-5,0.000880271419196672,0.00197980055185577,0.00250406869828298,
0.00300266268960072,0.00331712911283045,0.00413059578319974,0.00532772256794858,
0.0057574742158991,0.00600532537920143,0.00738304200408561,0.00900794430850162,
0.00900798806880215,0.0112899391783712,0.0120106507584029,0.0122570346230108,
0.0135119821032032,0.0138815868497288,0.0147250110537092,0.0150133134480036,
0.0155067088258865,0.016845214616771,0.0180159761376041,0.0187586550708964,
0.0195173074824044,0.0203855296680284,0.0210186388272047,0.0220135800001955,
0.0236425023713017,0.0240213015168053,0.0244570699511879,0.0252717472664166,
0.0255226328616056,0.0270239642064059,0.0285252955512062,0.0285300848199135,
0.0293428874314582,0.0300266268960065,0.0301588925271162,0.0313458910919184,
0.031787155165216,0.033029289585607,0.0334140923804464,0.0345306209304072,
0.0350404780787163,0.0360319522752075,0.0366663282699641,0.0375332836200077,
0.0382915981957545,0.039034614964808,0.0412861444660561,0.041540518345781,
0.0420372776544085,0.0431651404778179,0.0447901356468785,0.045039940344009,
0.0470573761227504,0.0480426030336095),.UNSPECIFIED.);
#2329=B_SPLINE_CURVE_WITH_KNOTS('',3,(#101794,#101795,#101796,#101797,#101798,
#101799,#101800,#101801),.UNSPECIFIED.,.F.,.F.,(4,2,2,4),(0.100097362857501,
0.102091718402555,0.103088896175082,0.104086073947609),.UNSPECIFIED.);
#2330=B_SPLINE_CURVE_WITH_KNOTS('',3,(#101961,#101962,#101963,#101964,#101965,
#101966,#101967,#101968,#101969,#101970,#101971,#101972,#101973,#101974,
#101975,#101976,#101977,#101978,#101979,#101980,#101981,#101982,#101983,
#101984,#101985,#101986,#101987,#101988,#101989,#101990,#101991,#101992,
#101993,#101994,#101995,#101996,#101997,#101998,#101999,#102000,#102001,
#102002,#102003,#102004,#102005,#102006,#102007,#102008,#102009,#102010,
#102011,#102012,#102013,#102014,#102015,#102016,#102017,#102018,#102019,
#102020,#102021,#102022,#102023,#102024,#102025,#102026,#102027,#102028,
#102029,#102030,#102031,#102032,#102033,#102034,#102035,#102036,#102037,
#102038,#102039,#102040,#102041,#102042,#102043,#102044,#102045,#102046,
#102047,#102048,#102049,#102050,#102051,#102052,#102053,#102054,#102055,
#102056,#102057,#102058,#102059,#102060,#102061,#102062,#102063,#102064,
#102065,#102066,#102067,#102068,#102069,#102070,#102071,#102072,#102073,
#102074,#102075,#102076,#102077,#102078,#102079,#102080,#102081,#102082,
#102083,#102084,#102085,#102086,#102087,#102088,#102089,#102090,#102091,
#102092,#102093,#102094,#102095,#102096,#102097,#102098,#102099,#102100,
#102101,#102102,#102103,#102104,#102105,#102106,#102107,#102108,#102109,
#102110,#102111,#102112,#102113,#102114,#102115,#102116,#102117,#102118,
#102119,#102120,#102121,#102122,#102123,#102124,#102125,#102126,#102127,
#102128,#102129,#102130,#102131,#102132,#102133,#102134,#102135,#102136,
#102137,#102138,#102139,#102140,#102141,#102142,#102143,#102144,#102145,
#102146,#102147,#102148,#102149,#102150,#102151,#102152,#102153,#102154,
#102155,#102156,#102157,#102158,#102159,#102160,#102161,#102162,#102163,
#102164,#102165,#102166,#102167,#102168,#102169,#102170,#102171,#102172,
#102173,#102174,#102175,#102176,#102177,#102178,#102179,#102180,#102181,
#102182,#102183),.UNSPECIFIED.,.F.,.F.,(4,3,3,3,3,3,3,3,3,3,3,3,3,3,3,3,
3,3,3,3,3,3,3,3,3,3,3,3,3,3,3,3,3,3,3,3,3,3,3,3,3,3,3,3,3,3,3,3,3,3,3,3,
3,3,3,3,3,3,3,3,3,3,3,3,3,3,3,3,3,3,3,3,3,3,4),(0.0536197899396224,0.0552276244004006,
0.0552355709876449,0.0564636360413837,0.056836730186764,0.0568513520356673,
0.0585010989846075,0.0600604289236084,0.0600829141317123,0.0616747375677009,
0.0616986951797348,0.0631694062564402,0.0632905117196437,0.0633144762277572,
0.0653332916274416,0.0665264501713466,0.0665460383238021,0.0680226211568013,
0.0681465613676236,0.0681618193718244,0.0697679763088799,0.0697776004198467,
0.0713906714255839,0.0713933814678691,0.0730091625158914,0.0730146093723318,
0.0752607556604403,0.0762407246119361,0.0762648548190898,0.0777231476585592,
0.0778565056599585,0.0778906973850273,0.0791924472928067,0.0794722867079808,
0.0795162256569394,0.0810880677560031,0.0811414459847621,0.0823878645714303,
0.0827038488040255,0.082765970222281,0.0844200933214862,0.0859354109000701,
0.0860114915248442,0.0868961672850943,0.0875511919480923,0.0887466775684487,
0.0891669729961145,0.0892519026800103,0.0907827540441368,0.090869989342466,
0.0922381233782822,0.092398535092159,0.0924866314778507,0.0942502320947376,
0.0956300971882036,0.0957154955381666,0.0971616980126198,0.0972458782362259,
0.097327446100537,0.0983010085687495,0.0988616592842482,0.0989376222126474,
0.0999829246184123,0.10047744033227,0.100546243852972,0.101152494922671,
0.101724341209343,0.102093221380293,0.102150357244739,0.102702522250806,
0.102901111904304,0.103522312960998,0.103709002428315,0.104937728080333,
0.105324783476337),.UNSPECIFIED.);
#2331=B_SPLINE_CURVE_WITH_KNOTS('',3,(#102187,#102188,#102189,#102190,#102191,
#102192,#102193,#102194,#102195,#102196,#102197,#102198,#102199,#102200,
#102201,#102202,#102203,#102204,#102205,#102206,#102207,#102208,#102209,
#102210,#102211,#102212,#102213,#102214,#102215,#102216,#102217,#102218,
#102219,#102220,#102221,#102222,#102223,#102224,#102225,#102226,#102227,
#102228,#102229,#102230,#102231,#102232,#102233,#102234,#102235,#102236,
#102237,#102238,#102239,#102240),.UNSPECIFIED.,.F.,.F.,(4,2,2,2,2,2,2,2,
2,2,2,2,2,2,2,2,2,2,2,2,2,2,2,2,2,2,4),(0.,0.00156341081501294,0.00312682163002588,
0.00469023244503882,0.00625364326005176,0.00938046489007764,0.0109438757050905,
0.0125072865201034,0.0156341081501293,0.0171975189651422,0.0187609297801551,
0.021887751410181,0.0226694568176875,0.023451162225194,0.0250145730402071,
0.0265779838552202,0.0281413946702332,0.0312682163002594,0.0328316271152726,
0.0343950379302857,0.037521859560312,0.0406486811903383,0.0422120920053514,
0.0437755028203645,0.0469023244503908,0.0484657352654039,0.050029146080417),
 .UNSPECIFIED.);
#2332=B_SPLINE_CURVE_WITH_KNOTS('',3,(#102242,#102243,#102244,#102245,#102246,
#102247,#102248,#102249,#102250,#102251),.UNSPECIFIED.,.F.,.F.,(4,3,3,4),
(0.101994009991496,0.102941137438368,0.1034279046247,0.103888264885239),
 .UNSPECIFIED.);
#2333=B_SPLINE_CURVE_WITH_KNOTS('',3,(#102405,#102406,#102407,#102408,#102409,
#102410,#102411,#102412,#102413,#102414,#102415,#102416,#102417,#102418,
#102419,#102420,#102421,#102422,#102423,#102424,#102425,#102426,#102427,
#102428,#102429,#102430,#102431,#102432,#102433,#102434,#102435,#102436,
#102437,#102438,#102439,#102440,#102441,#102442,#102443,#102444,#102445,
#102446,#102447,#102448,#102449,#102450,#102451,#102452,#102453,#102454,
#102455,#102456,#102457,#102458,#102459,#102460,#102461,#102462,#102463,
#102464,#102465,#102466,#102467,#102468,#102469,#102470,#102471,#102472,
#102473,#102474,#102475,#102476,#102477,#102478,#102479,#102480,#102481,
#102482,#102483,#102484,#102485,#102486,#102487,#102488,#102489,#102490,
#102491,#102492,#102493,#102494,#102495,#102496,#102497,#102498,#102499,
#102500,#102501,#102502,#102503,#102504,#102505,#102506,#102507,#102508,
#102509,#102510,#102511,#102512,#102513,#102514,#102515,#102516,#102517,
#102518,#102519,#102520,#102521,#102522,#102523,#102524,#102525,#102526,
#102527,#102528,#102529,#102530,#102531,#102532,#102533,#102534,#102535,
#102536,#102537,#102538,#102539,#102540,#102541,#102542,#102543,#102544,
#102545,#102546,#102547,#102548,#102549,#102550,#102551,#102552,#102553,
#102554,#102555,#102556,#102557,#102558,#102559,#102560,#102561,#102562,
#102563,#102564,#102565,#102566,#102567,#102568,#102569,#102570,#102571,
#102572,#102573,#102574,#102575,#102576,#102577,#102578,#102579,#102580,
#102581,#102582,#102583,#102584,#102585,#102586,#102587,#102588,#102589,
#102590,#102591,#102592,#102593,#102594,#102595,#102596,#102597,#102598,
#102599,#102600,#102601,#102602,#102603),.UNSPECIFIED.,.F.,.F.,(4,3,3,3,
3,3,3,3,3,3,3,3,3,3,3,3,3,3,3,3,3,3,3,3,3,3,3,3,3,3,3,3,3,3,3,3,3,3,3,3,
3,3,3,3,3,3,3,3,3,3,3,3,3,3,3,3,3,3,3,3,3,3,3,3,3,3,4),(0.0415609574076441,
0.0419999079181986,0.0424456108255441,0.0428514400237989,0.0434891733075762,
0.0441269065913535,0.0441419226399537,0.0454112381061315,0.0454324052561084,
0.0465323604473209,0.0466965822688831,0.0467228878722632,0.0484820040281491,
0.0492715033675918,0.0493038531045728,0.050735911668559,0.0518516607057079,
0.0518848183368824,0.0535408116928349,0.0544369446773842,0.054465783569192,
0.0555110612923409,0.0557314168323167,0.0557562661853469,0.0570268987744937,
0.0570467488015017,0.0580899941196728,0.0583234009749456,0.0583372314176566,
0.0593028016534022,0.0596206777396424,0.0596277140338114,0.0622086792661211,
0.0622163187211141,0.063499161882276,0.0635142754825525,0.0647896444984309,
0.0648116296745799,0.0660801271145858,0.0661083966471777,0.0673706097307407,
0.0674045134523431,0.0688635319844597,0.0699515749630503,0.0699933139595394,
0.0712420575792051,0.0712859635838356,0.0722808578696521,0.0725325401953599,
0.0725774037566074,0.0740349703455224,0.0751135054276695,0.0751563211290189,
0.0761837854504818,0.0764039880438243,0.0764437283836802,0.0775804812596956,
0.0776944706599792,0.0777298862469096,0.078984953276134,0.0790147568862244,
0.0801773798800301,0.0802754358922888,0.0802979121042526,0.0811942832430378,
0.0820670967544178,0.0828564011245984),.UNSPECIFIED.);
#2334=B_SPLINE_CURVE_WITH_KNOTS('',3,(#102607,#102608,#102609,#102610,#102611,
#102612,#102613,#102614,#102615,#102616,#102617,#102618,#102619,#102620,
#102621,#102622,#102623,#102624,#102625,#102626,#102627,#102628,#102629,
#102630,#102631,#102632,#102633,#102634,#102635,#102636,#102637,#102638,
#102639,#102640,#102641,#102642,#102643,#102644,#102645,#102646,#102647,
#102648,#102649,#102650,#102651,#102652,#102653,#102654,#102655,#102656,
#102657,#102658,#102659,#102660,#102661,#102662,#102663,#102664,#102665,
#102666,#102667,#102668,#102669,#102670,#102671,#102672,#102673,#102674,
#102675,#102676,#102677,#102678,#102679,#102680,#102681,#102682,#102683,
#102684,#102685,#102686,#102687,#102688,#102689,#102690,#102691,#102692,
#102693,#102694,#102695,#102696,#102697,#102698,#102699,#102700,#102701,
#102702,#102703,#102704,#102705,#102706,#102707,#102708,#102709,#102710,
#102711,#102712,#102713,#102714,#102715,#102716,#102717,#102718,#102719,
#102720,#102721,#102722,#102723,#102724,#102725,#102726,#102727,#102728,
#102729,#102730,#102731,#102732,#102733,#102734,#102735,#102736,#102737,
#102738,#102739,#102740,#102741,#102742,#102743,#102744,#102745,#102746,
#102747,#102748,#102749,#102750,#102751,#102752,#102753,#102754,#102755,
#102756,#102757,#102758,#102759,#102760,#102761,#102762,#102763,#102764,
#102765,#102766,#102767,#102768,#102769,#102770,#102771,#102772,#102773,
#102774,#102775,#102776,#102777,#102778,#102779,#102780,#102781,#102782,
#102783,#102784,#102785,#102786,#102787,#102788,#102789,#102790,#102791,
#102792,#102793,#102794,#102795,#102796,#102797,#102798,#102799,#102800,
#102801,#102802,#102803,#102804,#102805,#102806,#102807,#102808,#102809,
#102810,#102811,#102812,#102813,#102814,#102815,#102816,#102817,#102818,
#102819,#102820),.UNSPECIFIED.,.F.,.F.,(4,3,3,3,3,3,3,3,3,3,3,3,3,3,3,3,
3,3,3,3,3,3,3,3,3,3,3,3,3,3,3,3,3,3,3,3,3,3,3,3,3,3,3,3,3,3,3,3,3,3,3,3,
3,3,3,3,3,3,3,3,3,3,3,3,3,3,3,3,3,3,3,4),(0.,0.000919480979116562,0.00186665391132835,
0.00222303890370072,0.00246023501007185,0.00308006741789906,0.00345996891983423,
0.00369035251510777,0.00469778641362987,0.00492047002014368,0.00577875096523307,
0.00593619564291911,0.0061505875251796,0.00691217011921717,0.00717505541494648,
0.00738070503021552,0.00841742521903872,0.00946182449544707,0.00965322408999174,
0.00984094004028725,0.010527196801318,0.0108924604402717,0.0110710575453231,
0.0121313588744037,0.012301175050359,0.0135614282722574,0.014608084951402,
0.0147614100604307,0.0155427428164244,0.0158457881834858,0.0159915275654665,
0.0170831200839182,0.0172216450705023,0.0180163683085078,0.0183201098374356,
0.0184517625755382,0.0191739816007739,0.0195568018131331,0.019681880080574,
0.0208560722381215,0.022030264395669,0.0221421150906457,0.0229078739325012,
0.0232673524625759,0.0233722325956815,0.0245048134750371,0.0246023501007174,
0.0254360756729617,0.0257427490373535,0.0258324676057532,0.026634352472116,
0.0269811460780054,0.027062585110789,0.028478718853076,0.0294588729843419,
0.0295228201208608,0.0310014861472409,0.0319371442892162,0.0319830551309325,
0.0335148785822243,0.0344145418676412,0.0344432901410042,0.0353749506243358,
0.0356525636344977,0.0356734076460401,0.0368901184213511,0.036903525151076,
0.0375185839035939,0.0381336426561119,0.0385671407304433,0.0389938437394035,
0.0393637601611478),.UNSPECIFIED.);
#2335=B_SPLINE_CURVE_WITH_KNOTS('',3,(#102826,#102827,#102828,#102829,#102830,
#102831,#102832,#102833,#102834,#102835,#102836,#102837,#102838,#102839,
#102840,#102841,#102842,#102843,#102844,#102845,#102846,#102847,#102848,
#102849,#102850,#102851,#102852,#102853,#102854,#102855,#102856,#102857,
#102858,#102859,#102860,#102861,#102862,#102863,#102864,#102865,#102866,
#102867,#102868,#102869,#102870,#102871,#102872,#102873,#102874,#102875),
 .UNSPECIFIED.,.T.,.F.,(4,2,2,2,2,2,2,2,2,2,2,2,2,2,2,2,2,2,2,2,2,2,2,2,
4),(-7.68142619696719,-7.4403709942257,-7.19931579148422,-6.71720538600124,
-6.23913751686332,-6.00010358229436,-5.7610696477254,-5.52203571315644,
-5.28300177858748,-4.80493390944956,-4.32282350396658,-4.08176830122509,
-3.8407130984836,-3.59965789574211,-3.35860269300062,-2.87649228751764,
-2.39842441837972,-2.15939048381076,-1.9203565492418,-1.68132261467284,
-1.44228868010388,-0.964220810965958,-0.482110405482979,-0.24105520274149,
0.),.UNSPECIFIED.);
#2336=B_SPLINE_CURVE_WITH_KNOTS('',3,(#102878,#102879,#102880,#102881,#102882,
#102883,#102884,#102885,#102886,#102887,#102888,#102889,#102890,#102891,
#102892,#102893,#102894,#102895,#102896,#102897,#102898,#102899,#102900,
#102901,#102902,#102903,#102904,#102905,#102906,#102907,#102908,#102909,
#102910,#102911,#102912,#102913,#102914,#102915,#102916,#102917,#102918,
#102919,#102920,#102921,#102922,#102923,#102924,#102925,#102926,#102927,
#102928,#102929),.UNSPECIFIED.,.F.,.F.,(4,2,2,2,2,2,2,2,2,2,2,2,2,2,2,2,
2,2,2,2,2,2,2,2,2,4),(0.0396248818917468,0.0420848252462546,0.0433147969235084,
0.0445447686007623,0.0457747402780162,0.04700471195527,0.0494646553097779,
0.0506946269870318,0.0519245986642857,0.0543845420187934,0.0556145136960473,
0.0568444853733012,0.059304428727809,0.0605344004050629,0.0617643720823168,
0.0629943437595707,0.0642243154368246,0.0666842587913323,0.0679142304685862,
0.0691442021458401,0.0703741738230939,0.0716041455003478,0.0740640888548556,
0.0752940605321094,0.0765240322093633,0.078983975563871),.UNSPECIFIED.);
#2337=B_SPLINE_CURVE_WITH_KNOTS('',3,(#102933,#102934,#102935,#102936,#102937,
#102938,#102939,#102940,#102941,#102942,#102943,#102944,#102945,#102946,
#102947,#102948,#102949,#102950,#102951,#102952,#102953,#102954,#102955,
#102956,#102957),.UNSPECIFIED.,.F.,.F.,(4,3,3,3,3,3,3,3,4),(0.050029146080417,
0.0504604958563081,0.0505100567684285,0.0509435518624711,0.05099096745644,
0.0514718781444515,0.0516554513507709,0.0517123334884572,0.0519527888232233),
 .UNSPECIFIED.);
#2338=B_SPLINE_CURVE_WITH_KNOTS('',3,(#102960,#102961,#102962,#102963,#102964,
#102965,#102966,#102967,#102968,#102969,#102970,#102971,#102972,#102973,
#102974,#102975,#102976,#102977,#102978,#102979,#102980,#102981,#102982,
#102983,#102984,#102985,#102986,#102987,#102988,#102989,#102990,#102991,
#102992,#102993,#102994,#102995,#102996,#102997,#102998,#102999,#103000,
#103001,#103002,#103003,#103004,#103005,#103006,#103007,#103008,#103009),
 .UNSPECIFIED.,.F.,.F.,(4,2,2,2,2,2,2,2,2,2,2,2,2,2,2,2,2,2,2,2,2,2,2,2,
4),(0.0520590732062046,0.0550614663094106,0.0558120645852121,0.0565626628610136,
0.0580638594126165,0.0595650559642194,0.0610662525158222,0.0640686456190281,
0.0655698421706312,0.0670710387222342,0.0700734318254404,0.0715746283770435,
0.0730758249286466,0.0760782180318527,0.0775794145834557,0.0790806111350588,
0.0805818076866618,0.0820830042382649,0.0850853973414709,0.0880877904446769,
0.0910901835478829,0.094092576651089,0.095593773202692,0.097094969754295,
0.100097362857501),.UNSPECIFIED.);
#2339=B_SPLINE_CURVE_WITH_KNOTS('',3,(#103010,#103011,#103012,#103013,#103014,
#103015,#103016,#103017,#103018,#103019),.UNSPECIFIED.,.F.,.F.,(4,2,2,2,
4),(0.0480426030336095,0.0490467205767583,0.050050838119907,0.0510549556630558,
0.0520590732062046),.UNSPECIFIED.);
#2340=B_SPLINE_CURVE_WITH_KNOTS('',3,(#103020,#103021,#103022,#103023,#103024,
#103025,#103026,#103027,#103028,#103029,#103030,#103031,#103032,#103033,
#103034,#103035,#103036,#103037,#103038,#103039,#103040,#103041,#103042,
#103043,#103044,#103045,#103046,#103047,#103048,#103049,#103050,#103051,
#103052,#103053,#103054,#103055,#103056,#103057,#103058,#103059,#103060,
#103061,#103062,#103063,#103064,#103065,#103066,#103067,#103068,#103069,
#103070,#103071,#103072,#103073,#103074,#103075,#103076,#103077,#103078,
#103079,#103080,#103081,#103082,#103083,#103084,#103085,#103086,#103087,
#103088,#103089,#103090,#103091,#103092,#103093,#103094,#103095,#103096,
#103097,#103098,#103099,#103100,#103101,#103102,#103103,#103104,#103105,
#103106,#103107,#103108,#103109,#103110,#103111,#103112,#103113,#103114,
#103115,#103116,#103117,#103118,#103119,#103120,#103121,#103122,#103123,
#103124,#103125,#103126,#103127,#103128,#103129,#103130,#103131,#103132,
#103133,#103134,#103135,#103136,#103137,#103138,#103139,#103140,#103141,
#103142,#103143,#103144,#103145,#103146,#103147,#103148,#103149,#103150,
#103151,#103152,#103153,#103154,#103155,#103156,#103157,#103158,#103159,
#103160,#103161,#103162,#103163,#103164,#103165,#103166,#103167,#103168,
#103169,#103170,#103171,#103172,#103173,#103174,#103175,#103176,#103177,
#103178,#103179,#103180,#103181,#103182,#103183,#103184,#103185,#103186,
#103187,#103188,#103189,#103190,#103191,#103192,#103193,#103194,#103195,
#103196,#103197,#103198,#103199,#103200,#103201,#103202,#103203,#103204,
#103205,#103206,#103207,#103208,#103209,#103210,#103211,#103212,#103213,
#103214,#103215,#103216,#103217,#103218,#103219,#103220,#103221,#103222,
#103223,#103224),.UNSPECIFIED.,.F.,.F.,(4,3,3,3,3,3,3,3,3,3,3,3,3,3,3,3,
3,3,3,3,3,3,3,3,3,3,3,3,3,3,3,3,3,3,3,3,3,3,3,3,3,3,3,3,3,3,3,3,3,3,3,3,
3,3,3,3,3,3,3,3,3,3,3,3,3,3,3,3,4),(0.051952788832463,0.0523437358727679,
0.0530396348010499,0.0532815940436916,0.0535165769936827,0.0550803651549024,
0.0565315459304904,0.0566441533161221,0.0573435791058262,0.0581553062489572,
0.0582079414773418,0.0597781972481066,0.0613355177997813,0.0614004919138027,
0.0627595431987245,0.0628993059610011,0.0630224461823624,0.0644630941222208,
0.066266557277031,0.0675906704446604,0.0678890579253495,0.0688036127964717,
0.0691544586058802,0.0695121857757964,0.0705623247811663,0.0707182467671,
0.0722820349283198,0.0727603963114585,0.0735729358548261,0.0738458230895395,
0.0743855823551034,0.0760111644019604,0.0769733994119791,0.0775954188216906,
0.0776371348320698,0.077755293492589,0.0783329590757904,0.0784502993253913,
0.078537187573199,0.079263366729678,0.0801009757344188,0.0816647638956387,
0.0825143971297319,0.0832285520568585,0.0853698372315117,0.0857634780397394,
0.0863561283792982,0.0870860429658589,0.087387128745137,0.087919916540518,
0.0890096229688163,0.0894837047017378,0.0904433744732693,0.0906319233369378,
0.0910474928629577,0.0918522904268146,0.0922540308854937,0.0926112810241775,
0.0947257451253502,0.0954981621844028,0.095738857346617,0.0966800930537847,
0.0971208482525778,0.0973026455078367,0.098172856385979,0.0987443411160432,
0.0988664336690564,0.100855253343851,0.101994009991496),.UNSPECIFIED.);
#2341=B_SPLINE_CURVE_WITH_KNOTS('',3,(#103281,#103282,#103283,#103284,#103285,
#103286,#103287,#103288,#103289,#103290,#103291,#103292,#103293,#103294,
#103295,#103296,#103297,#103298,#103299,#103300,#103301,#103302,#103303,
#103304,#103305),.UNSPECIFIED.,.F.,.F.,(4,3,3,3,3,3,3,3,4),(3.14159265358979,
3.53429173528852,3.92699081698724,4.31968989868597,4.71238898038469,5.10508806208341,
5.49778714378214,5.89048622548086,6.28318530717959),.UNSPECIFIED.);
#2342=B_SPLINE_CURVE_WITH_KNOTS('',3,(#103330,#103331,#103332,#103333,#103334,
#103335,#103336,#103337,#103338,#103339,#103340,#103341,#103342,#103343,
#103344,#103345,#103346,#103347,#103348,#103349,#103350,#103351,#103352,
#103353,#103354,#103355,#103356,#103357,#103358,#103359,#103360,#103361,
#103362,#103363,#103364,#103365,#103366,#103367,#103368,#103369,#103370,
#103371,#103372,#103373,#103374,#103375,#103376,#103377,#103378,#103379,
#103380,#103381,#103382,#103383,#103384,#103385,#103386,#103387,#103388,
#103389,#103390,#103391,#103392,#103393,#103394,#103395,#103396,#103397,
#103398,#103399,#103400,#103401,#103402,#103403,#103404,#103405,#103406,
#103407,#103408,#103409,#103410,#103411,#103412,#103413,#103414,#103415,
#103416,#103417,#103418,#103419,#103420,#103421,#103422,#103423,#103424,
#103425,#103426,#103427,#103428,#103429,#103430,#103431,#103432,#103433,
#103434,#103435,#103436,#103437,#103438,#103439,#103440,#103441,#103442,
#103443,#103444,#103445,#103446,#103447,#103448,#103449,#103450,#103451,
#103452,#103453,#103454,#103455,#103456,#103457,#103458,#103459,#103460,
#103461,#103462,#103463,#103464,#103465,#103466,#103467,#103468,#103469,
#103470,#103471,#103472,#103473,#103474),.UNSPECIFIED.,.F.,.F.,(4,3,3,3,
3,3,3,3,3,3,3,3,3,3,3,3,3,3,3,3,3,3,3,3,3,3,3,3,3,3,3,3,3,3,3,3,3,3,3,3,
3,3,3,3,3,3,3,3,4),(0.00175934839635171,0.00264937165101398,0.00281190034136253,
0.0029216913114692,0.00345298327300805,0.00350284378635125,0.00386445228637335,
0.00408494443402798,0.0045643909026228,0.0050528930166323,0.00525444258302874,
0.00573754835263548,0.00596955617639502,0.00642216793328342,0.00688988455817184,
0.00702210812140589,0.00759015068768004,0.00807466006641675,0.00817328490518593,
0.00875592930808911,0.00912721201142762,0.00950595668589702,0.00965348798393305,
0.0099194404906703,0.0101797639564385,0.0106406398760054,0.0110804857260411,
0.0112323159014494,0.0116411351505613,0.0120566663811269,0.0122406856381238,
0.0122848678464602,0.0133374197914711,0.013400690819128,0.0139807325781765,
0.014389971736482,0.014560858934484,0.0150704291285518,0.0154425236814929,
0.015721211993778,0.0159687996539983,0.0164950756265037,0.0168813629537642,
0.0174094393522003,0.0174613379315374,0.0175476275715146,0.0180410999382036,
0.0185583303726384,0.0186001795165254),.UNSPECIFIED.);
#2343=B_SPLINE_CURVE_WITH_KNOTS('',3,(#103494,#103495,#103496,#103497,#103498,
#103499),.UNSPECIFIED.,.F.,.F.,(4,2,4),(0.0186001795165254,0.0194806906344087,
0.0203612017522921),.UNSPECIFIED.);
#2344=B_SPLINE_CURVE_WITH_KNOTS('',3,(#103501,#103502,#103503,#103504,#103505,
#103506,#103507,#103508,#103509,#103510,#103511,#103512,#103513,#103514,
#103515,#103516,#103517,#103518,#103519,#103520,#103521,#103522,#103523,
#103524,#103525),.UNSPECIFIED.,.F.,.F.,(4,3,3,3,3,3,3,3,4),(0.,0.392699081698723,
0.785398163397448,1.17809724509617,1.5707963267949,1.96349540849362,2.35619449019234,
2.74889357189107,3.14159265358979),.UNSPECIFIED.);
#2345=B_SPLINE_CURVE_WITH_KNOTS('',3,(#103581,#103582,#103583,#103584,#103585,
#103586,#103587,#103588,#103589,#103590,#103591,#103592,#103593,#103594,
#103595,#103596,#103597,#103598,#103599,#103600,#103601,#103602,#103603,
#103604,#103605,#103606,#103607,#103608,#103609,#103610,#103611,#103612,
#103613,#103614,#103615,#103616,#103617,#103618,#103619,#103620,#103621,
#103622,#103623,#103624,#103625,#103626,#103627,#103628,#103629,#103630,
#103631,#103632,#103633,#103634,#103635,#103636,#103637,#103638,#103639,
#103640,#103641,#103642,#103643,#103644,#103645,#103646,#103647,#103648,
#103649,#103650,#103651,#103652,#103653,#103654,#103655,#103656,#103657,
#103658,#103659,#103660,#103661,#103662,#103663,#103664,#103665,#103666,
#103667,#103668,#103669,#103670,#103671,#103672,#103673,#103674,#103675,
#103676,#103677,#103678,#103679,#103680,#103681,#103682,#103683,#103684,
#103685,#103686,#103687,#103688,#103689,#103690,#103691,#103692,#103693,
#103694,#103695,#103696,#103697,#103698,#103699,#103700,#103701,#103702,
#103703,#103704,#103705,#103706,#103707,#103708,#103709,#103710,#103711,
#103712,#103713,#103714,#103715,#103716,#103717,#103718,#103719,#103720,
#103721,#103722,#103723,#103724,#103725,#103726,#103727,#103728,#103729,
#103730,#103731,#103732,#103733,#103734,#103735,#103736,#103737,#103738,
#103739,#103740,#103741,#103742,#103743,#103744,#103745,#103746,#103747,
#103748,#103749,#103750,#103751,#103752,#103753,#103754,#103755,#103756,
#103757,#103758,#103759,#103760,#103761,#103762,#103763,#103764,#103765,
#103766,#103767,#103768,#103769,#103770,#103771,#103772,#103773,#103774,
#103775,#103776,#103777,#103778,#103779,#103780,#103781,#103782,#103783,
#103784,#103785,#103786,#103787,#103788,#103789,#103790,#103791),
 .UNSPECIFIED.,.F.,.F.,(4,3,3,3,3,3,3,3,3,3,3,3,3,3,3,3,3,3,3,3,3,3,3,3,
3,3,3,3,3,3,3,3,3,3,3,3,3,3,3,3,3,3,3,3,3,3,3,3,3,3,3,3,3,3,3,3,3,3,3,3,
3,3,3,3,3,3,3,3,3,3,4),(0.040185803323384,0.0413856421772186,0.0414967660328816,
0.0415142729908562,0.0422433040571364,0.0428064492703943,0.0428427426583284,
0.0441360070801344,0.0454292715019403,0.0454996819932728,0.0464712818980196,
0.0467431693953829,0.046828151660745,0.0477888706112027,0.0480601760161093,
0.0481566213282172,0.0494297557376454,0.0505688592524304,0.0507028901470736,
0.0508135606631617,0.05208542808009,0.0533572954970183,0.0534704999981061,
0.0543381547764814,0.0546885729894539,0.0547989696655784,0.0560224031717165,
0.0561274393330507,0.0570603085182229,0.0579546885749173,0.0586976832404988,
0.0587843786679952,0.0596803976577506,0.0605641633514876,0.0613811379148684,
0.0614413180029398,0.0626283973946032,0.0627251289020388,0.062769787670412,
0.0640695304066911,0.0640982573378843,0.0654135246131901,0.0654267270053565,
0.06664916102305,0.0667551966728288,0.0667570806288456,0.0685560798819261,
0.0694121360077733,0.069439147524414,0.0705885834253151,0.0707406056752456,
0.0707771747906088,0.0719257582233479,0.0720690753427178,0.072112636943896,
0.0733975450101901,0.0734454921936495,0.0745326321982652,0.0747260146776624,
0.0747757157272833,0.0763275630104522,0.0773829540126069,0.0774278153549588,
0.0787114236800792,0.0787493996324898,0.0798784815282868,0.0800398933475515,
0.0800679872775242,0.0812906359372778,0.0824788066968498,0.0826968326824961),
 .UNSPECIFIED.);
#2346=B_SPLINE_CURVE_WITH_KNOTS('',3,(#103793,#103794,#103795,#103796,#103797,
#103798,#103799,#103800,#103801,#103802,#103803,#103804,#103805,#103806,
#103807,#103808,#103809,#103810,#103811,#103812,#103813,#103814,#103815,
#103816,#103817,#103818,#103819,#103820,#103821,#103822,#103823,#103824,
#103825,#103826,#103827,#103828,#103829,#103830,#103831,#103832,#103833,
#103834,#103835,#103836,#103837,#103838,#103839,#103840,#103841,#103842,
#103843,#103844,#103845,#103846,#103847,#103848,#103849,#103850,#103851,
#103852,#103853,#103854,#103855,#103856,#103857,#103858,#103859,#103860,
#103861,#103862,#103863,#103864,#103865,#103866,#103867,#103868,#103869,
#103870,#103871,#103872,#103873,#103874,#103875,#103876,#103877,#103878,
#103879,#103880,#103881,#103882,#103883,#103884,#103885,#103886,#103887,
#103888,#103889,#103890,#103891,#103892,#103893,#103894,#103895,#103896,
#103897,#103898,#103899,#103900,#103901,#103902,#103903,#103904,#103905,
#103906,#103907,#103908,#103909,#103910,#103911,#103912,#103913,#103914,
#103915,#103916,#103917,#103918,#103919,#103920,#103921,#103922,#103923,
#103924,#103925,#103926,#103927,#103928,#103929,#103930,#103931,#103932,
#103933,#103934,#103935,#103936,#103937,#103938,#103939,#103940,#103941,
#103942,#103943,#103944,#103945,#103946,#103947,#103948,#103949,#103950,
#103951,#103952,#103953,#103954,#103955,#103956,#103957,#103958,#103959,
#103960,#103961,#103962,#103963,#103964,#103965,#103966,#103967,#103968,
#103969,#103970,#103971,#103972,#103973,#103974,#103975,#103976,#103977,
#103978,#103979,#103980,#103981,#103982,#103983,#103984,#103985,#103986,
#103987,#103988,#103989,#103990,#103991,#103992,#103993,#103994,#103995,
#103996,#103997,#103998,#103999,#104000),.UNSPECIFIED.,.F.,.F.,(4,3,3,3,
3,3,3,3,3,3,3,3,3,3,3,3,3,3,3,3,3,3,3,3,3,3,3,3,3,3,3,3,3,3,3,3,3,3,3,3,
3,3,3,3,3,3,3,3,3,3,3,3,3,3,3,3,3,3,3,3,3,3,3,3,3,3,3,3,3,4),(0.00187081090387685,
0.00271260435667731,0.00362268902859222,0.00470889615954381,0.0051051220936109,
0.00599081910916758,0.00672227768847788,0.00778276880661964,0.00833943328334486,
0.00942599481829403,0.0104998696456864,0.0115737444730788,0.0123823222705124,
0.0131909000679459,0.0142060282593073,0.014808055662813,0.01570812992925,
0.0164252112576801,0.0170970893496278,0.0177619833705879,0.0180423668525471,
0.0190026734096154,0.019950368561138,0.0208795972594237,0.0212766780422811,
0.0222765344942613,0.0232692933815865,0.0242499722556784,0.0245109892320151,
0.0253195670294486,0.025748847290095,0.0261281448268821,0.0270598184241075,
0.027745300421749,0.0287399757306573,0.029362456016616,0.0299897241643628,
0.0306190954857662,0.030979611611483,0.0318533830950452,0.032738324644238,
0.0336403396115833,0.034213922801217,0.0352558542716105,0.035831078396084,
0.0367181867272328,0.0374482339909511,0.038496060625361,0.0395893029030231,
0.0406825451806851,0.0413774134031154,0.0420918307001871,0.0422997007755522,
0.0433943605093511,0.0439168563704194,0.0450236020511531,0.0455340119652865,
0.04634258976272,0.0470220692265429,0.0471511675601536,0.048029000435268,
0.0488603746190341,0.0496350381747758,0.050385478749888,0.0511032328730903,
0.0517960284135848,0.0520026343447552,0.0527090367424346,0.0534533603415312,
0.0536197899396224),.UNSPECIFIED.);
#2347=B_SPLINE_CURVE_WITH_KNOTS('',3,(#104001,#104002,#104003,#104004,#104005,
#104006,#104007,#104008,#104009,#104010,#104011,#104012,#104013,#104014,
#104015,#104016,#104017,#104018,#104019,#104020,#104021,#104022,#104023,
#104024,#104025,#104026,#104027,#104028,#104029,#104030,#104031,#104032,
#104033,#104034,#104035,#104036,#104037,#104038,#104039,#104040,#104041,
#104042,#104043,#104044,#104045,#104046,#104047,#104048,#104049,#104050,
#104051,#104052),.UNSPECIFIED.,.F.,.F.,(4,2,2,2,2,2,2,2,2,2,2,2,2,2,2,2,
2,2,2,2,2,2,2,2,2,4),(0.000252666121810611,0.00283443432717517,0.00412531842985747,
0.00541620253253977,0.00799797073790439,0.00928885484058674,0.0105797389432691,
0.0118706230459514,0.0131615071486338,0.0157432753539985,0.0170341594566808,
0.018325043559363,0.0196159276620453,0.0209068117647276,0.0234885799700922,
0.0247794640727745,0.0260703481754568,0.0286521163808214,0.0299430004835037,
0.031233884586186,0.0338156527915506,0.0363974209969151,0.0376883050995973,
0.0389791892022796,0.0402700733049619,0.0415609574076441),.UNSPECIFIED.);
#2348=B_SPLINE_CURVE_WITH_KNOTS('',3,(#104846,#104847,#104848,#104849,#104850,
#104851,#104852,#104853,#104854,#104855,#104856,#104857,#104858,#104859,
#104860,#104861,#104862,#104863,#104864,#104865,#104866,#104867,#104868,
#104869,#104870,#104871,#104872,#104873,#104874,#104875,#104876,#104877,
#104878,#104879,#104880,#104881,#104882,#104883,#104884,#104885,#104886,
#104887,#104888,#104889,#104890,#104891,#104892,#104893,#104894,#104895,
#104896,#104897,#104898,#104899,#104900,#104901,#104902,#104903,#104904,
#104905,#104906,#104907,#104908,#104909,#104910,#104911,#104912,#104913,
#104914,#104915,#104916,#104917,#104918,#104919,#104920,#104921,#104922,
#104923,#104924,#104925,#104926,#104927,#104928,#104929,#104930,#104931,
#104932,#104933,#104934,#104935,#104936,#104937,#104938,#104939,#104940,
#104941,#104942,#104943,#104944,#104945,#104946,#104947,#104948,#104949,
#104950,#104951,#104952,#104953,#104954,#104955,#104956,#104957,#104958,
#104959,#104960,#104961,#104962,#104963,#104964,#104965,#104966,#104967,
#104968,#104969,#104970,#104971,#104972,#104973,#104974,#104975,#104976,
#104977,#104978,#104979,#104980,#104981,#104982,#104983,#104984,#104985,
#104986,#104987,#104988,#104989,#104990,#104991,#104992,#104993,#104994,
#104995,#104996,#104997,#104998,#104999,#105000,#105001,#105002,#105003,
#105004,#105005,#105006,#105007,#105008,#105009,#105010,#105011,#105012,
#105013,#105014,#105015,#105016,#105017,#105018,#105019,#105020,#105021,
#105022,#105023,#105024,#105025,#105026,#105027,#105028,#105029,#105030,
#105031,#105032,#105033,#105034,#105035,#105036,#105037,#105038,#105039,
#105040,#105041,#105042,#105043,#105044,#105045,#105046,#105047,#105048,
#105049,#105050,#105051,#105052,#105053,#105054,#105055,#105056),
 .UNSPECIFIED.,.F.,.F.,(4,3,3,3,3,3,3,3,3,3,3,3,3,3,3,3,3,3,3,3,3,3,3,3,
3,3,3,3,3,3,3,3,3,3,3,3,3,3,3,3,3,3,3,3,3,3,3,3,3,3,3,3,3,3,3,3,3,3,3,3,
3,3,3,3,3,3,3,3,3,3,4),(0.040185803323384,0.041385642177111,0.0414967660328816,
0.0415142729908562,0.0422433040571271,0.0428064492703943,0.0428427426583284,
0.0441360070801344,0.0454292715019403,0.0454996819932728,0.0464712818980038,
0.046743169395383,0.046828151660745,0.0477888706109921,0.0480601760161093,
0.0481566213282172,0.0494297557376455,0.050568859252351,0.0507028901470738,
0.0508135606631617,0.05208542808009,0.0533572954970184,0.0534704999981061,
0.0543381547765564,0.0546885729894539,0.0547989696655784,0.0560224031717167,
0.0561274393330507,0.0570603085182185,0.0579546885749104,0.0586976832404988,
0.0587843786679952,0.0596803976577581,0.0605641633515005,0.0613811379148684,
0.0614413180029398,0.062628397394844,0.0627251289020388,0.062769787670412,
0.0640695304066911,0.0640982573378843,0.0654135246131901,0.0654267270053565,
0.0666491610230946,0.0667551966728288,0.0667570806288456,0.0685560798820927,
0.0694121360077733,0.069439147524414,0.0705885834257307,0.0707406056752456,
0.0707771747906088,0.071925758222996,0.0720690753427178,0.072112636943896,
0.0733975450101901,0.0734454921936494,0.0745326321983655,0.0747260146776624,
0.0747757157272833,0.0763275630090201,0.0773829540126069,0.0774278153549589,
0.0787114236800792,0.0787493996324898,0.0798784815281566,0.0800398933475515,
0.0800679872775241,0.0812906359372127,0.0824788066966756,0.0826968326824961),
 .UNSPECIFIED.);
#2349=B_SPLINE_CURVE_WITH_KNOTS('',3,(#105185,#105186,#105187,#105188,#105189,
#105190,#105191,#105192,#105193,#105194,#105195,#105196,#105197,#105198,
#105199,#105200,#105201,#105202,#105203,#105204,#105205,#105206,#105207,
#105208,#105209,#105210,#105211,#105212,#105213,#105214,#105215,#105216,
#105217,#105218,#105219,#105220,#105221,#105222,#105223,#105224,#105225,
#105226,#105227,#105228,#105229,#105230,#105231,#105232,#105233,#105234,
#105235,#105236,#105237,#105238,#105239,#105240,#105241,#105242,#105243,
#105244,#105245,#105246,#105247,#105248,#105249,#105250,#105251,#105252,
#105253,#105254,#105255,#105256,#105257,#105258,#105259,#105260,#105261,
#105262,#105263,#105264,#105265,#105266,#105267,#105268,#105269,#105270,
#105271,#105272,#105273,#105274,#105275,#105276,#105277,#105278,#105279,
#105280,#105281,#105282,#105283,#105284,#105285,#105286,#105287,#105288,
#105289,#105290,#105291,#105292,#105293,#105294,#105295,#105296,#105297,
#105298,#105299,#105300,#105301,#105302,#105303,#105304,#105305,#105306,
#105307,#105308,#105309,#105310,#105311,#105312,#105313,#105314,#105315,
#105316,#105317,#105318,#105319,#105320,#105321,#105322,#105323,#105324,
#105325,#105326,#105327,#105328,#105329,#105330,#105331,#105332,#105333,
#105334,#105335,#105336,#105337,#105338,#105339,#105340,#105341,#105342,
#105343,#105344,#105345,#105346,#105347,#105348,#105349,#105350,#105351,
#105352,#105353,#105354,#105355,#105356,#105357,#105358,#105359,#105360,
#105361,#105362,#105363,#105364,#105365,#105366,#105367,#105368,#105369,
#105370,#105371,#105372,#105373,#105374,#105375,#105376,#105377,#105378,
#105379,#105380,#105381,#105382,#105383,#105384,#105385,#105386,#105387,
#105388,#105389,#105390,#105391,#105392),.UNSPECIFIED.,.F.,.F.,(4,3,3,3,
3,3,3,3,3,3,3,3,3,3,3,3,3,3,3,3,3,3,3,3,3,3,3,3,3,3,3,3,3,3,3,3,3,3,3,3,
3,3,3,3,3,3,3,3,3,3,3,3,3,3,3,3,3,3,3,3,3,3,3,3,3,3,3,3,3,4),(0.00187081090387685,
0.00271260435668075,0.00362268902859932,0.0047088961595475,0.0051051220936109,
0.00599081910917896,0.00672227768847788,0.00778276880660481,0.00833943328334486,
0.00942599481828414,0.0104998696456815,0.0115737444730788,0.0123823222705124,
0.0131909000679459,0.0142060282592838,0.014808055662813,0.0157081299291953,
0.0164252112576801,0.0170970893496155,0.0177619833705849,0.0180423668525471,
0.0190026734096196,0.0199503685611344,0.0208795972594173,0.0212766780422811,
0.0222765344942665,0.0232692933815988,0.0242499722556933,0.0245109892320151,
0.0253195670294486,0.0257488472900959,0.0261281448268821,0.0270598184241087,
0.027745300421749,0.0287399757306378,0.029362456016616,0.0299897241643665,
0.0306190954857663,0.030979611611483,0.0318533830950635,0.0327383246442732,
0.0336403396115905,0.034213922801217,0.0352558542716055,0.035831078396084,
0.0367181867272809,0.0374482339909511,0.0384960606253587,0.0395893029030219,
0.0406825451806851,0.0413774134031492,0.0420918307002056,0.0422997007755522,
0.0433943605093599,0.0439168563704194,0.045023602051156,0.0455340119652865,
0.04634258976272,0.0470220692264879,0.0471511675601536,0.04802900043527,
0.0488603746190379,0.0496350381747814,0.050385478749888,0.0511032328730951,
0.0517960284135882,0.0520026343447552,0.0527090367424356,0.0534533603415317,
0.0536197899396224),.UNSPECIFIED.);
#2350=B_SPLINE_CURVE_WITH_KNOTS('',3,(#105393,#105394,#105395,#105396,#105397,
#105398,#105399,#105400,#105401,#105402,#105403,#105404,#105405,#105406,
#105407,#105408,#105409,#105410,#105411,#105412,#105413,#105414,#105415,
#105416,#105417,#105418,#105419,#105420,#105421,#105422,#105423,#105424,
#105425,#105426,#105427,#105428,#105429,#105430,#105431,#105432,#105433,
#105434,#105435,#105436,#105437,#105438,#105439,#105440,#105441,#105442,
#105443,#105444),.UNSPECIFIED.,.F.,.F.,(4,2,2,2,2,2,2,2,2,2,2,2,2,2,2,2,
2,2,2,2,2,2,2,2,2,4),(0.000252666121810611,0.00283443432717517,0.00412531842985747,
0.00541620253253977,0.00799797073790439,0.00928885484058674,0.0105797389432691,
0.0118706230459514,0.0131615071486338,0.0157432753539985,0.0170341594566808,
0.018325043559363,0.0196159276620453,0.0209068117647276,0.0234885799700922,
0.0247794640727745,0.0260703481754568,0.0286521163808214,0.0299430004835037,
0.031233884586186,0.0338156527915506,0.0363974209969151,0.0376883050995973,
0.0389791892022796,0.0402700733049619,0.0415609574076441),.UNSPECIFIED.);
#2351=B_SPLINE_CURVE_WITH_KNOTS('',3,(#105992,#105993,#105994,#105995,#105996,
#105997),.UNSPECIFIED.,.F.,.F.,(4,2,4),(0.,0.000429537087177428,0.000859074174354856),
 .UNSPECIFIED.);
#2352=B_SPLINE_CURVE_WITH_KNOTS('',3,(#106005,#106006,#106007,#106008,#106009,
#106010,#106011,#106012,#106013,#106014,#106015,#106016,#106017,#106018,
#106019,#106020,#106021,#106022,#106023,#106024,#106025,#106026),
 .UNSPECIFIED.,.F.,.F.,(4,3,3,3,3,3,3,4),(1.38777878078145E-17,0.000188059268556367,
0.000214020122328391,0.000428040244656768,0.000642060366985145,0.000721468200741508,
0.000798165243973893,0.000856080489313522),.UNSPECIFIED.);
#2353=B_SPLINE_CURVE_WITH_KNOTS('',3,(#106031,#106032,#106033,#106034,#106035,
#106036,#106037,#106038,#106039,#106040,#106041,#106042,#106043,#106044,
#106045,#106046,#106047,#106048,#106049,#106050,#106051,#106052),
 .UNSPECIFIED.,.F.,.F.,(4,3,3,3,3,3,3,4),(0.,7.79304036744801E-5,0.000158641952040327,
0.00021866555281504,0.000437331105630081,0.000655996658445121,0.000848137862261846,
0.000874662211260162),.UNSPECIFIED.);
#2354=B_SPLINE_CURVE_WITH_KNOTS('',3,(#106060,#106061,#106062,#106063,#106064,
#106065),.UNSPECIFIED.,.F.,.F.,(4,2,4),(1.38777878078145E-17,0.000428854539313667,
0.00085770907862732),.UNSPECIFIED.);
#2355=B_SPLINE_CURVE_WITH_KNOTS('',3,(#106068,#106069,#106070,#106071,#106072,
#106073,#106074,#106075,#106076,#106077,#106078,#106079,#106080,#106081,
#106082,#106083,#106084,#106085,#106086,#106087,#106088,#106089,#106090,
#106091,#106092,#106093,#106094,#106095,#106096,#106097,#106098,#106099,
#106100,#106101,#106102,#106103,#106104,#106105,#106106,#106107,#106108,
#106109,#106110,#106111,#106112,#106113,#106114,#106115,#106116),
 .UNSPECIFIED.,.F.,.F.,(4,3,3,3,3,3,3,3,3,3,3,3,3,3,3,3,4),(0.,0.000172655359583005,
0.000214472733930129,0.000345356453129998,0.00040194427569836,0.000426371089395591,
0.000551635597584684,0.000633757499696936,0.000803888551396719,0.000836019899938085,
0.00100450939519915,0.00116399791926213,0.00120583282709508,0.00122724609507386,
0.00139282382099101,0.00156108680528541,0.00160777710279344),
 .UNSPECIFIED.);
#2356=B_SPLINE_CURVE_WITH_KNOTS('',3,(#106119,#106120,#106121,#106122,#106123,
#106124,#106125,#106126,#106127,#106128,#106129,#106130,#106131,#106132,
#106133,#106134,#106135,#106136,#106137,#106138,#106139,#106140,#106141,
#106142,#106143,#106144,#106145,#106146,#106147,#106148,#106149,#106150,
#106151,#106152,#106153,#106154,#106155,#106156,#106157,#106158,#106159,
#106160,#106161),.UNSPECIFIED.,.F.,.F.,(4,3,3,3,3,3,3,3,3,3,3,3,3,3,4),
(0.,0.00097071180919006,0.00109494777504685,0.00211704535126196,0.00219853891044863,
0.00223735799194462,0.00296830632650111,0.00376840487765825,0.00443540273119751,
0.00447471598388924,0.00577557119702807,0.00668663775574798,0.00671207397583386,
0.00820153167491206,0.00894943196777848),.UNSPECIFIED.);
#2357=B_SPLINE_CURVE_WITH_KNOTS('',3,(#106237,#106238,#106239,#106240,#106241,
#106242,#106243,#106244,#106245,#106246,#106247,#106248,#106249,#106250,
#106251,#106252,#106253,#106254,#106255,#106256,#106257,#106258,#106259,
#106260,#106261,#106262,#106263,#106264,#106265,#106266,#106267,#106268,
#106269,#106270,#106271,#106272,#106273,#106274,#106275,#106276,#106277,
#106278,#106279),.UNSPECIFIED.,.F.,.F.,(4,3,3,3,3,3,3,3,3,3,3,3,3,3,4),
(0.,0.000970711791819082,0.0010949477750237,0.00211704534669127,0.00219853891044869,
0.00223735799194468,0.00296830632781392,0.0037684048802517,0.00443540273119768,
0.00447471598388935,0.00577557115859329,0.0066866377557481,0.00671207397583403,
0.00820153142505179,0.00894943196777871),.UNSPECIFIED.);
#2358=B_SPLINE_CURVE_WITH_KNOTS('',3,(#106281,#106282,#106283,#106284,#106285,
#106286,#106287,#106288,#106289,#106290,#106291,#106292,#106293,#106294,
#106295,#106296,#106297,#106298,#106299,#106300,#106301,#106302,#106303,
#106304,#106305,#106306,#106307,#106308,#106309,#106310,#106311,#106312,
#106313,#106314,#106315,#106316,#106317,#106318,#106319,#106320,#106321,
#106322,#106323,#106324,#106325,#106326,#106327,#106328,#106329,#106330,
#106331,#106332,#106333,#106334,#106335),.UNSPECIFIED.,.F.,.F.,(4,3,3,3,
3,3,3,3,3,3,3,3,3,3,3,3,3,3,4),(0.,0.00011263901958812,0.000224528452761069,
0.000335876538867614,0.000378780084712497,0.000403082142219989,0.000535803330753571,
0.000671115250426468,0.000770572167488891,0.000806164284439978,0.000922051893666942,
0.000990761403542633,0.00108645700528024,0.00114554120348879,0.00118215260701784,
0.00126269703837782,0.00139376821745601,0.00152129814935798,0.00161232856888021),
 .UNSPECIFIED.);
#2359=B_SPLINE_CURVE_WITH_KNOTS('',3,(#106339,#106340,#106341,#106342,#106343,
#106344,#106345,#106346,#106347,#106348,#106349,#106350,#106351,#106352,
#106353,#106354,#106355,#106356,#106357,#106358,#106359,#106360,#106361,
#106362,#106363,#106364,#106365,#106366,#106367,#106368,#106369,#106370,
#106371,#106372,#106373,#106374,#106375,#106376,#106377,#106378,#106379,
#106380,#106381,#106382,#106383,#106384,#106385,#106386,#106387),
 .UNSPECIFIED.,.F.,.F.,(4,3,3,3,3,3,3,3,3,3,3,3,3,3,3,3,4),(0.,0.000167524699450898,
0.000332355096398968,0.00037843928853009,0.000399734851137576,0.000557949097585033,
0.000724839875838272,0.000767514974710719,0.000799469702275151,0.000968665570301764,
0.001093241519164,0.00117491201007438,0.00119920455341273,0.00132936882535921,
0.00138564559355697,0.00155735189376102,0.0015989394045503),
 .UNSPECIFIED.);
#2360=B_SPLINE_CURVE_WITH_KNOTS('',3,(#106393,#106394,#106395,#106396,#106397,
#106398,#106399,#106400,#106401,#106402),.UNSPECIFIED.,.F.,.F.,(4,2,2,2,
4),(0.,0.000406430200333951,0.000812860400667902,0.00121929060100185,0.0016257208013358),
 .UNSPECIFIED.);
#2925=SHAPE_REPRESENTATION_RELATIONSHIP('SRR','None',#130947,#2933);
#2933=ADVANCED_BREP_SHAPE_REPRESENTATION('',(#2947),#130907);
#2941=STYLED_ITEM('',(#130991),#2947);
#2947=MANIFOLD_SOLID_BREP('Body1',#45457);
#3635=PLANE('',#48825);
#3636=PLANE('',#48828);
#3637=PLANE('',#48834);
#3638=PLANE('',#48837);
#3639=PLANE('',#48843);
#3640=PLANE('',#48844);
#3641=PLANE('',#48847);
#3642=PLANE('',#48848);
#5263=LINE('',#97319,#7037);
#5264=LINE('',#97321,#7038);
#5265=LINE('',#97406,#7039);
#5266=LINE('',#97420,#7040);
#5267=LINE('',#98900,#7041);
#5268=LINE('',#99188,#7042);
#5269=LINE('',#100546,#7043);
#5270=LINE('',#100753,#7044);
#5271=LINE('',#102877,#7045);
#5272=LINE('',#102959,#7046);
#5273=LINE('',#103475,#7047);
#5274=LINE('',#105942,#7048);
#5275=LINE('',#105945,#7049);
#5276=LINE('',#105948,#7050);
#5277=LINE('',#105951,#7051);
#5278=LINE('',#105953,#7052);
#5279=LINE('',#105956,#7053);
#5280=LINE('',#105961,#7054);
#5281=LINE('',#105963,#7055);
#5282=LINE('',#105966,#7056);
#5283=LINE('',#105967,#7057);
#5284=LINE('',#105973,#7058);
#5285=LINE('',#105976,#7059);
#5286=LINE('',#105978,#7060);
#5287=LINE('',#105979,#7061);
#5288=LINE('',#105984,#7062);
#5289=LINE('',#105985,#7063);
#5290=LINE('',#105987,#7064);
#5291=LINE('',#105988,#7065);
#5292=LINE('',#105999,#7066);
#5293=LINE('',#106001,#7067);
#5294=LINE('',#106003,#7068);
#5295=LINE('',#106027,#7069);
#5296=LINE('',#106054,#7070);
#5297=LINE('',#106056,#7071);
#5298=LINE('',#106058,#7072);
#5299=LINE('',#106066,#7073);
#7037=VECTOR('',#59006,19.4499999999999);
#7038=VECTOR('',#59007,1000.);
#7039=VECTOR('',#59010,1000.);
#7040=VECTOR('',#59029,19.45);
#7041=VECTOR('',#59046,12.3);
#7042=VECTOR('',#59051,15.7183063441034);
#7043=VECTOR('',#59082,12.2808574779498);
#7044=VECTOR('',#59085,19.45);
#7045=VECTOR('',#59102,12.3);
#7046=VECTOR('',#59107,15.7183063441034);
#7047=VECTOR('',#59114,5.84048589276829);
#7048=VECTOR('',#59131,1000.);
#7049=VECTOR('',#59134,1000.);
#7050=VECTOR('',#59137,1000.);
#7051=VECTOR('',#59140,1000.);
#7052=VECTOR('',#59141,1000.);
#7053=VECTOR('',#59144,1000.);
#7054=VECTOR('',#59149,1000.);
#7055=VECTOR('',#59150,1000.);
#7056=VECTOR('',#59153,1000.);
#7057=VECTOR('',#59154,1000.);
#7058=VECTOR('',#59159,1000.);
#7059=VECTOR('',#59162,1000.);
#7060=VECTOR('',#59165,1000.);
#7061=VECTOR('',#59166,1000.);
#7062=VECTOR('',#59171,1000.);
#7063=VECTOR('',#59172,1000.);
#7064=VECTOR('',#59175,1000.);
#7065=VECTOR('',#59176,1000.);
#7066=VECTOR('',#59179,1000.);
#7067=VECTOR('',#59180,1000.);
#7068=VECTOR('',#59181,1000.);
#7069=VECTOR('',#59182,1000.);
#7070=VECTOR('',#59185,1000.);
#7071=VECTOR('',#59186,1000.);
#7072=VECTOR('',#59187,1000.);
#7073=VECTOR('',#59188,1000.);
#8654=CYLINDRICAL_SURFACE('',#48775,19.4499999999999);
#8655=CYLINDRICAL_SURFACE('',#48785,19.45);
#8656=CYLINDRICAL_SURFACE('',#48793,12.3);
#8657=CYLINDRICAL_SURFACE('',#48795,15.7183063441034);
#8658=CYLINDRICAL_SURFACE('',#48810,12.2808574779498);
#8659=CYLINDRICAL_SURFACE('',#48811,19.45);
#8660=CYLINDRICAL_SURFACE('',#48819,12.3);
#8661=CYLINDRICAL_SURFACE('',#48821,15.7183063441034);
#8662=CYLINDRICAL_SURFACE('',#48824,5.84048589276829);
#8663=CYLINDRICAL_SURFACE('',#48826,19.45);
#8664=CYLINDRICAL_SURFACE('',#48827,21.0115219102092);
#8665=CYLINDRICAL_SURFACE('',#48829,19.45);
#8666=CYLINDRICAL_SURFACE('',#48830,21.0115219102092);
#8667=CYLINDRICAL_SURFACE('',#48831,18.1223816084529);
#8668=CYLINDRICAL_SURFACE('',#48840,18.1223816084529);
#8669=CYLINDRICAL_SURFACE('',#48846,12.2099993856753);
#8670=CYLINDRICAL_SURFACE('',#48851,1.);
#8671=CYLINDRICAL_SURFACE('',#48857,1.);
#8672=CYLINDRICAL_SURFACE('',#48860,1.);
#8673=CYLINDRICAL_SURFACE('',#48861,1.);
#8674=CYLINDRICAL_SURFACE('',#48866,0.5);
#8675=CYLINDRICAL_SURFACE('',#48868,0.5);
#8676=CYLINDRICAL_SURFACE('',#48873,0.5);
#8677=CYLINDRICAL_SURFACE('',#48875,0.5);
#8678=CYLINDRICAL_SURFACE('',#48877,0.5);
#8679=CYLINDRICAL_SURFACE('',#48884,0.5);
#8680=CYLINDRICAL_SURFACE('',#48886,0.5);
#8681=CYLINDRICAL_SURFACE('',#48891,0.5);
#11203=FACE_OUTER_BOUND('',#15245,.T.);
#11204=FACE_OUTER_BOUND('',#15246,.T.);
#11205=FACE_OUTER_BOUND('',#15247,.T.);
#11206=FACE_OUTER_BOUND('',#15248,.T.);
#11207=FACE_OUTER_BOUND('',#15249,.T.);
#11208=FACE_OUTER_BOUND('',#15250,.T.);
#11209=FACE_OUTER_BOUND('',#15251,.T.);
#11210=FACE_OUTER_BOUND('',#15252,.T.);
#11211=FACE_OUTER_BOUND('',#15253,.T.);
#11212=FACE_OUTER_BOUND('',#15254,.T.);
#11213=FACE_OUTER_BOUND('',#15255,.T.);
#11214=FACE_OUTER_BOUND('',#15256,.T.);
#11215=FACE_OUTER_BOUND('',#15257,.T.);
#11216=FACE_OUTER_BOUND('',#15258,.T.);
#11217=FACE_OUTER_BOUND('',#15259,.T.);
#11218=FACE_OUTER_BOUND('',#15260,.T.);
#11219=FACE_OUTER_BOUND('',#15261,.T.);
#11220=FACE_OUTER_BOUND('',#15262,.T.);
#11221=FACE_OUTER_BOUND('',#15263,.T.);
#11222=FACE_OUTER_BOUND('',#15264,.T.);
#11223=FACE_OUTER_BOUND('',#15268,.T.);
#11224=FACE_OUTER_BOUND('',#15269,.T.);
#11225=FACE_OUTER_BOUND('',#15270,.T.);
#11226=FACE_OUTER_BOUND('',#15271,.T.);
#11227=FACE_OUTER_BOUND('',#15272,.T.);
#11228=FACE_OUTER_BOUND('',#15273,.T.);
#11229=FACE_OUTER_BOUND('',#15274,.T.);
#11230=FACE_OUTER_BOUND('',#15275,.T.);
#11231=FACE_OUTER_BOUND('',#15276,.T.);
#11232=FACE_OUTER_BOUND('',#15277,.T.);
#11233=FACE_OUTER_BOUND('',#15279,.T.);
#11234=FACE_OUTER_BOUND('',#15281,.T.);
#11235=FACE_OUTER_BOUND('',#15282,.T.);
#11236=FACE_OUTER_BOUND('',#15283,.T.);
#11237=FACE_OUTER_BOUND('',#15284,.T.);
#11238=FACE_OUTER_BOUND('',#15285,.T.);
#11239=FACE_OUTER_BOUND('',#15286,.T.);
#11240=FACE_OUTER_BOUND('',#15287,.T.);
#11241=FACE_OUTER_BOUND('',#15288,.T.);
#11242=FACE_OUTER_BOUND('',#15290,.T.);
#11243=FACE_OUTER_BOUND('',#15292,.T.);
#11244=FACE_OUTER_BOUND('',#15293,.T.);
#11245=FACE_OUTER_BOUND('',#15294,.T.);
#11246=FACE_OUTER_BOUND('',#15295,.T.);
#11247=FACE_OUTER_BOUND('',#15296,.T.);
#11248=FACE_OUTER_BOUND('',#15297,.T.);
#11249=FACE_OUTER_BOUND('',#15298,.T.);
#11250=FACE_OUTER_BOUND('',#15299,.T.);
#11251=FACE_OUTER_BOUND('',#15300,.T.);
#11252=FACE_OUTER_BOUND('',#15301,.T.);
#11253=FACE_OUTER_BOUND('',#15302,.T.);
#11254=FACE_OUTER_BOUND('',#15303,.T.);
#11255=FACE_OUTER_BOUND('',#15304,.T.);
#11256=FACE_OUTER_BOUND('',#15305,.T.);
#11257=FACE_OUTER_BOUND('',#15306,.T.);
#11258=FACE_OUTER_BOUND('',#15307,.T.);
#11259=FACE_OUTER_BOUND('',#15308,.T.);
#11260=FACE_OUTER_BOUND('',#15309,.T.);
#11261=FACE_OUTER_BOUND('',#15310,.T.);
#11262=FACE_OUTER_BOUND('',#15311,.T.);
#11263=FACE_OUTER_BOUND('',#15312,.T.);
#11264=FACE_OUTER_BOUND('',#15313,.T.);
#11265=FACE_OUTER_BOUND('',#15314,.T.);
#11266=FACE_OUTER_BOUND('',#15315,.T.);
#11267=FACE_OUTER_BOUND('',#15316,.T.);
#11268=FACE_OUTER_BOUND('',#15317,.T.);
#11269=FACE_OUTER_BOUND('',#15318,.T.);
#11270=FACE_OUTER_BOUND('',#15319,.T.);
#11271=FACE_OUTER_BOUND('',#15320,.T.);
#11272=FACE_OUTER_BOUND('',#15321,.T.);
#11273=FACE_OUTER_BOUND('',#15322,.T.);
#11274=FACE_OUTER_BOUND('',#15323,.T.);
#11275=FACE_OUTER_BOUND('',#15324,.T.);
#11276=FACE_OUTER_BOUND('',#15325,.T.);
#11277=FACE_OUTER_BOUND('',#15326,.T.);
#11278=FACE_OUTER_BOUND('',#15327,.T.);
#11279=FACE_OUTER_BOUND('',#15328,.T.);
#11280=FACE_OUTER_BOUND('',#15329,.T.);
#11281=FACE_OUTER_BOUND('',#15330,.T.);
#15245=EDGE_LOOP('',(#36426,#36427,#36428,#36429,#36430));
#15246=EDGE_LOOP('',(#36431,#36432,#36433,#36434));
#15247=EDGE_LOOP('',(#36435,#36436,#36437,#36438));
#15248=EDGE_LOOP('',(#36439,#36440,#36441,#36442,#36443));
#15249=EDGE_LOOP('',(#36444,#36445,#36446,#36447,#36448,#36449,#36450,#36451,
#36452,#36453,#36454));
#15250=EDGE_LOOP('',(#36455,#36456,#36457,#36458,#36459));
#15251=EDGE_LOOP('',(#36460,#36461,#36462,#36463));
#15252=EDGE_LOOP('',(#36464,#36465,#36466,#36467,#36468));
#15253=EDGE_LOOP('',(#36469,#36470,#36471,#36472,#36473));
#15254=EDGE_LOOP('',(#36474,#36475,#36476,#36477,#36478));
#15255=EDGE_LOOP('',(#36479,#36480,#36481,#36482,#36483));
#15256=EDGE_LOOP('',(#36484,#36485,#36486,#36487,#36488,#36489,#36490,#36491));
#15257=EDGE_LOOP('',(#36492,#36493,#36494,#36495,#36496,#36497,#36498,#36499,
#36500,#36501));
#15258=EDGE_LOOP('',(#36502,#36503,#36504,#36505,#36506));
#15259=EDGE_LOOP('',(#36507,#36508,#36509,#36510,#36511));
#15260=EDGE_LOOP('',(#36512,#36513,#36514,#36515,#36516));
#15261=EDGE_LOOP('',(#36517,#36518,#36519,#36520));
#15262=EDGE_LOOP('',(#36521,#36522,#36523,#36524,#36525));
#15263=EDGE_LOOP('',(#36526,#36527,#36528,#36529,#36530,#36531,#36532,#36533,
#36534,#36535));
#15264=EDGE_LOOP('',(#36536,#36537,#36538,#36539,#36540));
#15265=EDGE_LOOP('',(#36541,#36542));
#15266=EDGE_LOOP('',(#36543,#36544));
#15267=EDGE_LOOP('',(#36545,#36546));
#15268=EDGE_LOOP('',(#36547,#36548,#36549,#36550,#36551));
#15269=EDGE_LOOP('',(#36552,#36553,#36554,#36555,#36556));
#15270=EDGE_LOOP('',(#36557,#36558,#36559,#36560,#36561));
#15271=EDGE_LOOP('',(#36562,#36563,#36564,#36565,#36566,#36567,#36568));
#15272=EDGE_LOOP('',(#36569,#36570,#36571,#36572,#36573,#36574,#36575,#36576,
#36577,#36578));
#15273=EDGE_LOOP('',(#36579,#36580,#36581,#36582));
#15274=EDGE_LOOP('',(#36583,#36584,#36585,#36586,#36587,#36588,#36589,#36590));
#15275=EDGE_LOOP('',(#36591,#36592));
#15276=EDGE_LOOP('',(#36593,#36594,#36595,#36596));
#15277=EDGE_LOOP('',(#36597,#36598));
#15278=EDGE_LOOP('',(#36599));
#15279=EDGE_LOOP('',(#36600,#36601));
#15280=EDGE_LOOP('',(#36602,#36603));
#15281=EDGE_LOOP('',(#36604,#36605,#36606,#36607,#36608));
#15282=EDGE_LOOP('',(#36609,#36610,#36611,#36612,#36613));
#15283=EDGE_LOOP('',(#36614,#36615,#36616,#36617,#36618));
#15284=EDGE_LOOP('',(#36619));
#15285=EDGE_LOOP('',(#36620,#36621,#36622,#36623,#36624));
#15286=EDGE_LOOP('',(#36625,#36626,#36627,#36628,#36629));
#15287=EDGE_LOOP('',(#36630,#36631,#36632,#36633,#36634));
#15288=EDGE_LOOP('',(#36635,#36636));
#15289=EDGE_LOOP('',(#36637,#36638));
#15290=EDGE_LOOP('',(#36639,#36640));
#15291=EDGE_LOOP('',(#36641,#36642));
#15292=EDGE_LOOP('',(#36643,#36644,#36645,#36646,#36647));
#15293=EDGE_LOOP('',(#36648,#36649,#36650,#36651,#36652));
#15294=EDGE_LOOP('',(#36653,#36654,#36655,#36656,#36657));
#15295=EDGE_LOOP('',(#36658,#36659,#36660,#36661));
#15296=EDGE_LOOP('',(#36662,#36663,#36664,#36665,#36666,#36667,#36668,#36669));
#15297=EDGE_LOOP('',(#36670,#36671,#36672,#36673,#36674,#36675,#36676,#36677));
#15298=EDGE_LOOP('',(#36678,#36679,#36680,#36681));
#15299=EDGE_LOOP('',(#36682,#36683,#36684,#36685));
#15300=EDGE_LOOP('',(#36686,#36687,#36688,#36689));
#15301=EDGE_LOOP('',(#36690,#36691,#36692,#36693));
#15302=EDGE_LOOP('',(#36694,#36695,#36696,#36697,#36698,#36699));
#15303=EDGE_LOOP('',(#36700,#36701,#36702,#36703,#36704,#36705));
#15304=EDGE_LOOP('',(#36706,#36707,#36708,#36709));
#15305=EDGE_LOOP('',(#36710,#36711,#36712,#36713));
#15306=EDGE_LOOP('',(#36714,#36715,#36716));
#15307=EDGE_LOOP('',(#36717,#36718,#36719,#36720));
#15308=EDGE_LOOP('',(#36721,#36722,#36723));
#15309=EDGE_LOOP('',(#36724,#36725,#36726,#36727));
#15310=EDGE_LOOP('',(#36728,#36729,#36730,#36731));
#15311=EDGE_LOOP('',(#36732,#36733,#36734,#36735));
#15312=EDGE_LOOP('',(#36736,#36737,#36738,#36739));
#15313=EDGE_LOOP('',(#36740,#36741,#36742,#36743));
#15314=EDGE_LOOP('',(#36744,#36745,#36746,#36747));
#15315=EDGE_LOOP('',(#36748,#36749,#36750,#36751));
#15316=EDGE_LOOP('',(#36752,#36753,#36754,#36755));
#15317=EDGE_LOOP('',(#36756,#36757,#36758,#36759));
#15318=EDGE_LOOP('',(#36760,#36761,#36762));
#15319=EDGE_LOOP('',(#36763,#36764,#36765,#36766));
#15320=EDGE_LOOP('',(#36767,#36768,#36769,#36770));
#15321=EDGE_LOOP('',(#36771,#36772,#36773,#36774));
#15322=EDGE_LOOP('',(#36775,#36776,#36777,#36778));
#15323=EDGE_LOOP('',(#36779,#36780,#36781));
#15324=EDGE_LOOP('',(#36782,#36783,#36784));
#15325=EDGE_LOOP('',(#36785,#36786,#36787,#36788));
#15326=EDGE_LOOP('',(#36789,#36790,#36791,#36792));
#15327=EDGE_LOOP('',(#36793,#36794,#36795,#36796));
#15328=EDGE_LOOP('',(#36797,#36798,#36799));
#15329=EDGE_LOOP('',(#36800,#36801,#36802,#36803));
#15330=EDGE_LOOP('',(#36804,#36805,#36806,#36807));
#19315=CIRCLE('',#48755,19.4499999999999);
#19316=CIRCLE('',#48756,19.4499999999999);
#19317=CIRCLE('',#48757,0.5);
#19318=CIRCLE('',#48758,18.95);
#19319=CIRCLE('',#48760,12.2099993856753);
#19320=CIRCLE('',#48761,0.500000000000003);
#19321=CIRCLE('',#48762,12.7099993856753);
#19322=CIRCLE('',#48763,0.500000000000003);
#19323=CIRCLE('',#48765,12.7099993856753);
#19324=CIRCLE('',#48766,0.500000000000003);
#19325=CIRCLE('',#48767,12.2099993856753);
#19326=CIRCLE('',#48768,0.500000000000003);
#19327=CIRCLE('',#48770,19.4499999999999);
#19328=CIRCLE('',#48771,1.);
#19329=CIRCLE('',#48772,18.4499999999999);
#19330=CIRCLE('',#48773,1.);
#19331=CIRCLE('',#48774,19.4499999999999);
#19332=CIRCLE('',#48776,19.4499999999999);
#19333=CIRCLE('',#48778,0.5);
#19334=CIRCLE('',#48779,19.45);
#19335=CIRCLE('',#48780,19.45);
#19336=CIRCLE('',#48782,18.95);
#19337=CIRCLE('',#48783,0.5);
#19338=CIRCLE('',#48784,19.45);
#19339=CIRCLE('',#48786,0.250000000000021);
#19340=CIRCLE('',#48787,0.250000000000041);
#19341=CIRCLE('',#48788,0.249999999999985);
#19342=CIRCLE('',#48789,0.250000000000026);
#19343=CIRCLE('',#48790,0.249999999999998);
#19344=CIRCLE('',#48791,0.249999999999995);
#19345=CIRCLE('',#48792,9.76525702848835);
#19346=CIRCLE('',#48794,9.76341648719587);
#19347=CIRCLE('',#48796,0.500000000000001);
#19348=CIRCLE('',#48797,0.500000000000002);
#19349=CIRCLE('',#48798,0.500000000000001);
#19350=CIRCLE('',#48799,0.499999999999998);
#19351=CIRCLE('',#48800,0.500000000000001);
#19352=CIRCLE('',#48801,0.499999999999998);
#19353=CIRCLE('',#48803,19.45);
#19354=CIRCLE('',#48804,0.5);
#19355=CIRCLE('',#48806,19.45);
#19356=CIRCLE('',#48807,19.45);
#19357=CIRCLE('',#48808,1.);
#19358=CIRCLE('',#48809,18.45);
#19359=CIRCLE('',#48812,0.250000000000021);
#19360=CIRCLE('',#48813,0.250000000000042);
#19361=CIRCLE('',#48814,0.249999999999985);
#19362=CIRCLE('',#48815,0.250000000000026);
#19363=CIRCLE('',#48816,0.249999999999998);
#19364=CIRCLE('',#48817,9.76525702848803);
#19365=CIRCLE('',#48818,0.249999999999995);
#19366=CIRCLE('',#48820,9.76341648759087);
#19367=CIRCLE('',#48822,1.);
#19368=CIRCLE('',#48823,1.);
#19369=CIRCLE('',#48832,18.1223816084529);
#19370=CIRCLE('',#48833,18.1223816084529);
#19371=CIRCLE('',#48835,17.1223816084529);
#19372=CIRCLE('',#48836,17.1223816084529);
#19373=CIRCLE('',#48838,17.1223816084529);
#19374=CIRCLE('',#48839,17.1223816084529);
#19375=CIRCLE('',#48841,18.1223816084529);
#19376=CIRCLE('',#48842,18.1223816084529);
#19377=CIRCLE('',#48845,20.4499999999999);
#19378=CIRCLE('',#48850,1.);
#19379=CIRCLE('',#48852,1.00000000000002);
#19380=CIRCLE('',#48854,1.00000000000002);
#19381=CIRCLE('',#48856,1.);
#19382=CIRCLE('',#48859,1.);
#19383=CIRCLE('',#48862,1.);
#19384=CIRCLE('',#48864,0.5);
#19385=CIRCLE('',#48865,0.5);
#19386=CIRCLE('',#48867,0.5);
#19387=CIRCLE('',#48869,0.5);
#19388=CIRCLE('',#48871,0.5);
#19389=CIRCLE('',#48872,0.5);
#19390=CIRCLE('',#48874,0.5);
#19391=CIRCLE('',#48876,0.5);
#19392=CIRCLE('',#48878,0.5);
#19393=CIRCLE('',#48879,0.499999999999994);
#19394=CIRCLE('',#48881,0.5);
#19395=CIRCLE('',#48883,0.5);
#19396=CIRCLE('',#48885,0.5);
#19397=CIRCLE('',#48887,0.5);
#19398=CIRCLE('',#48889,0.5);
#19399=CIRCLE('',#48890,0.5);
#22611=VERTEX_POINT('',#97282);
#22612=VERTEX_POINT('',#97283);
#22613=VERTEX_POINT('',#97286);
#22614=VERTEX_POINT('',#97290);
#22615=VERTEX_POINT('',#97291);
#22616=VERTEX_POINT('',#97293);
#22617=VERTEX_POINT('',#97295);
#22618=VERTEX_POINT('',#97299);
#22619=VERTEX_POINT('',#97300);
#22620=VERTEX_POINT('',#97302);
#22621=VERTEX_POINT('',#97304);
#22622=VERTEX_POINT('',#97308);
#22623=VERTEX_POINT('',#97309);
#22624=VERTEX_POINT('',#97311);
#22625=VERTEX_POINT('',#97313);
#22626=VERTEX_POINT('',#97315);
#22627=VERTEX_POINT('',#97320);
#22628=VERTEX_POINT('',#97322);
#22629=VERTEX_POINT('',#97360);
#22630=VERTEX_POINT('',#97362);
#22631=VERTEX_POINT('',#97408);
#22632=VERTEX_POINT('',#97410);
#22633=VERTEX_POINT('',#97414);
#22634=VERTEX_POINT('',#97416);
#22635=VERTEX_POINT('',#97601);
#22636=VERTEX_POINT('',#97602);
#22637=VERTEX_POINT('',#97778);
#22638=VERTEX_POINT('',#97780);
#22639=VERTEX_POINT('',#97839);
#22640=VERTEX_POINT('',#98005);
#22641=VERTEX_POINT('',#98006);
#22642=VERTEX_POINT('',#98061);
#22643=VERTEX_POINT('',#98063);
#22644=VERTEX_POINT('',#98287);
#22645=VERTEX_POINT('',#98449);
#22646=VERTEX_POINT('',#98450);
#22647=VERTEX_POINT('',#98665);
#22648=VERTEX_POINT('',#98667);
#22649=VERTEX_POINT('',#98867);
#22650=VERTEX_POINT('',#98871);
#22651=VERTEX_POINT('',#98872);
#22652=VERTEX_POINT('',#98899);
#22653=VERTEX_POINT('',#98981);
#22654=VERTEX_POINT('',#99187);
#22655=VERTEX_POINT('',#99412);
#22656=VERTEX_POINT('',#99413);
#22657=VERTEX_POINT('',#99559);
#22658=VERTEX_POINT('',#99561);
#22659=VERTEX_POINT('',#99746);
#22660=VERTEX_POINT('',#99916);
#22661=VERTEX_POINT('',#99917);
#22662=VERTEX_POINT('',#99972);
#22663=VERTEX_POINT('',#99974);
#22664=VERTEX_POINT('',#100031);
#22665=VERTEX_POINT('',#100208);
#22666=VERTEX_POINT('',#100209);
#22667=VERTEX_POINT('',#100264);
#22668=VERTEX_POINT('',#100266);
#22669=VERTEX_POINT('',#100323);
#22670=VERTEX_POINT('',#100339);
#22671=VERTEX_POINT('',#100343);
#22672=VERTEX_POINT('',#100344);
#22673=VERTEX_POINT('',#100347);
#22674=VERTEX_POINT('',#100351);
#22675=VERTEX_POINT('',#100545);
#22676=VERTEX_POINT('',#100974);
#22677=VERTEX_POINT('',#100975);
#22678=VERTEX_POINT('',#101615);
#22679=VERTEX_POINT('',#101617);
#22680=VERTEX_POINT('',#101793);
#22681=VERTEX_POINT('',#101959);
#22682=VERTEX_POINT('',#101960);
#22683=VERTEX_POINT('',#102184);
#22684=VERTEX_POINT('',#102186);
#22685=VERTEX_POINT('',#102241);
#22686=VERTEX_POINT('',#102403);
#22687=VERTEX_POINT('',#102404);
#22688=VERTEX_POINT('',#102604);
#22689=VERTEX_POINT('',#102606);
#22690=VERTEX_POINT('',#102821);
#22691=VERTEX_POINT('',#102825);
#22692=VERTEX_POINT('',#102876);
#22693=VERTEX_POINT('',#102932);
#22694=VERTEX_POINT('',#102958);
#22695=VERTEX_POINT('',#103279);
#22696=VERTEX_POINT('',#103280);
#22697=VERTEX_POINT('',#103306);
#22698=VERTEX_POINT('',#103308);
#22699=VERTEX_POINT('',#103329);
#22700=VERTEX_POINT('',#105938);
#22701=VERTEX_POINT('',#105939);
#22702=VERTEX_POINT('',#105941);
#22703=VERTEX_POINT('',#105943);
#22704=VERTEX_POINT('',#105947);
#22705=VERTEX_POINT('',#105949);
#22706=VERTEX_POINT('',#105952);
#22707=VERTEX_POINT('',#105954);
#22708=VERTEX_POINT('',#105958);
#22709=VERTEX_POINT('',#105959);
#22710=VERTEX_POINT('',#105962);
#22711=VERTEX_POINT('',#105964);
#22712=VERTEX_POINT('',#105969);
#22713=VERTEX_POINT('',#105970);
#22714=VERTEX_POINT('',#105972);
#22715=VERTEX_POINT('',#105974);
#22716=VERTEX_POINT('',#105981);
#22717=VERTEX_POINT('',#105982);
#22718=VERTEX_POINT('',#105990);
#22719=VERTEX_POINT('',#105991);
#22720=VERTEX_POINT('',#105998);
#22721=VERTEX_POINT('',#106000);
#22722=VERTEX_POINT('',#106002);
#22723=VERTEX_POINT('',#106004);
#22724=VERTEX_POINT('',#106029);
#22725=VERTEX_POINT('',#106030);
#22726=VERTEX_POINT('',#106053);
#22727=VERTEX_POINT('',#106055);
#22728=VERTEX_POINT('',#106057);
#22729=VERTEX_POINT('',#106059);
#27557=EDGE_CURVE('',#22611,#22612,#19315,.T.);
#27558=EDGE_CURVE('',#22612,#22611,#19316,.T.);
#27559=EDGE_CURVE('',#22612,#22613,#19317,.T.);
#27560=EDGE_CURVE('',#22613,#22613,#19318,.T.);
#27561=EDGE_CURVE('',#22614,#22615,#19319,.T.);
#27562=EDGE_CURVE('',#22616,#22614,#19320,.T.);
#27563=EDGE_CURVE('',#22617,#22616,#19321,.T.);
#27564=EDGE_CURVE('',#22617,#22615,#19322,.T.);
#27565=EDGE_CURVE('',#22618,#22619,#19323,.T.);
#27566=EDGE_CURVE('',#22620,#22618,#19324,.T.);
#27567=EDGE_CURVE('',#22621,#22620,#19325,.T.);
#27568=EDGE_CURVE('',#22621,#22619,#19326,.T.);
#27569=EDGE_CURVE('',#22622,#22623,#19327,.T.);
#27570=EDGE_CURVE('',#22622,#22624,#19328,.T.);
#27571=EDGE_CURVE('',#22625,#22624,#19329,.T.);
#27572=EDGE_CURVE('',#22626,#22625,#19330,.T.);
#27573=EDGE_CURVE('',#22623,#22626,#19331,.T.);
#27574=EDGE_CURVE('',#22611,#22623,#5263,.T.);
#27575=EDGE_CURVE('',#22626,#22627,#5264,.T.);
#27576=EDGE_CURVE('',#22627,#22628,#2294,.T.);
#27577=EDGE_CURVE('',#22628,#22629,#19332,.T.);
#27578=EDGE_CURVE('',#22629,#22630,#2295,.T.);
#27579=EDGE_CURVE('',#22622,#22630,#5265,.T.);
#27580=EDGE_CURVE('',#22613,#22631,#19333,.T.);
#27581=EDGE_CURVE('',#22632,#22631,#19334,.T.);
#27582=EDGE_CURVE('',#22631,#22632,#19335,.T.);
#27583=EDGE_CURVE('',#22633,#22633,#19336,.T.);
#27584=EDGE_CURVE('',#22633,#22634,#19337,.T.);
#27585=EDGE_CURVE('',#22634,#22634,#19338,.T.);
#27586=EDGE_CURVE('',#22634,#22632,#5266,.T.);
#27587=EDGE_CURVE('',#22635,#22636,#2296,.T.);
#27588=EDGE_CURVE('',#22636,#22637,#19339,.T.);
#27589=EDGE_CURVE('',#22637,#22638,#2297,.T.);
#27590=EDGE_CURVE('',#22639,#22638,#19340,.T.);
#27591=EDGE_CURVE('',#22639,#22635,#2298,.T.);
#27592=EDGE_CURVE('',#22640,#22641,#2299,.T.);
#27593=EDGE_CURVE('',#22641,#22642,#19341,.T.);
#27594=EDGE_CURVE('',#22642,#22643,#2300,.T.);
#27595=EDGE_CURVE('',#22644,#22643,#19342,.T.);
#27596=EDGE_CURVE('',#22644,#22640,#2301,.T.);
#27597=EDGE_CURVE('',#22645,#22646,#2302,.T.);
#27598=EDGE_CURVE('',#22646,#22647,#19343,.T.);
#27599=EDGE_CURVE('',#22647,#22648,#2303,.T.);
#27600=EDGE_CURVE('',#22649,#22648,#19344,.T.);
#27601=EDGE_CURVE('',#22649,#22645,#19345,.T.);
#27602=EDGE_CURVE('',#22650,#22651,#2304,.T.);
#27603=EDGE_CURVE('',#22651,#22652,#5267,.T.);
#27604=EDGE_CURVE('',#22646,#22652,#19346,.T.);
#27605=EDGE_CURVE('',#22652,#22649,#2305,.T.);
#27606=EDGE_CURVE('',#22651,#22650,#2306,.T.);
#27607=EDGE_CURVE('',#22653,#22644,#2307,.T.);
#27608=EDGE_CURVE('',#22653,#22654,#5268,.T.);
#27609=EDGE_CURVE('',#22636,#22654,#2308,.T.);
#27610=EDGE_CURVE('',#22654,#22639,#2309,.T.);
#27611=EDGE_CURVE('',#22641,#22653,#2310,.T.);
#27612=EDGE_CURVE('',#22655,#22656,#2311,.T.);
#27613=EDGE_CURVE('',#22655,#22657,#19347,.T.);
#27614=EDGE_CURVE('',#22658,#22657,#2312,.T.);
#27615=EDGE_CURVE('',#22659,#22658,#19348,.T.);
#27616=EDGE_CURVE('',#22656,#22659,#2313,.T.);
#27617=EDGE_CURVE('',#22660,#22661,#2314,.T.);
#27618=EDGE_CURVE('',#22660,#22662,#19349,.T.);
#27619=EDGE_CURVE('',#22663,#22662,#2315,.T.);
#27620=EDGE_CURVE('',#22664,#22663,#19350,.T.);
#27621=EDGE_CURVE('',#22661,#22664,#2316,.T.);
#27622=EDGE_CURVE('',#22665,#22666,#2317,.T.);
#27623=EDGE_CURVE('',#22665,#22667,#19351,.T.);
#27624=EDGE_CURVE('',#22668,#22667,#2318,.T.);
#27625=EDGE_CURVE('',#22669,#22668,#19352,.T.);
#27626=EDGE_CURVE('',#22666,#22669,#2319,.T.);
#27627=EDGE_CURVE('',#22670,#22670,#19353,.T.);
#27628=EDGE_CURVE('',#22670,#22633,#19354,.T.);
#27629=EDGE_CURVE('',#22671,#22672,#19355,.T.);
#27630=EDGE_CURVE('',#22672,#22671,#19356,.T.);
#27631=EDGE_CURVE('',#22672,#22673,#19357,.T.);
#27632=EDGE_CURVE('',#22673,#22673,#19358,.T.);
#27633=EDGE_CURVE('',#22664,#22674,#2320,.T.);
#27634=EDGE_CURVE('',#22674,#22675,#5269,.T.);
#27635=EDGE_CURVE('',#22675,#22665,#2321,.T.);
#27636=EDGE_CURVE('',#22669,#22675,#2322,.T.);
#27637=EDGE_CURVE('',#22674,#22660,#2323,.T.);
#27638=EDGE_CURVE('',#22671,#22670,#5270,.T.);
#27639=EDGE_CURVE('',#22638,#22637,#2324,.T.);
#27640=EDGE_CURVE('',#22676,#22677,#2325,.T.);
#27641=EDGE_CURVE('',#22677,#22676,#2326,.T.);
#27642=EDGE_CURVE('',#22657,#22658,#2327,.T.);
#27643=EDGE_CURVE('',#22677,#22678,#19359,.T.);
#27644=EDGE_CURVE('',#22679,#22678,#2328,.T.);
#27645=EDGE_CURVE('',#22680,#22679,#2329,.T.);
#27646=EDGE_CURVE('',#22676,#22680,#19360,.T.);
#27647=EDGE_CURVE('',#22681,#22682,#2330,.T.);
#27648=EDGE_CURVE('',#22681,#22683,#19361,.T.);
#27649=EDGE_CURVE('',#22684,#22683,#2331,.T.);
#27650=EDGE_CURVE('',#22685,#22684,#2332,.T.);
#27651=EDGE_CURVE('',#22682,#22685,#19362,.T.);
#27652=EDGE_CURVE('',#22686,#22687,#2333,.T.);
#27653=EDGE_CURVE('',#22686,#22688,#19363,.T.);
#27654=EDGE_CURVE('',#22689,#22688,#2334,.T.);
#27655=EDGE_CURVE('',#22690,#22689,#19364,.T.);
#27656=EDGE_CURVE('',#22687,#22690,#19365,.T.);
#27657=EDGE_CURVE('',#22691,#22691,#2335,.T.);
#27658=EDGE_CURVE('',#22691,#22692,#5271,.T.);
#27659=EDGE_CURVE('',#22692,#22690,#2336,.T.);
#27660=EDGE_CURVE('',#22688,#22692,#19366,.T.);
#27661=EDGE_CURVE('',#22683,#22693,#2337,.T.);
#27662=EDGE_CURVE('',#22693,#22694,#5272,.T.);
#27663=EDGE_CURVE('',#22694,#22680,#2338,.T.);
#27664=EDGE_CURVE('',#22678,#22694,#2339,.T.);
#27665=EDGE_CURVE('',#22693,#22685,#2340,.T.);
#27666=EDGE_CURVE('',#22695,#22696,#2341,.T.);
#27667=EDGE_CURVE('',#22695,#22697,#19367,.T.);
#27668=EDGE_CURVE('',#22698,#22697,#43,.T.);
#27669=EDGE_CURVE('',#22696,#22698,#19368,.T.);
#27670=EDGE_CURVE('',#22659,#22699,#2342,.T.);
#27671=EDGE_CURVE('',#22699,#22698,#5273,.T.);
#27672=EDGE_CURVE('',#22697,#22698,#44,.T.);
#27673=EDGE_CURVE('',#22699,#22655,#2343,.T.);
#27674=EDGE_CURVE('',#22696,#22695,#2344,.T.);
#27675=EDGE_CURVE('',#22667,#22668,#2345,.T.);
#27676=EDGE_CURVE('',#22682,#22681,#2346,.T.);
#27677=EDGE_CURVE('',#22687,#22686,#2347,.T.);
#27678=EDGE_CURVE('',#22662,#22663,#2348,.T.);
#27679=EDGE_CURVE('',#22643,#22642,#2349,.T.);
#27680=EDGE_CURVE('',#22648,#22647,#2350,.T.);
#27681=EDGE_CURVE('',#22700,#22701,#19369,.T.);
#27682=EDGE_CURVE('',#22701,#22702,#5274,.T.);
#27683=EDGE_CURVE('',#22702,#22703,#19370,.T.);
#27684=EDGE_CURVE('',#22700,#22703,#5275,.T.);
#27685=EDGE_CURVE('',#22616,#22704,#5276,.T.);
#27686=EDGE_CURVE('',#22704,#22705,#19371,.T.);
#27687=EDGE_CURVE('',#22705,#22622,#5277,.T.);
#27688=EDGE_CURVE('',#22630,#22706,#5278,.T.);
#27689=EDGE_CURVE('',#22706,#22707,#19372,.T.);
#27690=EDGE_CURVE('',#22707,#22617,#5279,.T.);
#27691=EDGE_CURVE('',#22708,#22709,#19373,.T.);
#27692=EDGE_CURVE('',#22709,#22618,#5280,.T.);
#27693=EDGE_CURVE('',#22619,#22710,#5281,.T.);
#27694=EDGE_CURVE('',#22710,#22711,#19374,.T.);
#27695=EDGE_CURVE('',#22711,#22627,#5282,.T.);
#27696=EDGE_CURVE('',#22626,#22708,#5283,.T.);
#27697=EDGE_CURVE('',#22712,#22713,#19375,.T.);
#27698=EDGE_CURVE('',#22713,#22714,#5284,.T.);
#27699=EDGE_CURVE('',#22714,#22715,#19376,.T.);
#27700=EDGE_CURVE('',#22712,#22715,#5285,.T.);
#27701=EDGE_CURVE('',#22703,#22625,#5286,.T.);
#27702=EDGE_CURVE('',#22624,#22700,#5287,.T.);
#27703=EDGE_CURVE('',#22716,#22717,#19377,.T.);
#27704=EDGE_CURVE('',#22717,#22712,#5288,.T.);
#27705=EDGE_CURVE('',#22715,#22716,#5289,.T.);
#27706=EDGE_CURVE('',#22615,#22621,#5290,.T.);
#27707=EDGE_CURVE('',#22620,#22614,#5291,.T.);
#27708=EDGE_CURVE('',#22718,#22719,#2351,.T.);
#27709=EDGE_CURVE('',#22719,#22720,#5292,.T.);
#27710=EDGE_CURVE('',#22720,#22721,#5293,.T.);
#27711=EDGE_CURVE('',#22721,#22722,#5294,.T.);
#27712=EDGE_CURVE('',#22722,#22723,#2352,.T.);
#27713=EDGE_CURVE('',#22723,#22718,#5295,.T.);
#27714=EDGE_CURVE('',#22724,#22725,#2353,.T.);
#27715=EDGE_CURVE('',#22725,#22726,#5296,.T.);
#27716=EDGE_CURVE('',#22726,#22727,#5297,.T.);
#27717=EDGE_CURVE('',#22727,#22728,#5298,.T.);
#27718=EDGE_CURVE('',#22728,#22729,#2354,.T.);
#27719=EDGE_CURVE('',#22729,#22724,#5299,.T.);
#27720=EDGE_CURVE('',#22714,#22707,#2355,.T.);
#27721=EDGE_CURVE('',#22715,#22706,#19378,.T.);
#27722=EDGE_CURVE('',#22716,#22630,#2356,.T.);
#27723=EDGE_CURVE('',#22716,#22629,#19379,.T.);
#27724=EDGE_CURVE('',#22717,#22628,#19380,.T.);
#27725=EDGE_CURVE('',#22717,#22627,#2357,.T.);
#27726=EDGE_CURVE('',#22710,#22713,#2358,.T.);
#27727=EDGE_CURVE('',#22711,#22712,#19381,.T.);
#27728=EDGE_CURVE('',#22704,#22701,#2359,.T.);
#27729=EDGE_CURVE('',#22705,#22700,#19382,.T.);
#27730=EDGE_CURVE('',#22708,#22703,#19383,.T.);
#27731=EDGE_CURVE('',#22702,#22709,#2360,.T.);
#27732=EDGE_CURVE('',#22713,#22724,#19384,.T.);
#27733=EDGE_CURVE('',#22725,#22710,#19385,.T.);
#27734=EDGE_CURVE('',#22726,#22619,#19386,.T.);
#27735=EDGE_CURVE('',#22714,#22729,#19387,.T.);
#27736=EDGE_CURVE('',#22726,#22621,#19388,.T.);
#27737=EDGE_CURVE('',#22707,#22728,#19389,.T.);
#27738=EDGE_CURVE('',#22727,#22615,#19390,.T.);
#27739=EDGE_CURVE('',#22617,#22727,#19391,.T.);
#27740=EDGE_CURVE('',#22618,#22721,#19392,.T.);
#27741=EDGE_CURVE('',#22722,#22709,#19393,.T.);
#27742=EDGE_CURVE('',#22620,#22721,#19394,.T.);
#27743=EDGE_CURVE('',#22723,#22702,#19395,.T.);
#27744=EDGE_CURVE('',#22614,#22720,#19396,.T.);
#27745=EDGE_CURVE('',#22718,#22701,#19397,.T.);
#27746=EDGE_CURVE('',#22616,#22720,#19398,.T.);
#27747=EDGE_CURVE('',#22719,#22704,#19399,.T.);
#36426=ORIENTED_EDGE('',*,*,#27557,.F.);
#36427=ORIENTED_EDGE('',*,*,#27558,.F.);
#36428=ORIENTED_EDGE('',*,*,#27559,.T.);
#36429=ORIENTED_EDGE('',*,*,#27560,.T.);
#36430=ORIENTED_EDGE('',*,*,#27559,.F.);
#36431=ORIENTED_EDGE('',*,*,#27561,.F.);
#36432=ORIENTED_EDGE('',*,*,#27562,.F.);
#36433=ORIENTED_EDGE('',*,*,#27563,.F.);
#36434=ORIENTED_EDGE('',*,*,#27564,.T.);
#36435=ORIENTED_EDGE('',*,*,#27565,.F.);
#36436=ORIENTED_EDGE('',*,*,#27566,.F.);
#36437=ORIENTED_EDGE('',*,*,#27567,.F.);
#36438=ORIENTED_EDGE('',*,*,#27568,.T.);
#36439=ORIENTED_EDGE('',*,*,#27569,.F.);
#36440=ORIENTED_EDGE('',*,*,#27570,.T.);
#36441=ORIENTED_EDGE('',*,*,#27571,.F.);
#36442=ORIENTED_EDGE('',*,*,#27572,.F.);
#36443=ORIENTED_EDGE('',*,*,#27573,.F.);
#36444=ORIENTED_EDGE('',*,*,#27557,.T.);
#36445=ORIENTED_EDGE('',*,*,#27558,.T.);
#36446=ORIENTED_EDGE('',*,*,#27574,.T.);
#36447=ORIENTED_EDGE('',*,*,#27573,.T.);
#36448=ORIENTED_EDGE('',*,*,#27575,.T.);
#36449=ORIENTED_EDGE('',*,*,#27576,.T.);
#36450=ORIENTED_EDGE('',*,*,#27577,.T.);
#36451=ORIENTED_EDGE('',*,*,#27578,.T.);
#36452=ORIENTED_EDGE('',*,*,#27579,.F.);
#36453=ORIENTED_EDGE('',*,*,#27569,.T.);
#36454=ORIENTED_EDGE('',*,*,#27574,.F.);
#36455=ORIENTED_EDGE('',*,*,#27560,.F.);
#36456=ORIENTED_EDGE('',*,*,#27580,.T.);
#36457=ORIENTED_EDGE('',*,*,#27581,.F.);
#36458=ORIENTED_EDGE('',*,*,#27582,.F.);
#36459=ORIENTED_EDGE('',*,*,#27580,.F.);
#36460=ORIENTED_EDGE('',*,*,#27583,.T.);
#36461=ORIENTED_EDGE('',*,*,#27584,.T.);
#36462=ORIENTED_EDGE('',*,*,#27585,.F.);
#36463=ORIENTED_EDGE('',*,*,#27584,.F.);
#36464=ORIENTED_EDGE('',*,*,#27585,.T.);
#36465=ORIENTED_EDGE('',*,*,#27586,.T.);
#36466=ORIENTED_EDGE('',*,*,#27581,.T.);
#36467=ORIENTED_EDGE('',*,*,#27582,.T.);
#36468=ORIENTED_EDGE('',*,*,#27586,.F.);
#36469=ORIENTED_EDGE('',*,*,#27587,.T.);
#36470=ORIENTED_EDGE('',*,*,#27588,.T.);
#36471=ORIENTED_EDGE('',*,*,#27589,.T.);
#36472=ORIENTED_EDGE('',*,*,#27590,.F.);
#36473=ORIENTED_EDGE('',*,*,#27591,.T.);
#36474=ORIENTED_EDGE('',*,*,#27592,.T.);
#36475=ORIENTED_EDGE('',*,*,#27593,.T.);
#36476=ORIENTED_EDGE('',*,*,#27594,.T.);
#36477=ORIENTED_EDGE('',*,*,#27595,.F.);
#36478=ORIENTED_EDGE('',*,*,#27596,.T.);
#36479=ORIENTED_EDGE('',*,*,#27597,.T.);
#36480=ORIENTED_EDGE('',*,*,#27598,.T.);
#36481=ORIENTED_EDGE('',*,*,#27599,.T.);
#36482=ORIENTED_EDGE('',*,*,#27600,.F.);
#36483=ORIENTED_EDGE('',*,*,#27601,.T.);
#36484=ORIENTED_EDGE('',*,*,#27602,.T.);
#36485=ORIENTED_EDGE('',*,*,#27603,.T.);
#36486=ORIENTED_EDGE('',*,*,#27604,.F.);
#36487=ORIENTED_EDGE('',*,*,#27597,.F.);
#36488=ORIENTED_EDGE('',*,*,#27601,.F.);
#36489=ORIENTED_EDGE('',*,*,#27605,.F.);
#36490=ORIENTED_EDGE('',*,*,#27603,.F.);
#36491=ORIENTED_EDGE('',*,*,#27606,.T.);
#36492=ORIENTED_EDGE('',*,*,#27596,.F.);
#36493=ORIENTED_EDGE('',*,*,#27607,.F.);
#36494=ORIENTED_EDGE('',*,*,#27608,.T.);
#36495=ORIENTED_EDGE('',*,*,#27609,.F.);
#36496=ORIENTED_EDGE('',*,*,#27587,.F.);
#36497=ORIENTED_EDGE('',*,*,#27591,.F.);
#36498=ORIENTED_EDGE('',*,*,#27610,.F.);
#36499=ORIENTED_EDGE('',*,*,#27608,.F.);
#36500=ORIENTED_EDGE('',*,*,#27611,.F.);
#36501=ORIENTED_EDGE('',*,*,#27592,.F.);
#36502=ORIENTED_EDGE('',*,*,#27612,.F.);
#36503=ORIENTED_EDGE('',*,*,#27613,.T.);
#36504=ORIENTED_EDGE('',*,*,#27614,.F.);
#36505=ORIENTED_EDGE('',*,*,#27615,.F.);
#36506=ORIENTED_EDGE('',*,*,#27616,.F.);
#36507=ORIENTED_EDGE('',*,*,#27617,.F.);
#36508=ORIENTED_EDGE('',*,*,#27618,.T.);
#36509=ORIENTED_EDGE('',*,*,#27619,.F.);
#36510=ORIENTED_EDGE('',*,*,#27620,.F.);
#36511=ORIENTED_EDGE('',*,*,#27621,.F.);
#36512=ORIENTED_EDGE('',*,*,#27622,.F.);
#36513=ORIENTED_EDGE('',*,*,#27623,.T.);
#36514=ORIENTED_EDGE('',*,*,#27624,.F.);
#36515=ORIENTED_EDGE('',*,*,#27625,.F.);
#36516=ORIENTED_EDGE('',*,*,#27626,.F.);
#36517=ORIENTED_EDGE('',*,*,#27627,.F.);
#36518=ORIENTED_EDGE('',*,*,#27628,.T.);
#36519=ORIENTED_EDGE('',*,*,#27583,.F.);
#36520=ORIENTED_EDGE('',*,*,#27628,.F.);
#36521=ORIENTED_EDGE('',*,*,#27629,.F.);
#36522=ORIENTED_EDGE('',*,*,#27630,.F.);
#36523=ORIENTED_EDGE('',*,*,#27631,.T.);
#36524=ORIENTED_EDGE('',*,*,#27632,.F.);
#36525=ORIENTED_EDGE('',*,*,#27631,.F.);
#36526=ORIENTED_EDGE('',*,*,#27621,.T.);
#36527=ORIENTED_EDGE('',*,*,#27633,.T.);
#36528=ORIENTED_EDGE('',*,*,#27634,.T.);
#36529=ORIENTED_EDGE('',*,*,#27635,.T.);
#36530=ORIENTED_EDGE('',*,*,#27622,.T.);
#36531=ORIENTED_EDGE('',*,*,#27626,.T.);
#36532=ORIENTED_EDGE('',*,*,#27636,.T.);
#36533=ORIENTED_EDGE('',*,*,#27634,.F.);
#36534=ORIENTED_EDGE('',*,*,#27637,.T.);
#36535=ORIENTED_EDGE('',*,*,#27617,.T.);
#36536=ORIENTED_EDGE('',*,*,#27629,.T.);
#36537=ORIENTED_EDGE('',*,*,#27630,.T.);
#36538=ORIENTED_EDGE('',*,*,#27638,.T.);
#36539=ORIENTED_EDGE('',*,*,#27627,.T.);
#36540=ORIENTED_EDGE('',*,*,#27638,.F.);
#36541=ORIENTED_EDGE('',*,*,#27639,.F.);
#36542=ORIENTED_EDGE('',*,*,#27589,.F.);
#36543=ORIENTED_EDGE('',*,*,#27640,.T.);
#36544=ORIENTED_EDGE('',*,*,#27641,.T.);
#36545=ORIENTED_EDGE('',*,*,#27614,.T.);
#36546=ORIENTED_EDGE('',*,*,#27642,.T.);
#36547=ORIENTED_EDGE('',*,*,#27641,.F.);
#36548=ORIENTED_EDGE('',*,*,#27643,.T.);
#36549=ORIENTED_EDGE('',*,*,#27644,.F.);
#36550=ORIENTED_EDGE('',*,*,#27645,.F.);
#36551=ORIENTED_EDGE('',*,*,#27646,.F.);
#36552=ORIENTED_EDGE('',*,*,#27647,.F.);
#36553=ORIENTED_EDGE('',*,*,#27648,.T.);
#36554=ORIENTED_EDGE('',*,*,#27649,.F.);
#36555=ORIENTED_EDGE('',*,*,#27650,.F.);
#36556=ORIENTED_EDGE('',*,*,#27651,.F.);
#36557=ORIENTED_EDGE('',*,*,#27652,.F.);
#36558=ORIENTED_EDGE('',*,*,#27653,.T.);
#36559=ORIENTED_EDGE('',*,*,#27654,.F.);
#36560=ORIENTED_EDGE('',*,*,#27655,.F.);
#36561=ORIENTED_EDGE('',*,*,#27656,.F.);
#36562=ORIENTED_EDGE('',*,*,#27657,.F.);
#36563=ORIENTED_EDGE('',*,*,#27658,.T.);
#36564=ORIENTED_EDGE('',*,*,#27659,.T.);
#36565=ORIENTED_EDGE('',*,*,#27655,.T.);
#36566=ORIENTED_EDGE('',*,*,#27654,.T.);
#36567=ORIENTED_EDGE('',*,*,#27660,.T.);
#36568=ORIENTED_EDGE('',*,*,#27658,.F.);
#36569=ORIENTED_EDGE('',*,*,#27649,.T.);
#36570=ORIENTED_EDGE('',*,*,#27661,.T.);
#36571=ORIENTED_EDGE('',*,*,#27662,.T.);
#36572=ORIENTED_EDGE('',*,*,#27663,.T.);
#36573=ORIENTED_EDGE('',*,*,#27645,.T.);
#36574=ORIENTED_EDGE('',*,*,#27644,.T.);
#36575=ORIENTED_EDGE('',*,*,#27664,.T.);
#36576=ORIENTED_EDGE('',*,*,#27662,.F.);
#36577=ORIENTED_EDGE('',*,*,#27665,.T.);
#36578=ORIENTED_EDGE('',*,*,#27650,.T.);
#36579=ORIENTED_EDGE('',*,*,#27666,.F.);
#36580=ORIENTED_EDGE('',*,*,#27667,.T.);
#36581=ORIENTED_EDGE('',*,*,#27668,.F.);
#36582=ORIENTED_EDGE('',*,*,#27669,.F.);
#36583=ORIENTED_EDGE('',*,*,#27616,.T.);
#36584=ORIENTED_EDGE('',*,*,#27670,.T.);
#36585=ORIENTED_EDGE('',*,*,#27671,.T.);
#36586=ORIENTED_EDGE('',*,*,#27668,.T.);
#36587=ORIENTED_EDGE('',*,*,#27672,.T.);
#36588=ORIENTED_EDGE('',*,*,#27671,.F.);
#36589=ORIENTED_EDGE('',*,*,#27673,.T.);
#36590=ORIENTED_EDGE('',*,*,#27612,.T.);
#36591=ORIENTED_EDGE('',*,*,#27674,.T.);
#36592=ORIENTED_EDGE('',*,*,#27666,.T.);
#36593=ORIENTED_EDGE('',*,*,#27667,.F.);
#36594=ORIENTED_EDGE('',*,*,#27674,.F.);
#36595=ORIENTED_EDGE('',*,*,#27669,.T.);
#36596=ORIENTED_EDGE('',*,*,#27672,.F.);
#36597=ORIENTED_EDGE('',*,*,#27624,.T.);
#36598=ORIENTED_EDGE('',*,*,#27675,.T.);
#36599=ORIENTED_EDGE('',*,*,#27657,.T.);
#36600=ORIENTED_EDGE('',*,*,#27676,.T.);
#36601=ORIENTED_EDGE('',*,*,#27647,.T.);
#36602=ORIENTED_EDGE('',*,*,#27677,.T.);
#36603=ORIENTED_EDGE('',*,*,#27652,.T.);
#36604=ORIENTED_EDGE('',*,*,#27653,.F.);
#36605=ORIENTED_EDGE('',*,*,#27677,.F.);
#36606=ORIENTED_EDGE('',*,*,#27656,.T.);
#36607=ORIENTED_EDGE('',*,*,#27659,.F.);
#36608=ORIENTED_EDGE('',*,*,#27660,.F.);
#36609=ORIENTED_EDGE('',*,*,#27648,.F.);
#36610=ORIENTED_EDGE('',*,*,#27676,.F.);
#36611=ORIENTED_EDGE('',*,*,#27651,.T.);
#36612=ORIENTED_EDGE('',*,*,#27665,.F.);
#36613=ORIENTED_EDGE('',*,*,#27661,.F.);
#36614=ORIENTED_EDGE('',*,*,#27643,.F.);
#36615=ORIENTED_EDGE('',*,*,#27640,.F.);
#36616=ORIENTED_EDGE('',*,*,#27646,.T.);
#36617=ORIENTED_EDGE('',*,*,#27663,.F.);
#36618=ORIENTED_EDGE('',*,*,#27664,.F.);
#36619=ORIENTED_EDGE('',*,*,#27632,.T.);
#36620=ORIENTED_EDGE('',*,*,#27623,.F.);
#36621=ORIENTED_EDGE('',*,*,#27635,.F.);
#36622=ORIENTED_EDGE('',*,*,#27636,.F.);
#36623=ORIENTED_EDGE('',*,*,#27625,.T.);
#36624=ORIENTED_EDGE('',*,*,#27675,.F.);
#36625=ORIENTED_EDGE('',*,*,#27618,.F.);
#36626=ORIENTED_EDGE('',*,*,#27637,.F.);
#36627=ORIENTED_EDGE('',*,*,#27633,.F.);
#36628=ORIENTED_EDGE('',*,*,#27620,.T.);
#36629=ORIENTED_EDGE('',*,*,#27678,.F.);
#36630=ORIENTED_EDGE('',*,*,#27613,.F.);
#36631=ORIENTED_EDGE('',*,*,#27673,.F.);
#36632=ORIENTED_EDGE('',*,*,#27670,.F.);
#36633=ORIENTED_EDGE('',*,*,#27615,.T.);
#36634=ORIENTED_EDGE('',*,*,#27642,.F.);
#36635=ORIENTED_EDGE('',*,*,#27619,.T.);
#36636=ORIENTED_EDGE('',*,*,#27678,.T.);
#36637=ORIENTED_EDGE('',*,*,#27602,.F.);
#36638=ORIENTED_EDGE('',*,*,#27606,.F.);
#36639=ORIENTED_EDGE('',*,*,#27679,.F.);
#36640=ORIENTED_EDGE('',*,*,#27594,.F.);
#36641=ORIENTED_EDGE('',*,*,#27680,.F.);
#36642=ORIENTED_EDGE('',*,*,#27599,.F.);
#36643=ORIENTED_EDGE('',*,*,#27598,.F.);
#36644=ORIENTED_EDGE('',*,*,#27604,.T.);
#36645=ORIENTED_EDGE('',*,*,#27605,.T.);
#36646=ORIENTED_EDGE('',*,*,#27600,.T.);
#36647=ORIENTED_EDGE('',*,*,#27680,.T.);
#36648=ORIENTED_EDGE('',*,*,#27593,.F.);
#36649=ORIENTED_EDGE('',*,*,#27611,.T.);
#36650=ORIENTED_EDGE('',*,*,#27607,.T.);
#36651=ORIENTED_EDGE('',*,*,#27595,.T.);
#36652=ORIENTED_EDGE('',*,*,#27679,.T.);
#36653=ORIENTED_EDGE('',*,*,#27588,.F.);
#36654=ORIENTED_EDGE('',*,*,#27609,.T.);
#36655=ORIENTED_EDGE('',*,*,#27610,.T.);
#36656=ORIENTED_EDGE('',*,*,#27590,.T.);
#36657=ORIENTED_EDGE('',*,*,#27639,.T.);
#36658=ORIENTED_EDGE('',*,*,#27681,.T.);
#36659=ORIENTED_EDGE('',*,*,#27682,.T.);
#36660=ORIENTED_EDGE('',*,*,#27683,.T.);
#36661=ORIENTED_EDGE('',*,*,#27684,.F.);
#36662=ORIENTED_EDGE('',*,*,#27563,.T.);
#36663=ORIENTED_EDGE('',*,*,#27685,.T.);
#36664=ORIENTED_EDGE('',*,*,#27686,.T.);
#36665=ORIENTED_EDGE('',*,*,#27687,.T.);
#36666=ORIENTED_EDGE('',*,*,#27579,.T.);
#36667=ORIENTED_EDGE('',*,*,#27688,.T.);
#36668=ORIENTED_EDGE('',*,*,#27689,.T.);
#36669=ORIENTED_EDGE('',*,*,#27690,.T.);
#36670=ORIENTED_EDGE('',*,*,#27691,.T.);
#36671=ORIENTED_EDGE('',*,*,#27692,.T.);
#36672=ORIENTED_EDGE('',*,*,#27565,.T.);
#36673=ORIENTED_EDGE('',*,*,#27693,.T.);
#36674=ORIENTED_EDGE('',*,*,#27694,.T.);
#36675=ORIENTED_EDGE('',*,*,#27695,.T.);
#36676=ORIENTED_EDGE('',*,*,#27575,.F.);
#36677=ORIENTED_EDGE('',*,*,#27696,.T.);
#36678=ORIENTED_EDGE('',*,*,#27697,.T.);
#36679=ORIENTED_EDGE('',*,*,#27698,.T.);
#36680=ORIENTED_EDGE('',*,*,#27699,.T.);
#36681=ORIENTED_EDGE('',*,*,#27700,.F.);
#36682=ORIENTED_EDGE('',*,*,#27684,.T.);
#36683=ORIENTED_EDGE('',*,*,#27701,.T.);
#36684=ORIENTED_EDGE('',*,*,#27571,.T.);
#36685=ORIENTED_EDGE('',*,*,#27702,.T.);
#36686=ORIENTED_EDGE('',*,*,#27703,.T.);
#36687=ORIENTED_EDGE('',*,*,#27704,.T.);
#36688=ORIENTED_EDGE('',*,*,#27700,.T.);
#36689=ORIENTED_EDGE('',*,*,#27705,.T.);
#36690=ORIENTED_EDGE('',*,*,#27561,.T.);
#36691=ORIENTED_EDGE('',*,*,#27706,.T.);
#36692=ORIENTED_EDGE('',*,*,#27567,.T.);
#36693=ORIENTED_EDGE('',*,*,#27707,.T.);
#36694=ORIENTED_EDGE('',*,*,#27708,.T.);
#36695=ORIENTED_EDGE('',*,*,#27709,.T.);
#36696=ORIENTED_EDGE('',*,*,#27710,.T.);
#36697=ORIENTED_EDGE('',*,*,#27711,.T.);
#36698=ORIENTED_EDGE('',*,*,#27712,.T.);
#36699=ORIENTED_EDGE('',*,*,#27713,.T.);
#36700=ORIENTED_EDGE('',*,*,#27714,.T.);
#36701=ORIENTED_EDGE('',*,*,#27715,.T.);
#36702=ORIENTED_EDGE('',*,*,#27716,.T.);
#36703=ORIENTED_EDGE('',*,*,#27717,.T.);
#36704=ORIENTED_EDGE('',*,*,#27718,.T.);
#36705=ORIENTED_EDGE('',*,*,#27719,.T.);
#36706=ORIENTED_EDGE('',*,*,#27699,.F.);
#36707=ORIENTED_EDGE('',*,*,#27720,.T.);
#36708=ORIENTED_EDGE('',*,*,#27689,.F.);
#36709=ORIENTED_EDGE('',*,*,#27721,.F.);
#36710=ORIENTED_EDGE('',*,*,#27721,.T.);
#36711=ORIENTED_EDGE('',*,*,#27688,.F.);
#36712=ORIENTED_EDGE('',*,*,#27722,.F.);
#36713=ORIENTED_EDGE('',*,*,#27705,.F.);
#36714=ORIENTED_EDGE('',*,*,#27722,.T.);
#36715=ORIENTED_EDGE('',*,*,#27578,.F.);
#36716=ORIENTED_EDGE('',*,*,#27723,.F.);
#36717=ORIENTED_EDGE('',*,*,#27723,.T.);
#36718=ORIENTED_EDGE('',*,*,#27577,.F.);
#36719=ORIENTED_EDGE('',*,*,#27724,.F.);
#36720=ORIENTED_EDGE('',*,*,#27703,.F.);
#36721=ORIENTED_EDGE('',*,*,#27724,.T.);
#36722=ORIENTED_EDGE('',*,*,#27576,.F.);
#36723=ORIENTED_EDGE('',*,*,#27725,.F.);
#36724=ORIENTED_EDGE('',*,*,#27694,.F.);
#36725=ORIENTED_EDGE('',*,*,#27726,.T.);
#36726=ORIENTED_EDGE('',*,*,#27697,.F.);
#36727=ORIENTED_EDGE('',*,*,#27727,.F.);
#36728=ORIENTED_EDGE('',*,*,#27725,.T.);
#36729=ORIENTED_EDGE('',*,*,#27695,.F.);
#36730=ORIENTED_EDGE('',*,*,#27727,.T.);
#36731=ORIENTED_EDGE('',*,*,#27704,.F.);
#36732=ORIENTED_EDGE('',*,*,#27686,.F.);
#36733=ORIENTED_EDGE('',*,*,#27728,.T.);
#36734=ORIENTED_EDGE('',*,*,#27681,.F.);
#36735=ORIENTED_EDGE('',*,*,#27729,.F.);
#36736=ORIENTED_EDGE('',*,*,#27729,.T.);
#36737=ORIENTED_EDGE('',*,*,#27702,.F.);
#36738=ORIENTED_EDGE('',*,*,#27570,.F.);
#36739=ORIENTED_EDGE('',*,*,#27687,.F.);
#36740=ORIENTED_EDGE('',*,*,#27572,.T.);
#36741=ORIENTED_EDGE('',*,*,#27701,.F.);
#36742=ORIENTED_EDGE('',*,*,#27730,.F.);
#36743=ORIENTED_EDGE('',*,*,#27696,.F.);
#36744=ORIENTED_EDGE('',*,*,#27683,.F.);
#36745=ORIENTED_EDGE('',*,*,#27731,.T.);
#36746=ORIENTED_EDGE('',*,*,#27691,.F.);
#36747=ORIENTED_EDGE('',*,*,#27730,.T.);
#36748=ORIENTED_EDGE('',*,*,#27732,.F.);
#36749=ORIENTED_EDGE('',*,*,#27726,.F.);
#36750=ORIENTED_EDGE('',*,*,#27733,.F.);
#36751=ORIENTED_EDGE('',*,*,#27714,.F.);
#36752=ORIENTED_EDGE('',*,*,#27733,.T.);
#36753=ORIENTED_EDGE('',*,*,#27693,.F.);
#36754=ORIENTED_EDGE('',*,*,#27734,.F.);
#36755=ORIENTED_EDGE('',*,*,#27715,.F.);
#36756=ORIENTED_EDGE('',*,*,#27732,.T.);
#36757=ORIENTED_EDGE('',*,*,#27719,.F.);
#36758=ORIENTED_EDGE('',*,*,#27735,.F.);
#36759=ORIENTED_EDGE('',*,*,#27698,.F.);
#36760=ORIENTED_EDGE('',*,*,#27736,.F.);
#36761=ORIENTED_EDGE('',*,*,#27734,.T.);
#36762=ORIENTED_EDGE('',*,*,#27568,.F.);
#36763=ORIENTED_EDGE('',*,*,#27735,.T.);
#36764=ORIENTED_EDGE('',*,*,#27718,.F.);
#36765=ORIENTED_EDGE('',*,*,#27737,.F.);
#36766=ORIENTED_EDGE('',*,*,#27720,.F.);
#36767=ORIENTED_EDGE('',*,*,#27736,.T.);
#36768=ORIENTED_EDGE('',*,*,#27706,.F.);
#36769=ORIENTED_EDGE('',*,*,#27738,.F.);
#36770=ORIENTED_EDGE('',*,*,#27716,.F.);
#36771=ORIENTED_EDGE('',*,*,#27737,.T.);
#36772=ORIENTED_EDGE('',*,*,#27717,.F.);
#36773=ORIENTED_EDGE('',*,*,#27739,.F.);
#36774=ORIENTED_EDGE('',*,*,#27690,.F.);
#36775=ORIENTED_EDGE('',*,*,#27740,.F.);
#36776=ORIENTED_EDGE('',*,*,#27692,.F.);
#36777=ORIENTED_EDGE('',*,*,#27741,.F.);
#36778=ORIENTED_EDGE('',*,*,#27711,.F.);
#36779=ORIENTED_EDGE('',*,*,#27566,.T.);
#36780=ORIENTED_EDGE('',*,*,#27740,.T.);
#36781=ORIENTED_EDGE('',*,*,#27742,.F.);
#36782=ORIENTED_EDGE('',*,*,#27739,.T.);
#36783=ORIENTED_EDGE('',*,*,#27738,.T.);
#36784=ORIENTED_EDGE('',*,*,#27564,.F.);
#36785=ORIENTED_EDGE('',*,*,#27741,.T.);
#36786=ORIENTED_EDGE('',*,*,#27731,.F.);
#36787=ORIENTED_EDGE('',*,*,#27743,.F.);
#36788=ORIENTED_EDGE('',*,*,#27712,.F.);
#36789=ORIENTED_EDGE('',*,*,#27742,.T.);
#36790=ORIENTED_EDGE('',*,*,#27710,.F.);
#36791=ORIENTED_EDGE('',*,*,#27744,.F.);
#36792=ORIENTED_EDGE('',*,*,#27707,.F.);
#36793=ORIENTED_EDGE('',*,*,#27743,.T.);
#36794=ORIENTED_EDGE('',*,*,#27682,.F.);
#36795=ORIENTED_EDGE('',*,*,#27745,.F.);
#36796=ORIENTED_EDGE('',*,*,#27713,.F.);
#36797=ORIENTED_EDGE('',*,*,#27562,.T.);
#36798=ORIENTED_EDGE('',*,*,#27744,.T.);
#36799=ORIENTED_EDGE('',*,*,#27746,.F.);
#36800=ORIENTED_EDGE('',*,*,#27745,.T.);
#36801=ORIENTED_EDGE('',*,*,#27728,.F.);
#36802=ORIENTED_EDGE('',*,*,#27747,.F.);
#36803=ORIENTED_EDGE('',*,*,#27708,.F.);
#36804=ORIENTED_EDGE('',*,*,#27746,.T.);
#36805=ORIENTED_EDGE('',*,*,#27709,.F.);
#36806=ORIENTED_EDGE('',*,*,#27747,.T.);
#36807=ORIENTED_EDGE('',*,*,#27685,.F.);
#42026=TOROIDAL_SURFACE('',#48754,18.9499999999999,0.5);
#42027=TOROIDAL_SURFACE('',#48759,12.7099993856753,0.5);
#42028=TOROIDAL_SURFACE('',#48764,12.7099993856753,0.5);
#42029=TOROIDAL_SURFACE('',#48769,18.4499999999999,1.);
#42030=TOROIDAL_SURFACE('',#48777,18.95,0.5);
#42031=TOROIDAL_SURFACE('',#48781,18.95,0.5);
#42032=TOROIDAL_SURFACE('',#48802,18.95,0.5);
#42033=TOROIDAL_SURFACE('',#48805,18.45,1.);
#42034=TOROIDAL_SURFACE('',#48849,17.122381608453,1.);
#42035=TOROIDAL_SURFACE('',#48853,20.4499999999999,1.);
#42036=TOROIDAL_SURFACE('',#48855,17.122381608453,1.);
#42037=TOROIDAL_SURFACE('',#48858,17.122381608453,1.);
#42038=TOROIDAL_SURFACE('',#48863,17.122381608453,1.);
#43783=ADVANCED_FACE('',(#11203),#42026,.T.);
#43784=ADVANCED_FACE('',(#11204),#42027,.T.);
#43785=ADVANCED_FACE('',(#11205),#42028,.T.);
#43786=ADVANCED_FACE('',(#11206),#42029,.T.);
#43787=ADVANCED_FACE('',(#11207),#8654,.T.);
#43788=ADVANCED_FACE('',(#11208),#42030,.T.);
#43789=ADVANCED_FACE('',(#11209),#42031,.T.);
#43790=ADVANCED_FACE('',(#11210),#8655,.T.);
#43791=ADVANCED_FACE('',(#11211),#1660,.T.);
#43792=ADVANCED_FACE('',(#11212),#1661,.T.);
#43793=ADVANCED_FACE('',(#11213),#1662,.T.);
#43794=ADVANCED_FACE('',(#11214),#8656,.F.);
#43795=ADVANCED_FACE('',(#11215),#8657,.T.);
#43796=ADVANCED_FACE('',(#11216),#1663,.T.);
#43797=ADVANCED_FACE('',(#11217),#1664,.T.);
#43798=ADVANCED_FACE('',(#11218),#1665,.T.);
#43799=ADVANCED_FACE('',(#11219),#42032,.T.);
#43800=ADVANCED_FACE('',(#11220),#42033,.T.);
#43801=ADVANCED_FACE('',(#11221),#8658,.F.);
#43802=ADVANCED_FACE('',(#11222,#724,#725,#726),#8659,.T.);
#43803=ADVANCED_FACE('',(#11223),#1666,.T.);
#43804=ADVANCED_FACE('',(#11224),#1667,.T.);
#43805=ADVANCED_FACE('',(#11225),#1668,.T.);
#43806=ADVANCED_FACE('',(#11226),#8660,.F.);
#43807=ADVANCED_FACE('',(#11227),#8661,.T.);
#43808=ADVANCED_FACE('',(#11228),#1669,.T.);
#43809=ADVANCED_FACE('',(#11229),#8662,.T.);
#43810=ADVANCED_FACE('',(#11230),#3635,.F.);
#43811=ADVANCED_FACE('',(#11231),#1670,.T.);
#43812=ADVANCED_FACE('',(#11232,#727),#8663,.F.);
#43813=ADVANCED_FACE('',(#11233,#728),#8664,.T.);
#43814=ADVANCED_FACE('',(#11234),#1671,.T.);
#43815=ADVANCED_FACE('',(#11235),#1672,.T.);
#43816=ADVANCED_FACE('',(#11236),#1673,.T.);
#43817=ADVANCED_FACE('',(#11237),#3636,.F.);
#43818=ADVANCED_FACE('',(#11238),#1674,.T.);
#43819=ADVANCED_FACE('',(#11239),#1675,.T.);
#43820=ADVANCED_FACE('',(#11240),#1676,.T.);
#43821=ADVANCED_FACE('',(#11241,#729),#8665,.F.);
#43822=ADVANCED_FACE('',(#11242,#730),#8666,.T.);
#43823=ADVANCED_FACE('',(#11243),#1677,.T.);
#43824=ADVANCED_FACE('',(#11244),#1678,.T.);
#43825=ADVANCED_FACE('',(#11245),#1679,.T.);
#43826=ADVANCED_FACE('',(#11246),#8667,.T.);
#43827=ADVANCED_FACE('',(#11247),#3637,.F.);
#43828=ADVANCED_FACE('',(#11248),#3638,.T.);
#43829=ADVANCED_FACE('',(#11249),#8668,.T.);
#43830=ADVANCED_FACE('',(#11250),#3639,.T.);
#43831=ADVANCED_FACE('',(#11251),#3640,.F.);
#43832=ADVANCED_FACE('',(#11252),#8669,.F.);
#43833=ADVANCED_FACE('',(#11253),#3641,.T.);
#43834=ADVANCED_FACE('',(#11254),#3642,.F.);
#43835=ADVANCED_FACE('',(#11255),#42034,.T.);
#43836=ADVANCED_FACE('',(#11256),#8670,.T.);
#43837=ADVANCED_FACE('',(#11257),#1680,.F.);
#43838=ADVANCED_FACE('',(#11258),#42035,.F.);
#43839=ADVANCED_FACE('',(#11259),#1681,.F.);
#43840=ADVANCED_FACE('',(#11260),#42036,.T.);
#43841=ADVANCED_FACE('',(#11261),#8671,.T.);
#43842=ADVANCED_FACE('',(#11262),#42037,.T.);
#43843=ADVANCED_FACE('',(#11263),#8672,.T.);
#43844=ADVANCED_FACE('',(#11264),#8673,.T.);
#43845=ADVANCED_FACE('',(#11265),#42038,.T.);
#43846=ADVANCED_FACE('',(#11266),#1682,.T.);
#43847=ADVANCED_FACE('',(#11267),#8674,.T.);
#43848=ADVANCED_FACE('',(#11268),#8675,.T.);
#43849=ADVANCED_FACE('',(#11269),#66,.T.);
#43850=ADVANCED_FACE('',(#11270),#1683,.T.);
#43851=ADVANCED_FACE('',(#11271),#8676,.T.);
#43852=ADVANCED_FACE('',(#11272),#8677,.T.);
#43853=ADVANCED_FACE('',(#11273),#8678,.T.);
#43854=ADVANCED_FACE('',(#11274),#67,.T.);
#43855=ADVANCED_FACE('',(#11275),#68,.T.);
#43856=ADVANCED_FACE('',(#11276),#1684,.T.);
#43857=ADVANCED_FACE('',(#11277),#8679,.T.);
#43858=ADVANCED_FACE('',(#11278),#8680,.T.);
#43859=ADVANCED_FACE('',(#11279),#69,.T.);
#43860=ADVANCED_FACE('',(#11280),#1685,.T.);
#43861=ADVANCED_FACE('',(#11281),#8681,.T.);
#45457=CLOSED_SHELL('',(#43783,#43784,#43785,#43786,#43787,#43788,#43789,
#43790,#43791,#43792,#43793,#43794,#43795,#43796,#43797,#43798,#43799,#43800,
#43801,#43802,#43803,#43804,#43805,#43806,#43807,#43808,#43809,#43810,#43811,
#43812,#43813,#43814,#43815,#43816,#43817,#43818,#43819,#43820,#43821,#43822,
#43823,#43824,#43825,#43826,#43827,#43828,#43829,#43830,#43831,#43832,#43833,
#43834,#43835,#43836,#43837,#43838,#43839,#43840,#43841,#43842,#43843,#43844,
#43845,#43846,#43847,#43848,#43849,#43850,#43851,#43852,#43853,#43854,#43855,
#43856,#43857,#43858,#43859,#43860,#43861));
#48753=AXIS2_PLACEMENT_3D('',#97280,#58960,#58961);
#48754=AXIS2_PLACEMENT_3D('',#97281,#58962,#58963);
#48755=AXIS2_PLACEMENT_3D('',#97284,#58964,#58965);
#48756=AXIS2_PLACEMENT_3D('',#97285,#58966,#58967);
#48757=AXIS2_PLACEMENT_3D('',#97287,#58968,#58969);
#48758=AXIS2_PLACEMENT_3D('',#97288,#58970,#58971);
#48759=AXIS2_PLACEMENT_3D('',#97289,#58972,#58973);
#48760=AXIS2_PLACEMENT_3D('',#97292,#58974,#58975);
#48761=AXIS2_PLACEMENT_3D('',#97294,#58976,#58977);
#48762=AXIS2_PLACEMENT_3D('',#97296,#58978,#58979);
#48763=AXIS2_PLACEMENT_3D('',#97297,#58980,#58981);
#48764=AXIS2_PLACEMENT_3D('',#97298,#58982,#58983);
#48765=AXIS2_PLACEMENT_3D('',#97301,#58984,#58985);
#48766=AXIS2_PLACEMENT_3D('',#97303,#58986,#58987);
#48767=AXIS2_PLACEMENT_3D('',#97305,#58988,#58989);
#48768=AXIS2_PLACEMENT_3D('',#97306,#58990,#58991);
#48769=AXIS2_PLACEMENT_3D('',#97307,#58992,#58993);
#48770=AXIS2_PLACEMENT_3D('',#97310,#58994,#58995);
#48771=AXIS2_PLACEMENT_3D('',#97312,#58996,#58997);
#48772=AXIS2_PLACEMENT_3D('',#97314,#58998,#58999);
#48773=AXIS2_PLACEMENT_3D('',#97316,#59000,#59001);
#48774=AXIS2_PLACEMENT_3D('',#97317,#59002,#59003);
#48775=AXIS2_PLACEMENT_3D('',#97318,#59004,#59005);
#48776=AXIS2_PLACEMENT_3D('',#97361,#59008,#59009);
#48777=AXIS2_PLACEMENT_3D('',#97407,#59011,#59012);
#48778=AXIS2_PLACEMENT_3D('',#97409,#59013,#59014);
#48779=AXIS2_PLACEMENT_3D('',#97411,#59015,#59016);
#48780=AXIS2_PLACEMENT_3D('',#97412,#59017,#59018);
#48781=AXIS2_PLACEMENT_3D('',#97413,#59019,#59020);
#48782=AXIS2_PLACEMENT_3D('',#97415,#59021,#59022);
#48783=AXIS2_PLACEMENT_3D('',#97417,#59023,#59024);
#48784=AXIS2_PLACEMENT_3D('',#97418,#59025,#59026);
#48785=AXIS2_PLACEMENT_3D('',#97419,#59027,#59028);
#48786=AXIS2_PLACEMENT_3D('',#97779,#59030,#59031);
#48787=AXIS2_PLACEMENT_3D('',#97840,#59032,#59033);
#48788=AXIS2_PLACEMENT_3D('',#98062,#59034,#59035);
#48789=AXIS2_PLACEMENT_3D('',#98288,#59036,#59037);
#48790=AXIS2_PLACEMENT_3D('',#98666,#59038,#59039);
#48791=AXIS2_PLACEMENT_3D('',#98868,#59040,#59041);
#48792=AXIS2_PLACEMENT_3D('',#98869,#59042,#59043);
#48793=AXIS2_PLACEMENT_3D('',#98870,#59044,#59045);
#48794=AXIS2_PLACEMENT_3D('',#98901,#59047,#59048);
#48795=AXIS2_PLACEMENT_3D('',#98980,#59049,#59050);
#48796=AXIS2_PLACEMENT_3D('',#99560,#59052,#59053);
#48797=AXIS2_PLACEMENT_3D('',#99747,#59054,#59055);
#48798=AXIS2_PLACEMENT_3D('',#99973,#59056,#59057);
#48799=AXIS2_PLACEMENT_3D('',#100032,#59058,#59059);
#48800=AXIS2_PLACEMENT_3D('',#100265,#59060,#59061);
#48801=AXIS2_PLACEMENT_3D('',#100324,#59062,#59063);
#48802=AXIS2_PLACEMENT_3D('',#100338,#59064,#59065);
#48803=AXIS2_PLACEMENT_3D('',#100340,#59066,#59067);
#48804=AXIS2_PLACEMENT_3D('',#100341,#59068,#59069);
#48805=AXIS2_PLACEMENT_3D('',#100342,#59070,#59071);
#48806=AXIS2_PLACEMENT_3D('',#100345,#59072,#59073);
#48807=AXIS2_PLACEMENT_3D('',#100346,#59074,#59075);
#48808=AXIS2_PLACEMENT_3D('',#100348,#59076,#59077);
#48809=AXIS2_PLACEMENT_3D('',#100349,#59078,#59079);
#48810=AXIS2_PLACEMENT_3D('',#100350,#59080,#59081);
#48811=AXIS2_PLACEMENT_3D('',#100752,#59083,#59084);
#48812=AXIS2_PLACEMENT_3D('',#101616,#59086,#59087);
#48813=AXIS2_PLACEMENT_3D('',#101802,#59088,#59089);
#48814=AXIS2_PLACEMENT_3D('',#102185,#59090,#59091);
#48815=AXIS2_PLACEMENT_3D('',#102252,#59092,#59093);
#48816=AXIS2_PLACEMENT_3D('',#102605,#59094,#59095);
#48817=AXIS2_PLACEMENT_3D('',#102822,#59096,#59097);
#48818=AXIS2_PLACEMENT_3D('',#102823,#59098,#59099);
#48819=AXIS2_PLACEMENT_3D('',#102824,#59100,#59101);
#48820=AXIS2_PLACEMENT_3D('',#102930,#59103,#59104);
#48821=AXIS2_PLACEMENT_3D('',#102931,#59105,#59106);
#48822=AXIS2_PLACEMENT_3D('',#103307,#59108,#59109);
#48823=AXIS2_PLACEMENT_3D('',#103327,#59110,#59111);
#48824=AXIS2_PLACEMENT_3D('',#103328,#59112,#59113);
#48825=AXIS2_PLACEMENT_3D('',#103500,#59115,#59116);
#48826=AXIS2_PLACEMENT_3D('',#103580,#59117,#59118);
#48827=AXIS2_PLACEMENT_3D('',#103792,#59119,#59120);
#48828=AXIS2_PLACEMENT_3D('',#104545,#59121,#59122);
#48829=AXIS2_PLACEMENT_3D('',#105183,#59123,#59124);
#48830=AXIS2_PLACEMENT_3D('',#105184,#59125,#59126);
#48831=AXIS2_PLACEMENT_3D('',#105937,#59127,#59128);
#48832=AXIS2_PLACEMENT_3D('',#105940,#59129,#59130);
#48833=AXIS2_PLACEMENT_3D('',#105944,#59132,#59133);
#48834=AXIS2_PLACEMENT_3D('',#105946,#59135,#59136);
#48835=AXIS2_PLACEMENT_3D('',#105950,#59138,#59139);
#48836=AXIS2_PLACEMENT_3D('',#105955,#59142,#59143);
#48837=AXIS2_PLACEMENT_3D('',#105957,#59145,#59146);
#48838=AXIS2_PLACEMENT_3D('',#105960,#59147,#59148);
#48839=AXIS2_PLACEMENT_3D('',#105965,#59151,#59152);
#48840=AXIS2_PLACEMENT_3D('',#105968,#59155,#59156);
#48841=AXIS2_PLACEMENT_3D('',#105971,#59157,#59158);
#48842=AXIS2_PLACEMENT_3D('',#105975,#59160,#59161);
#48843=AXIS2_PLACEMENT_3D('',#105977,#59163,#59164);
#48844=AXIS2_PLACEMENT_3D('',#105980,#59167,#59168);
#48845=AXIS2_PLACEMENT_3D('',#105983,#59169,#59170);
#48846=AXIS2_PLACEMENT_3D('',#105986,#59173,#59174);
#48847=AXIS2_PLACEMENT_3D('',#105989,#59177,#59178);
#48848=AXIS2_PLACEMENT_3D('',#106028,#59183,#59184);
#48849=AXIS2_PLACEMENT_3D('',#106067,#59189,#59190);
#48850=AXIS2_PLACEMENT_3D('',#106117,#59191,#59192);
#48851=AXIS2_PLACEMENT_3D('',#106118,#59193,#59194);
#48852=AXIS2_PLACEMENT_3D('',#106198,#59195,#59196);
#48853=AXIS2_PLACEMENT_3D('',#106199,#59197,#59198);
#48854=AXIS2_PLACEMENT_3D('',#106200,#59199,#59200);
#48855=AXIS2_PLACEMENT_3D('',#106280,#59201,#59202);
#48856=AXIS2_PLACEMENT_3D('',#106336,#59203,#59204);
#48857=AXIS2_PLACEMENT_3D('',#106337,#59205,#59206);
#48858=AXIS2_PLACEMENT_3D('',#106338,#59207,#59208);
#48859=AXIS2_PLACEMENT_3D('',#106388,#59209,#59210);
#48860=AXIS2_PLACEMENT_3D('',#106389,#59211,#59212);
#48861=AXIS2_PLACEMENT_3D('',#106390,#59213,#59214);
#48862=AXIS2_PLACEMENT_3D('',#106391,#59215,#59216);
#48863=AXIS2_PLACEMENT_3D('',#106392,#59217,#59218);
#48864=AXIS2_PLACEMENT_3D('',#106433,#59219,#59220);
#48865=AXIS2_PLACEMENT_3D('',#106434,#59221,#59222);
#48866=AXIS2_PLACEMENT_3D('',#106435,#59223,#59224);
#48867=AXIS2_PLACEMENT_3D('',#106436,#59225,#59226);
#48868=AXIS2_PLACEMENT_3D('',#106437,#59227,#59228);
#48869=AXIS2_PLACEMENT_3D('',#106438,#59229,#59230);
#48870=AXIS2_PLACEMENT_3D('',#106439,#59231,#59232);
#48871=AXIS2_PLACEMENT_3D('',#106440,#59233,#59234);
#48872=AXIS2_PLACEMENT_3D('',#106483,#59235,#59236);
#48873=AXIS2_PLACEMENT_3D('',#106484,#59237,#59238);
#48874=AXIS2_PLACEMENT_3D('',#106485,#59239,#59240);
#48875=AXIS2_PLACEMENT_3D('',#106486,#59241,#59242);
#48876=AXIS2_PLACEMENT_3D('',#106487,#59243,#59244);
#48877=AXIS2_PLACEMENT_3D('',#106488,#59245,#59246);
#48878=AXIS2_PLACEMENT_3D('',#106489,#59247,#59248);
#48879=AXIS2_PLACEMENT_3D('',#106490,#59249,#59250);
#48880=AXIS2_PLACEMENT_3D('',#106491,#59251,#59252);
#48881=AXIS2_PLACEMENT_3D('',#106492,#59253,#59254);
#48882=AXIS2_PLACEMENT_3D('',#106493,#59255,#59256);
#48883=AXIS2_PLACEMENT_3D('',#106524,#59257,#59258);
#48884=AXIS2_PLACEMENT_3D('',#106525,#59259,#59260);
#48885=AXIS2_PLACEMENT_3D('',#106526,#59261,#59262);
#48886=AXIS2_PLACEMENT_3D('',#106527,#59263,#59264);
#48887=AXIS2_PLACEMENT_3D('',#106528,#59265,#59266);
#48888=AXIS2_PLACEMENT_3D('',#106529,#59267,#59268);
#48889=AXIS2_PLACEMENT_3D('',#106530,#59269,#59270);
#48890=AXIS2_PLACEMENT_3D('',#106573,#59271,#59272);
#48891=AXIS2_PLACEMENT_3D('',#106574,#59273,#59274);
#58960=DIRECTION('axis',(0.,0.,1.));
#58961=DIRECTION('refdir',(1.,0.,0.));
#58962=DIRECTION('center_axis',(1.,0.,0.));
#58963=DIRECTION('ref_axis',(0.,0.,-1.));
#58964=DIRECTION('center_axis',(1.,0.,0.));
#58965=DIRECTION('ref_axis',(0.,0.,-1.));
#58966=DIRECTION('center_axis',(1.,0.,0.));
#58967=DIRECTION('ref_axis',(0.,0.,-1.));
#58968=DIRECTION('center_axis',(0.,-1.,0.));
#58969=DIRECTION('ref_axis',(0.,0.,1.));
#58970=DIRECTION('center_axis',(1.,0.,0.));
#58971=DIRECTION('ref_axis',(0.,0.,-1.));
#58972=DIRECTION('center_axis',(0.,-1.,0.));
#58973=DIRECTION('ref_axis',(0.,0.,-1.));
#58974=DIRECTION('center_axis',(0.,1.,0.));
#58975=DIRECTION('ref_axis',(0.,0.,-1.));
#58976=DIRECTION('center_axis',(-0.666555993111408,0.,0.745454967149099));
#58977=DIRECTION('ref_axis',(0.745454967149099,0.,0.666555993111408));
#58978=DIRECTION('center_axis',(0.,-1.,0.));
#58979=DIRECTION('ref_axis',(0.,0.,-1.));
#58980=DIRECTION('center_axis',(-0.666555993111408,0.,-0.745454967149099));
#58981=DIRECTION('ref_axis',(0.745454967149099,0.,-0.666555993111408));
#58982=DIRECTION('center_axis',(0.,-1.,0.));
#58983=DIRECTION('ref_axis',(0.,0.,-1.));
#58984=DIRECTION('center_axis',(0.,1.,0.));
#58985=DIRECTION('ref_axis',(0.,0.,-1.));
#58986=DIRECTION('center_axis',(-0.666555993111408,0.,0.745454967149099));
#58987=DIRECTION('ref_axis',(0.745454967149099,0.,0.666555993111408));
#58988=DIRECTION('center_axis',(0.,-1.,0.));
#58989=DIRECTION('ref_axis',(0.,0.,-1.));
#58990=DIRECTION('center_axis',(-0.666555993111408,0.,-0.745454967149099));
#58991=DIRECTION('ref_axis',(0.745454967149099,0.,-0.666555993111408));
#58992=DIRECTION('center_axis',(1.,0.,0.));
#58993=DIRECTION('ref_axis',(0.,0.,-1.));
#58994=DIRECTION('center_axis',(-1.,0.,0.));
#58995=DIRECTION('ref_axis',(0.,0.,-1.));
#58996=DIRECTION('center_axis',(0.,0.,-1.));
#58997=DIRECTION('ref_axis',(-1.,0.,0.));
#58998=DIRECTION('center_axis',(1.,0.,0.));
#58999=DIRECTION('ref_axis',(0.,0.,-1.));
#59000=DIRECTION('center_axis',(0.,0.,1.));
#59001=DIRECTION('ref_axis',(1.,0.,0.));
#59002=DIRECTION('center_axis',(-1.,0.,0.));
#59003=DIRECTION('ref_axis',(0.,0.,-1.));
#59004=DIRECTION('center_axis',(-1.,0.,0.));
#59005=DIRECTION('ref_axis',(0.,0.,1.));
#59006=DIRECTION('',(1.,0.,0.));
#59007=DIRECTION('',(-1.,0.,0.));
#59008=DIRECTION('center_axis',(-1.,0.,1.56170177914177E-16));
#59009=DIRECTION('ref_axis',(-1.56170177914177E-16,0.,-1.));
#59010=DIRECTION('',(-1.,0.,0.));
#59011=DIRECTION('center_axis',(1.,0.,0.));
#59012=DIRECTION('ref_axis',(0.,0.,-1.));
#59013=DIRECTION('center_axis',(0.,-1.,0.));
#59014=DIRECTION('ref_axis',(0.,0.,1.));
#59015=DIRECTION('center_axis',(-1.,0.,0.));
#59016=DIRECTION('ref_axis',(0.,0.,-1.));
#59017=DIRECTION('center_axis',(-1.,0.,0.));
#59018=DIRECTION('ref_axis',(0.,0.,-1.));
#59019=DIRECTION('center_axis',(-1.,0.,0.));
#59020=DIRECTION('ref_axis',(0.,0.,1.));
#59021=DIRECTION('center_axis',(1.,0.,0.));
#59022=DIRECTION('ref_axis',(0.,0.,1.));
#59023=DIRECTION('center_axis',(0.,-1.,0.));
#59024=DIRECTION('ref_axis',(0.,0.,-1.));
#59025=DIRECTION('center_axis',(1.,0.,0.));
#59026=DIRECTION('ref_axis',(0.,0.,1.));
#59027=DIRECTION('center_axis',(-1.,0.,0.));
#59028=DIRECTION('ref_axis',(0.,0.,1.));
#59029=DIRECTION('',(1.,0.,0.));
#59030=DIRECTION('center_axis',(0.928966301520812,-0.281372335152031,0.240522804843608));
#59031=DIRECTION('ref_axis',(0.289882267482667,0.957062313017866,5.63993829393187E-15));
#59032=DIRECTION('center_axis',(-0.929823364809375,-0.279861066194094,-0.238969232084962));
#59033=DIRECTION('ref_axis',(0.2882113740593,-0.957566814307414,1.1677602810686E-14));
#59034=DIRECTION('center_axis',(-0.983705916475484,-0.132945851001502,0.121029213798216));
#59035=DIRECTION('ref_axis',(0.133930380500437,-0.990990743235782,1.03475023686325E-15));
#59036=DIRECTION('center_axis',(0.984136564099166,-0.131218424609742,-0.119402463316403));
#59037=DIRECTION('ref_axis',(0.132163933909845,0.991227872173434,-1.63884198414844E-15));
#59038=DIRECTION('center_axis',(0.999634880550771,-0.016329642943714,0.0215278505098936));
#59039=DIRECTION('ref_axis',(0.0215307213626423,4.0425685051786E-18,-0.999768187150204));
#59040=DIRECTION('center_axis',(-0.999680792908394,-0.01526908890116,-0.0201287658382933));
#59041=DIRECTION('ref_axis',(-0.0201311127099917,7.84436696756394E-18,0.999797348616737));
#59042=DIRECTION('center_axis',(0.000137653858420446,0.78765469274787,-0.616116925626681));
#59043=DIRECTION('ref_axis',(-0.000104683403461457,0.616116939438223,0.787654687016247));
#59044=DIRECTION('center_axis',(0.,-1.,0.));
#59045=DIRECTION('ref_axis',(0.,0.,1.));
#59046=DIRECTION('',(0.,-1.,0.));
#59047=DIRECTION('center_axis',(-0.000142617395615587,0.787779221568786,
0.615957691505477));
#59048=DIRECTION('ref_axis',(0.000106417131381098,0.615957706238014,-0.787779215771398));
#59049=DIRECTION('center_axis',(0.,-1.,0.));
#59050=DIRECTION('ref_axis',(0.,0.,1.));
#59051=DIRECTION('',(0.,1.,0.));
#59052=DIRECTION('center_axis',(0.285542519778965,-0.0955884964586558,0.953587074546972));
#59053=DIRECTION('ref_axis',(0.957973697650931,-3.97542076374563E-16,-0.28685605206968));
#59054=DIRECTION('center_axis',(-0.314704251896522,-0.0942607213325078,
-0.944497829670416));
#59055=DIRECTION('ref_axis',(-0.948721970571128,-5.65830961415102E-16,0.316111724799374));
#59056=DIRECTION('center_axis',(0.971123571857389,-0.158256544871534,0.178532557782247));
#59057=DIRECTION('ref_axis',(0.180811134609775,-8.5786423277988E-17,-0.983517835934421));
#59058=DIRECTION('center_axis',(-0.972285724910778,-0.155194176083419,-0.174857761750832));
#59059=DIRECTION('ref_axis',(-0.177002324580309,2.03190884905465E-16,0.984210433338911));
#59060=DIRECTION('center_axis',(-0.971123571857389,0.158256544871534,0.178532557782247));
#59061=DIRECTION('ref_axis',(0.180811134609775,-8.5786423277988E-17,0.983517835934421));
#59062=DIRECTION('center_axis',(0.972285724910778,0.155194176083419,-0.174857761750832));
#59063=DIRECTION('ref_axis',(-0.177002324580309,2.03190884905465E-16,-0.984210433338911));
#59064=DIRECTION('center_axis',(-1.,0.,0.));
#59065=DIRECTION('ref_axis',(0.,0.,1.));
#59066=DIRECTION('center_axis',(-1.,0.,0.));
#59067=DIRECTION('ref_axis',(0.,0.,1.));
#59068=DIRECTION('center_axis',(0.,-1.,0.));
#59069=DIRECTION('ref_axis',(0.,0.,-1.));
#59070=DIRECTION('center_axis',(1.,0.,0.));
#59071=DIRECTION('ref_axis',(0.,0.,-1.));
#59072=DIRECTION('center_axis',(1.,0.,0.));
#59073=DIRECTION('ref_axis',(0.,0.,-1.));
#59074=DIRECTION('center_axis',(1.,0.,0.));
#59075=DIRECTION('ref_axis',(0.,0.,-1.));
#59076=DIRECTION('center_axis',(0.,-1.,0.));
#59077=DIRECTION('ref_axis',(0.,0.,1.));
#59078=DIRECTION('center_axis',(-1.,0.,0.));
#59079=DIRECTION('ref_axis',(0.,0.,-1.));
#59080=DIRECTION('center_axis',(0.,1.,0.));
#59081=DIRECTION('ref_axis',(0.,0.,1.));
#59082=DIRECTION('',(0.,1.,0.));
#59083=DIRECTION('center_axis',(-1.,0.,0.));
#59084=DIRECTION('ref_axis',(0.,0.,1.));
#59085=DIRECTION('',(1.,0.,0.));
#59086=DIRECTION('center_axis',(0.928966301520812,0.281372335152031,0.240522804843608));
#59087=DIRECTION('ref_axis',(-0.289882267482667,0.957062313017866,-6.01031194250061E-15));
#59088=DIRECTION('center_axis',(-0.929823364809375,0.279861066194094,-0.238969232084962));
#59089=DIRECTION('ref_axis',(-0.2882113740593,-0.957566814307414,-1.12718317199366E-14));
#59090=DIRECTION('center_axis',(-0.983705916475484,0.132945851001502,0.121029213798216));
#59091=DIRECTION('ref_axis',(-0.133930380500437,-0.990990743235782,-1.03475023686325E-15));
#59092=DIRECTION('center_axis',(0.984136564099166,0.131218424609742,-0.119402463316403));
#59093=DIRECTION('ref_axis',(-0.132163933909845,0.991227872173434,1.63884198414844E-15));
#59094=DIRECTION('center_axis',(0.999634880550771,0.016329642943714,0.0215278505098936));
#59095=DIRECTION('ref_axis',(0.0215307213626423,-4.0425685051786E-18,-0.999768187150204));
#59096=DIRECTION('center_axis',(-0.000137653858420442,0.787654692747871,
0.616116925626681));
#59097=DIRECTION('ref_axis',(-0.000104683403375652,-0.616116939438222,0.787654687016248));
#59098=DIRECTION('center_axis',(-0.999680792908394,0.01526908890116,-0.0201287658382933));
#59099=DIRECTION('ref_axis',(-0.0201311127099917,-7.84436696756394E-18,
0.999797348616737));
#59100=DIRECTION('center_axis',(0.,1.,0.));
#59101=DIRECTION('ref_axis',(0.,0.,1.));
#59102=DIRECTION('',(0.,1.,0.));
#59103=DIRECTION('center_axis',(0.000142617394872601,0.787779221593475,
-0.615957691473901));
#59104=DIRECTION('ref_axis',(0.000106417135254732,-0.615957706206436,-0.787779215796088));
#59105=DIRECTION('center_axis',(0.,1.,0.));
#59106=DIRECTION('ref_axis',(0.,0.,1.));
#59107=DIRECTION('',(0.,-1.,0.));
#59108=DIRECTION('center_axis',(-1.24353895001492E-16,0.,-1.));
#59109=DIRECTION('ref_axis',(-1.,0.,1.24353895001492E-16));
#59110=DIRECTION('center_axis',(0.,0.,1.));
#59111=DIRECTION('ref_axis',(1.,0.,0.));
#59112=DIRECTION('center_axis',(-0.173648177666927,-0.984807753012209,0.));
#59113=DIRECTION('ref_axis',(0.984807753012209,-0.173648177666927,0.));
#59114=DIRECTION('',(0.173648177666927,0.984807753012209,0.));
#59115=DIRECTION('center_axis',(0.,-1.,0.));
#59116=DIRECTION('ref_axis',(0.,0.,-1.));
#59117=DIRECTION('center_axis',(-1.,0.,0.));
#59118=DIRECTION('ref_axis',(0.,0.,1.));
#59119=DIRECTION('center_axis',(-1.,0.,0.));
#59120=DIRECTION('ref_axis',(0.,0.,1.));
#59121=DIRECTION('center_axis',(1.,0.,0.));
#59122=DIRECTION('ref_axis',(0.,0.,-1.));
#59123=DIRECTION('center_axis',(-1.,0.,0.));
#59124=DIRECTION('ref_axis',(0.,0.,1.));
#59125=DIRECTION('center_axis',(-1.,0.,0.));
#59126=DIRECTION('ref_axis',(0.,0.,1.));
#59127=DIRECTION('center_axis',(0.,-1.,0.));
#59128=DIRECTION('ref_axis',(0.,0.,-1.));
#59129=DIRECTION('center_axis',(0.,-1.,0.));
#59130=DIRECTION('ref_axis',(0.,0.,-1.));
#59131=DIRECTION('',(0.,-1.,0.));
#59132=DIRECTION('center_axis',(0.,1.,0.));
#59133=DIRECTION('ref_axis',(0.,0.,-1.));
#59134=DIRECTION('',(0.,-1.,0.));
#59135=DIRECTION('center_axis',(0.,-1.,0.));
#59136=DIRECTION('ref_axis',(0.,0.,-1.));
#59137=DIRECTION('',(0.,0.,1.));
#59138=DIRECTION('center_axis',(0.,1.,0.));
#59139=DIRECTION('ref_axis',(0.,0.,-1.));
#59140=DIRECTION('',(0.,0.,-1.));
#59141=DIRECTION('',(1.56170177914177E-16,0.,1.));
#59142=DIRECTION('center_axis',(0.,1.,0.));
#59143=DIRECTION('ref_axis',(-8.10505695128492E-16,0.,-1.));
#59144=DIRECTION('',(0.,0.,-1.));
#59145=DIRECTION('center_axis',(0.,-1.,0.));
#59146=DIRECTION('ref_axis',(0.,0.,-1.));
#59147=DIRECTION('center_axis',(0.,-1.,0.));
#59148=DIRECTION('ref_axis',(0.,0.,-1.));
#59149=DIRECTION('',(0.,0.,-1.));
#59150=DIRECTION('',(0.,0.,1.));
#59151=DIRECTION('center_axis',(0.,-1.,0.));
#59152=DIRECTION('ref_axis',(0.,0.,-1.));
#59153=DIRECTION('',(-1.56170177914177E-16,0.,-1.));
#59154=DIRECTION('',(0.,0.,1.));
#59155=DIRECTION('center_axis',(0.,-1.,0.));
#59156=DIRECTION('ref_axis',(0.,0.,-1.));
#59157=DIRECTION('center_axis',(0.,1.,0.));
#59158=DIRECTION('ref_axis',(-7.65781678570401E-16,0.,-1.));
#59159=DIRECTION('',(0.,1.,0.));
#59160=DIRECTION('center_axis',(0.,-1.,0.));
#59161=DIRECTION('ref_axis',(0.,0.,-1.));
#59162=DIRECTION('',(0.,1.,0.));
#59163=DIRECTION('center_axis',(1.,0.,0.));
#59164=DIRECTION('ref_axis',(0.,0.,-1.));
#59165=DIRECTION('',(0.,0.,-1.));
#59166=DIRECTION('',(0.,0.,1.));
#59167=DIRECTION('center_axis',(1.,0.,-1.56170177914177E-16));
#59168=DIRECTION('ref_axis',(-1.56170177914177E-16,0.,-1.));
#59169=DIRECTION('center_axis',(1.,0.,-1.56170177914177E-16));
#59170=DIRECTION('ref_axis',(-1.56170177914177E-16,0.,-1.));
#59171=DIRECTION('',(1.56170177914177E-16,0.,1.));
#59172=DIRECTION('',(-1.56170177914177E-16,0.,-1.));
#59173=DIRECTION('center_axis',(0.,1.,0.));
#59174=DIRECTION('ref_axis',(1.22464679914735E-16,0.,-1.));
#59175=DIRECTION('',(0.,-1.,0.));
#59176=DIRECTION('',(0.,1.,0.));
#59177=DIRECTION('center_axis',(-1.,0.,0.));
#59178=DIRECTION('ref_axis',(0.,0.,1.));
#59179=DIRECTION('',(0.,0.,-1.));
#59180=DIRECTION('',(0.,-1.,0.));
#59181=DIRECTION('',(0.,0.,1.));
#59182=DIRECTION('',(0.,1.,0.));
#59183=DIRECTION('center_axis',(-1.,0.,0.));
#59184=DIRECTION('ref_axis',(0.,0.,1.));
#59185=DIRECTION('',(0.,0.,-1.));
#59186=DIRECTION('',(0.,1.,0.));
#59187=DIRECTION('',(0.,0.,1.));
#59188=DIRECTION('',(0.,-1.,0.));
#59189=DIRECTION('center_axis',(0.,-1.,0.));
#59190=DIRECTION('ref_axis',(0.,0.,-1.));
#59191=DIRECTION('center_axis',(0.,0.,-1.));
#59192=DIRECTION('ref_axis',(-1.,0.,0.));
#59193=DIRECTION('center_axis',(1.56170177914177E-16,0.,1.));
#59194=DIRECTION('ref_axis',(1.,0.,-1.56170177914177E-16));
#59195=DIRECTION('center_axis',(0.,0.431316910928101,-0.902200488997562));
#59196=DIRECTION('ref_axis',(0.,0.902200488997562,0.431316910928101));
#59197=DIRECTION('center_axis',(1.,0.,-1.56170177914177E-16));
#59198=DIRECTION('ref_axis',(0.,1.06001713493349E-14,1.));
#59199=DIRECTION('center_axis',(0.,0.431316910928101,0.902200488997562));
#59200=DIRECTION('ref_axis',(0.,-0.902200488997562,0.431316910928101));
#59201=DIRECTION('center_axis',(0.,-1.,0.));
#59202=DIRECTION('ref_axis',(0.,0.,-1.));
#59203=DIRECTION('center_axis',(0.,0.,-1.));
#59204=DIRECTION('ref_axis',(-1.,0.,0.));
#59205=DIRECTION('center_axis',(-1.56170177914177E-16,0.,-1.));
#59206=DIRECTION('ref_axis',(-1.,0.,1.56170177914177E-16));
#59207=DIRECTION('center_axis',(0.,-1.,0.));
#59208=DIRECTION('ref_axis',(0.,0.,-1.));
#59209=DIRECTION('center_axis',(0.,0.,-1.));
#59210=DIRECTION('ref_axis',(-1.,0.,0.));
#59211=DIRECTION('center_axis',(0.,0.,1.));
#59212=DIRECTION('ref_axis',(1.,0.,0.));
#59213=DIRECTION('center_axis',(0.,0.,-1.));
#59214=DIRECTION('ref_axis',(-1.,0.,0.));
#59215=DIRECTION('center_axis',(0.,0.,1.));
#59216=DIRECTION('ref_axis',(1.,0.,0.));
#59217=DIRECTION('center_axis',(0.,-1.,0.));
#59218=DIRECTION('ref_axis',(0.,0.,-1.));
#59219=DIRECTION('center_axis',(0.,1.,0.));
#59220=DIRECTION('ref_axis',(0.,0.,1.));
#59221=DIRECTION('center_axis',(0.,0.,-1.));
#59222=DIRECTION('ref_axis',(-1.,0.,0.));
#59223=DIRECTION('center_axis',(0.,0.,1.));
#59224=DIRECTION('ref_axis',(1.,0.,0.));
#59225=DIRECTION('center_axis',(0.,0.,-1.));
#59226=DIRECTION('ref_axis',(-1.,0.,0.));
#59227=DIRECTION('center_axis',(0.,-1.,0.));
#59228=DIRECTION('ref_axis',(0.480804881866777,0.,0.876827614513295));
#59229=DIRECTION('center_axis',(0.,1.,0.));
#59230=DIRECTION('ref_axis',(0.,0.,1.));
#59231=DIRECTION('center_axis',(0.,1.,0.));
#59232=DIRECTION('ref_axis',(1.,0.,0.));
#59233=DIRECTION('center_axis',(0.,1.,0.));
#59234=DIRECTION('ref_axis',(0.,0.,-1.));
#59235=DIRECTION('center_axis',(0.,0.,-1.));
#59236=DIRECTION('ref_axis',(-1.,0.,0.));
#59237=DIRECTION('center_axis',(0.,1.,0.));
#59238=DIRECTION('ref_axis',(0.,0.,1.));
#59239=DIRECTION('center_axis',(0.,1.,0.));
#59240=DIRECTION('ref_axis',(0.,0.,1.));
#59241=DIRECTION('center_axis',(0.,0.,1.));
#59242=DIRECTION('ref_axis',(1.,0.,0.));
#59243=DIRECTION('center_axis',(0.,0.,-1.));
#59244=DIRECTION('ref_axis',(-1.,0.,0.));
#59245=DIRECTION('center_axis',(0.,0.,-1.));
#59246=DIRECTION('ref_axis',(-1.,0.,0.));
#59247=DIRECTION('center_axis',(0.,0.,-1.));
#59248=DIRECTION('ref_axis',(-1.,0.,0.));
#59249=DIRECTION('center_axis',(0.,0.,1.));
#59250=DIRECTION('ref_axis',(1.,0.,0.));
#59251=DIRECTION('center_axis',(0.,1.,0.));
#59252=DIRECTION('ref_axis',(1.,0.,0.));
#59253=DIRECTION('center_axis',(0.,1.,0.));
#59254=DIRECTION('ref_axis',(0.,0.,-1.));
#59255=DIRECTION('center_axis',(0.,1.,0.));
#59256=DIRECTION('ref_axis',(1.,0.,0.));
#59257=DIRECTION('center_axis',(0.,1.,0.));
#59258=DIRECTION('ref_axis',(0.,0.,1.));
#59259=DIRECTION('center_axis',(0.,1.,0.));
#59260=DIRECTION('ref_axis',(0.,0.,1.));
#59261=DIRECTION('center_axis',(0.,1.,0.));
#59262=DIRECTION('ref_axis',(0.,0.,1.));
#59263=DIRECTION('center_axis',(0.,-1.,0.));
#59264=DIRECTION('ref_axis',(-0.48080488186677,0.,0.876827614513298));
#59265=DIRECTION('center_axis',(0.,1.,0.));
#59266=DIRECTION('ref_axis',(0.,0.,1.));
#59267=DIRECTION('center_axis',(0.,1.,0.));
#59268=DIRECTION('ref_axis',(1.,0.,0.));
#59269=DIRECTION('center_axis',(0.,0.,1.));
#59270=DIRECTION('ref_axis',(-1.,0.,0.));
#59271=DIRECTION('center_axis',(0.,0.,-1.));
#59272=DIRECTION('ref_axis',(-1.,0.,0.));
#59273=DIRECTION('center_axis',(0.,0.,-1.));
#59274=DIRECTION('ref_axis',(-1.,0.,0.));
#97280=CARTESIAN_POINT('',(0.,0.,0.));
#97281=CARTESIAN_POINT('Origin',(24.5,620.675373764374,64.2994740882088));
#97282=CARTESIAN_POINT('',(24.5,620.675373764374,44.8494740882089));
#97283=CARTESIAN_POINT('',(24.5,620.675373764374,83.7494740882087));
#97284=CARTESIAN_POINT('Origin',(24.5,620.675373764374,64.2994740882088));
#97285=CARTESIAN_POINT('Origin',(24.5,620.675373764374,64.2994740882088));
#97286=CARTESIAN_POINT('',(24.,620.675373764374,83.2494740882088));
#97287=CARTESIAN_POINT('Origin',(24.5,620.675373764374,83.2494740882087));
#97288=CARTESIAN_POINT('Origin',(24.,620.675373764374,64.2994740882088));
#97289=CARTESIAN_POINT('Origin',(52.8776183915471,639.625373764374,90.6087118617898));
#97290=CARTESIAN_POINT('',(61.9796230824862,639.625373764374,98.7473601281983));
#97291=CARTESIAN_POINT('',(43.775613700608,639.625373764374,98.7473601281983));
#97292=CARTESIAN_POINT('Origin',(52.8776183915471,639.625373764374,90.6087118617898));
#97293=CARTESIAN_POINT('',(62.3523505660608,640.125373764374,99.080638124754));
#97294=CARTESIAN_POINT('Origin',(62.3523505660608,639.625373764374,99.080638124754));
#97295=CARTESIAN_POINT('',(43.4028862170334,640.125373764374,99.080638124754));
#97296=CARTESIAN_POINT('Origin',(52.8776183915471,640.125373764374,90.6087118617898));
#97297=CARTESIAN_POINT('Origin',(43.4028862170334,639.625373764374,99.080638124754));
#97298=CARTESIAN_POINT('Origin',(52.8776183915471,601.725373764374,90.6087118617898));
#97299=CARTESIAN_POINT('',(62.3523505660608,601.225373764374,99.080638124754));
#97300=CARTESIAN_POINT('',(43.4028862170334,601.225373764374,99.080638124754));
#97301=CARTESIAN_POINT('Origin',(52.8776183915471,601.225373764374,90.6087118617898));
#97302=CARTESIAN_POINT('',(61.9796230824862,601.725373764374,98.7473601281983));
#97303=CARTESIAN_POINT('Origin',(62.3523505660608,601.725373764374,99.080638124754));
#97304=CARTESIAN_POINT('',(43.775613700608,601.725373764374,98.7473601281983));
#97305=CARTESIAN_POINT('Origin',(52.8776183915471,601.725373764374,90.6087118617898));
#97306=CARTESIAN_POINT('Origin',(43.4028862170334,601.725373764374,99.080638124754));
#97307=CARTESIAN_POINT('Origin',(70.,620.675373764374,64.2994740882088));
#97308=CARTESIAN_POINT('',(70.,640.125373764374,64.2994740882088));
#97309=CARTESIAN_POINT('',(70.,620.675373764374,44.8494740882089));
#97310=CARTESIAN_POINT('Origin',(70.,620.675373764374,64.2994740882088));
#97311=CARTESIAN_POINT('',(71.,639.125373764374,64.2994740882088));
#97312=CARTESIAN_POINT('Origin',(70.,639.125373764374,64.2994740882088));
#97313=CARTESIAN_POINT('',(71.,602.225373764374,64.2994740882088));
#97314=CARTESIAN_POINT('Origin',(71.,620.675373764374,64.2994740882088));
#97315=CARTESIAN_POINT('',(70.,601.225373764374,64.2994740882088));
#97316=CARTESIAN_POINT('Origin',(70.,602.225373764374,64.2994740882088));
#97317=CARTESIAN_POINT('Origin',(70.,620.675373764374,64.2994740882088));
#97318=CARTESIAN_POINT('Origin',(71.,620.675373764374,64.2994740882088));
#97319=CARTESIAN_POINT('',(71.,620.675373764374,44.8494740882089));
#97320=CARTESIAN_POINT('',(35.7552367830941,601.225373764374,64.2994740882088));
#97321=CARTESIAN_POINT('',(71.,601.225373764374,64.2994740882088));
#97322=CARTESIAN_POINT('',(33.7552367830941,603.127574253371,72.6885880057606));
#97323=CARTESIAN_POINT('Ctrl Pts',(35.7552367830941,601.225373764374,64.2994740882088));
#97324=CARTESIAN_POINT('Ctrl Pts',(35.6257365591854,601.225373764374,64.6933227733964));
#97325=CARTESIAN_POINT('Ctrl Pts',(35.4961078469376,601.237366261793,65.0875125516637));
#97326=CARTESIAN_POINT('Ctrl Pts',(35.3683280852255,601.261325958332,65.4811925716977));
#97327=CARTESIAN_POINT('Ctrl Pts',(35.2659632064297,601.280520167174,65.7965712122205));
#97328=CARTESIAN_POINT('Ctrl Pts',(35.164784366186,601.307395533574,66.1116230291669));
#97329=CARTESIAN_POINT('Ctrl Pts',(35.0658114313479,601.341963007925,66.425909717438));
#97330=CARTESIAN_POINT('Ctrl Pts',(35.0654326493907,601.342095302027,66.4271125324004));
#97331=CARTESIAN_POINT('Ctrl Pts',(35.0650539000296,601.342227708726,66.4283153352887));
#97332=CARTESIAN_POINT('Ctrl Pts',(35.0646751833233,601.342360228022,66.4295181260736));
#97333=CARTESIAN_POINT('Ctrl Pts',(34.9032152398727,601.39885775679,66.9423091618597));
#97334=CARTESIAN_POINT('Ctrl Pts',(34.7473679169488,601.47569378957,67.4534199949505));
#97335=CARTESIAN_POINT('Ctrl Pts',(34.6015663494618,601.573679242807,67.9640147041513));
#97336=CARTESIAN_POINT('Ctrl Pts',(34.5468057526337,601.610480917798,68.1557854203037));
#97337=CARTESIAN_POINT('Ctrl Pts',(34.4934625501783,601.650266373644,68.347483350911));
#97338=CARTESIAN_POINT('Ctrl Pts',(34.441772953152,601.693080009916,68.539170305048));
#97339=CARTESIAN_POINT('Ctrl Pts',(34.4412715863034,601.693495283765,68.5410295860184));
#97340=CARTESIAN_POINT('Ctrl Pts',(34.4407703749893,601.693910842595,68.5428888663075));
#97341=CARTESIAN_POINT('Ctrl Pts',(34.4402693194284,601.694326686444,68.544748145963));
#97342=CARTESIAN_POINT('Ctrl Pts',(34.2998573245699,601.810859600235,69.0657785182523));
#97343=CARTESIAN_POINT('Ctrl Pts',(34.1716160470563,601.950101647865,69.5868210918051));
#97344=CARTESIAN_POINT('Ctrl Pts',(34.064487473247,602.111405838435,70.1029417803957));
#97345=CARTESIAN_POINT('Ctrl Pts',(34.0274026664021,602.167244673377,70.2816078016488));
#97346=CARTESIAN_POINT('Ctrl Pts',(33.9928482010104,602.225727031641,70.4596837544423));
#97347=CARTESIAN_POINT('Ctrl Pts',(33.9611958099703,602.286825206801,70.6369642677272));
#97348=CARTESIAN_POINT('Ctrl Pts',(33.9609301528875,602.287338001015,70.638452175037));
#97349=CARTESIAN_POINT('Ctrl Pts',(33.9606647001835,602.287850979633,70.6399400267307));
#97350=CARTESIAN_POINT('Ctrl Pts',(33.9603994520774,602.288364142641,70.6414278226942));
#97351=CARTESIAN_POINT('Ctrl Pts',(33.8988854931898,602.407372299352,70.986464102381));
#97352=CARTESIAN_POINT('Ctrl Pts',(33.8482365019429,602.536496470251,71.3293804030283));
#97353=CARTESIAN_POINT('Ctrl Pts',(33.8123513013975,602.676232077861,71.6705933077606));
#97354=CARTESIAN_POINT('Ctrl Pts',(33.7806037130973,602.799855980581,71.9724639022542));
#97355=CARTESIAN_POINT('Ctrl Pts',(33.7602910819696,602.931779777438,72.2730015582567));
#97356=CARTESIAN_POINT('Ctrl Pts',(33.7560607839295,603.072602503069,72.57262184915));
#97357=CARTESIAN_POINT('Ctrl Pts',(33.7555148022906,603.090777728977,72.611292216089));
#97358=CARTESIAN_POINT('Ctrl Pts',(33.7552367835934,603.109101210383,72.6499473033098));
#97359=CARTESIAN_POINT('Ctrl Pts',(33.7552367830941,603.127574253371,72.6885880057606));
#97360=CARTESIAN_POINT('',(33.7552367830941,638.223173275376,72.6885880057604));
#97361=CARTESIAN_POINT('Origin',(33.7552367830941,620.675373764374,64.2994740882088));
#97362=CARTESIAN_POINT('',(35.7552367830941,640.125373764374,64.2994740882088));
#97363=CARTESIAN_POINT('Ctrl Pts',(33.7552367830941,638.223173275376,72.6885880057604));
#97364=CARTESIAN_POINT('Ctrl Pts',(33.7552367869584,638.366316942016,72.3891694511719));
#97365=CARTESIAN_POINT('Ctrl Pts',(33.7719257417031,638.500481620589,72.0888870509365));
#97366=CARTESIAN_POINT('Ctrl Pts',(33.8006485106675,638.626268389842,71.7873250236769));
#97367=CARTESIAN_POINT('Ctrl Pts',(33.8043525567342,638.642489666713,71.7484360279008));
#97368=CARTESIAN_POINT('Ctrl Pts',(33.808256796361,638.658571596475,71.7095257528911));
#97369=CARTESIAN_POINT('Ctrl Pts',(33.8123513034981,638.674515450813,71.6705933079404));
#97370=CARTESIAN_POINT('Ctrl Pts',(33.8482365102383,638.814251074653,71.3293803635857));
#97371=CARTESIAN_POINT('Ctrl Pts',(33.8988855120037,638.943375249915,70.9864640427555));
#97372=CARTESIAN_POINT('Ctrl Pts',(33.9603994665039,639.062383385352,70.6414278248801));
#97373=CARTESIAN_POINT('Ctrl Pts',(33.960667679382,639.062902284109,70.6399233994569));
#97374=CARTESIAN_POINT('Ctrl Pts',(33.9609361014569,639.06342099433,70.6384189170522));
#97375=CARTESIAN_POINT('Ctrl Pts',(33.9612047325023,639.063939516001,70.6369143777839));
#97376=CARTESIAN_POINT('Ctrl Pts',(34.0526561269075,639.240462411137,70.1247166389886));
#97377=CARTESIAN_POINT('Ctrl Pts',(34.168330227834,639.395147745896,69.6058806834539));
#97378=CARTESIAN_POINT('Ctrl Pts',(34.2992699048925,639.527337269571,69.0853523891265));
#97379=CARTESIAN_POINT('Ctrl Pts',(34.3445659440352,639.573065668885,68.9052857315297));
#97380=CARTESIAN_POINT('Ctrl Pts',(34.3916890276511,639.616102313696,68.7250163402484));
#97381=CARTESIAN_POINT('Ctrl Pts',(34.440269340592,639.656420841148,68.5447481511289));
#97382=CARTESIAN_POINT('Ctrl Pts',(34.4407795157771,639.656844253658,68.5428550312376));
#97383=CARTESIAN_POINT('Ctrl Pts',(34.4412898524366,639.657267370677,68.5409619106906));
#97384=CARTESIAN_POINT('Ctrl Pts',(34.4418003503396,639.657690192248,68.5390687894377));
#97385=CARTESIAN_POINT('Ctrl Pts',(34.5794751777585,639.771719821878,68.0285179325883));
#97386=CARTESIAN_POINT('Ctrl Pts',(34.7288776165414,639.864270380756,67.5178887275615));
#97387=CARTESIAN_POINT('Ctrl Pts',(34.8855569182322,639.93616826794,67.006014915324));
#97388=CARTESIAN_POINT('Ctrl Pts',(34.9443169906728,639.96313242347,66.8140448084693));
#97389=CARTESIAN_POINT('Ctrl Pts',(35.0041009383194,639.987191371054,66.6218996870685));
#97390=CARTESIAN_POINT('Ctrl Pts',(35.0646751529483,640.008387301716,66.4295181170863));
#97391=CARTESIAN_POINT('Ctrl Pts',(35.0650699280554,640.008525440127,66.4282643252648));
#97392=CARTESIAN_POINT('Ctrl Pts',(35.0654647386451,640.008663456191,66.4270105202926));
#97393=CARTESIAN_POINT('Ctrl Pts',(35.0658595846507,640.008801349907,66.4257567022029));
#97394=CARTESIAN_POINT('Ctrl Pts',(35.1771223453717,640.047658107464,66.0724461454543));
#97395=CARTESIAN_POINT('Ctrl Pts',(35.2912445666128,640.076808508222,65.7179802822932));
#97396=CARTESIAN_POINT('Ctrl Pts',(35.4066366929697,640.09623524223,65.3633493527697));
#97397=CARTESIAN_POINT('Ctrl Pts',(35.4643327561481,640.105948609234,65.186033888008));
#97398=CARTESIAN_POINT('Ctrl Pts',(35.5223291503942,640.113230342378,65.0087318398257));
#97399=CARTESIAN_POINT('Ctrl Pts',(35.5804869830593,640.118087133712,64.831397796837));
#97400=CARTESIAN_POINT('Ctrl Pts',(35.6150978613504,640.120977506445,64.7258627949723));
#97401=CARTESIAN_POINT('Ctrl Pts',(35.6499102657678,640.123016256969,64.6198773927215));
#97402=CARTESIAN_POINT('Ctrl Pts',(35.6846226908027,640.124185031716,64.5142623497308));
#97403=CARTESIAN_POINT('Ctrl Pts',(35.7082387308706,640.124980188817,64.4424088539142));
#97404=CARTESIAN_POINT('Ctrl Pts',(35.7318083908217,640.125373764374,64.3707267948586));
#97405=CARTESIAN_POINT('Ctrl Pts',(35.7552367830941,640.125373764374,64.2994740882088));
#97406=CARTESIAN_POINT('',(71.,640.125373764374,64.2994740882088));
#97407=CARTESIAN_POINT('Origin',(23.5,620.675373764374,64.2994740882088));
#97408=CARTESIAN_POINT('',(23.5,620.675373764374,83.7494740882088));
#97409=CARTESIAN_POINT('Origin',(23.5,620.675373764374,83.2494740882088));
#97410=CARTESIAN_POINT('',(23.5,620.675373764374,44.8494740882088));
#97411=CARTESIAN_POINT('Origin',(23.5,620.675373764374,64.2994740882088));
#97412=CARTESIAN_POINT('Origin',(23.5,620.675373764374,64.2994740882088));
#97413=CARTESIAN_POINT('Origin',(22.5,620.675373764374,64.2994740882088));
#97414=CARTESIAN_POINT('',(22.,620.675373764374,45.3494740882088));
#97415=CARTESIAN_POINT('Origin',(22.,620.675373764374,64.2994740882088));
#97416=CARTESIAN_POINT('',(22.5,620.675373764374,44.8494740882088));
#97417=CARTESIAN_POINT('Origin',(22.5,620.675373764374,45.3494740882088));
#97418=CARTESIAN_POINT('Origin',(22.5,620.675373764374,64.2994740882088));
#97419=CARTESIAN_POINT('Origin',(22.,620.675373764374,64.2994740882088));
#97420=CARTESIAN_POINT('',(22.,620.675373764374,44.8494740882088));
#97421=CARTESIAN_POINT('Ctrl Pts',(-4.46675582290381,607.708350351965,79.3699798038647));
#97422=CARTESIAN_POINT('Ctrl Pts',(-4.65179838528775,608.301384168068,79.3159462734029));
#97423=CARTESIAN_POINT('Ctrl Pts',(-4.39560350684042,607.872719845594,78.941911814982));
#97424=CARTESIAN_POINT('Ctrl Pts',(-3.27436645786458,608.106096967698,79.722255531378));
#97425=CARTESIAN_POINT('Ctrl Pts',(-3.35828013221585,608.779842649617,79.710778768012));
#97426=CARTESIAN_POINT('Ctrl Pts',(-3.22222729142889,608.265397557493,79.2841755866817));
#97427=CARTESIAN_POINT('Ctrl Pts',(-2.0401534841229,608.377157746436,79.9382527125226));
#97428=CARTESIAN_POINT('Ctrl Pts',(-2.13704517638702,609.079904904266,79.9301149240667));
#97429=CARTESIAN_POINT('Ctrl Pts',(-2.00765458360655,608.533014332571,79.4940431330354));
#97430=CARTESIAN_POINT('Ctrl Pts',(-0.477078115453726,608.470043666149,
80.0129132419871));
#97431=CARTESIAN_POINT('Ctrl Pts',(-0.504033715610802,609.190797807749,
80.0123807664004));
#97432=CARTESIAN_POINT('Ctrl Pts',(-0.46947699470708,608.624717782472,79.5665829488807));
#97433=CARTESIAN_POINT('Ctrl Pts',(-0.201739610759609,608.477464067233,
80.018847964929));
#97434=CARTESIAN_POINT('Ctrl Pts',(-0.213567627251543,609.199734125483,
80.0189726826106));
#97435=CARTESIAN_POINT('Ctrl Pts',(-0.198525207359669,608.632043701841,
79.5723490852243));
#97436=CARTESIAN_POINT('Ctrl Pts',(0.343267231354877,608.474402475761,80.016394319429));
#97437=CARTESIAN_POINT('Ctrl Pts',(0.363172475404081,609.19602915895,80.0162332785399));
#97438=CARTESIAN_POINT('Ctrl Pts',(0.337797886426132,608.629021099499,79.569965145871));
#97439=CARTESIAN_POINT('Ctrl Pts',(0.614288243293599,608.464030193296,80.0080931677934));
#97440=CARTESIAN_POINT('Ctrl Pts',(0.648999446052346,609.183542498368,80.0070154560597));
#97441=CARTESIAN_POINT('Ctrl Pts',(0.604500980807282,608.618780884095,79.5618998035947));
#97442=CARTESIAN_POINT('Ctrl Pts',(1.42305709514243,608.407424943048,79.9625420908729));
#97443=CARTESIAN_POINT('Ctrl Pts',(1.49988036818683,609.115508961494,79.9564789876385));
#97444=CARTESIAN_POINT('Ctrl Pts',(1.40038494278016,608.562896395885,79.5176427201739));
#97445=CARTESIAN_POINT('Ctrl Pts',(1.95650990903739,608.335644777334,79.9047081360849));
#97446=CARTESIAN_POINT('Ctrl Pts',(2.05434637538844,609.030990740555,79.8936395733644));
#97447=CARTESIAN_POINT('Ctrl Pts',(1.92534113326012,608.492029675597,79.4614512450883));
#97448=CARTESIAN_POINT('Ctrl Pts',(2.74875593427252,608.182424012343,79.777879100916));
#97449=CARTESIAN_POINT('Ctrl Pts',(2.8863399589135,608.8483829158,79.7536174784857));
#97450=CARTESIAN_POINT('Ctrl Pts',(2.70496406063899,608.340760187158,79.3382254829299));
#97451=CARTESIAN_POINT('Ctrl Pts',(3.01256338076222,608.12349345016,79.7286663835033));
#97452=CARTESIAN_POINT('Ctrl Pts',(3.15905718679442,608.779515695899,79.700294762995));
#97453=CARTESIAN_POINT('Ctrl Pts',(2.96456958631009,608.282579746035,79.290410633663));
#97454=CARTESIAN_POINT('Ctrl Pts',(3.53144620093892,607.993176826927,79.6182338532211));
#97455=CARTESIAN_POINT('Ctrl Pts',(3.69386701621685,608.627862943539,79.5809202469059));
#97456=CARTESIAN_POINT('Ctrl Pts',(3.47518780032947,608.153921993654,79.1831150315862));
#97457=CARTESIAN_POINT('Ctrl Pts',(3.78653130909377,607.921879230461,79.5570911547537));
#97458=CARTESIAN_POINT('Ctrl Pts',(3.95514895647901,608.545755658182,79.5154433630724));
#97459=CARTESIAN_POINT('Ctrl Pts',(3.72621041294374,608.083531812044,79.1237090131227));
#97460=CARTESIAN_POINT('Ctrl Pts',(4.54004264997885,607.69222741958,79.3568092233317));
#97461=CARTESIAN_POINT('Ctrl Pts',(4.71519034053281,608.285724795436,79.3041392307202));
#97462=CARTESIAN_POINT('Ctrl Pts',(4.46772555015823,607.856801716605,78.9291150218727));
#97463=CARTESIAN_POINT('Ctrl Pts',(5.02678739774566,607.518206712822,79.2008962492214));
#97464=CARTESIAN_POINT('Ctrl Pts',(5.20619063282509,608.090787346965,79.1411907055206));
#97465=CARTESIAN_POINT('Ctrl Pts',(4.94672040811002,607.684994790463,78.7776297759102));
#97466=CARTESIAN_POINT('Ctrl Pts',(5.97439705300667,607.139979558517,78.8468983899839));
#97467=CARTESIAN_POINT('Ctrl Pts',(6.15788846175844,607.669560635868,78.7714177057809));
#97468=CARTESIAN_POINT('Ctrl Pts',(5.87924293219311,607.311580055514,78.4336864380197));
#97469=CARTESIAN_POINT('Ctrl Pts',(6.43524462113633,606.935745723925,78.6487931851204));
#97470=CARTESIAN_POINT('Ctrl Pts',(6.6170133392223,607.446118460456,78.5679319403425));
#97471=CARTESIAN_POINT('Ctrl Pts',(6.33275437617335,607.109943925485,78.241207083469));
#97472=CARTESIAN_POINT('Ctrl Pts',(7.33453041364423,606.506055797746,78.2106205359385));
#97473=CARTESIAN_POINT('Ctrl Pts',(7.50949169824814,606.978742271419,78.1180713169069));
#97474=CARTESIAN_POINT('Ctrl Pts',(7.21772555207048,606.685719938611,77.8154792735));
#97475=CARTESIAN_POINT('Ctrl Pts',(7.76940426542435,606.282236687675,77.9721240183561));
#97476=CARTESIAN_POINT('Ctrl Pts',(7.93961757498883,606.73810424419,77.8759092393284));
#97477=CARTESIAN_POINT('Ctrl Pts',(7.64567757896694,606.464747461961,77.5837558363346));
#97478=CARTESIAN_POINT('Ctrl Pts',(9.0235661087087,605.602041993258,77.2068280660124));
#97479=CARTESIAN_POINT('Ctrl Pts',(9.14486309090703,606.028967316258,77.1186234238837));
#97480=CARTESIAN_POINT('Ctrl Pts',(8.87989624832361,605.793194699699,76.8401851017735));
#97481=CARTESIAN_POINT('Ctrl Pts',(9.79898624522685,605.134564116264,76.6280570123386));
#97482=CARTESIAN_POINT('Ctrl Pts',(9.91195517002788,605.535098232726,76.5412806704512));
#97483=CARTESIAN_POINT('Ctrl Pts',(9.6429736636773,605.331661990879,76.277848672361));
#97484=CARTESIAN_POINT('Ctrl Pts',(10.8844475000821,604.443294288982,75.6498569210074));
#97485=CARTESIAN_POINT('Ctrl Pts',(10.996929204677,604.796890866984,75.5414473133398));
#97486=CARTESIAN_POINT('Ctrl Pts',(10.7111493226909,604.649191799515,75.3274439525344));
#97487=CARTESIAN_POINT('Ctrl Pts',(11.2331134421883,604.214386386114,75.3052878963191));
#97488=CARTESIAN_POINT('Ctrl Pts',(11.3383050337577,604.558413915678,75.1981903967951));
#97489=CARTESIAN_POINT('Ctrl Pts',(11.0542671299848,604.423194954832,74.9926611496337));
#97490=CARTESIAN_POINT('Ctrl Pts',(11.9041426976532,603.763841215211,74.5757653364059));
#97491=CARTESIAN_POINT('Ctrl Pts',(11.9934013858358,604.091098654978,74.4717373421274));
#97492=CARTESIAN_POINT('Ctrl Pts',(11.7146199608134,603.978379024213,74.2838589448406));
#97493=CARTESIAN_POINT('Ctrl Pts',(12.2226419987782,603.544786801835,74.1948314957367));
#97494=CARTESIAN_POINT('Ctrl Pts',(12.3052838069643,603.86393368874,74.0929439227344));
#97495=CARTESIAN_POINT('Ctrl Pts',(12.0280511690333,603.762110554936,73.9137447966116));
#97496=CARTESIAN_POINT('Ctrl Pts',(13.1218292556881,602.915923230929,73.0096082212392));
#97497=CARTESIAN_POINT('Ctrl Pts',(13.1682069587253,603.225589567109,72.9350760877258));
#97498=CARTESIAN_POINT('Ctrl Pts',(12.9129429279531,603.141236478736,72.7621724811206));
#97499=CARTESIAN_POINT('Ctrl Pts',(13.6498656696272,602.532207939341,72.1603061192183));
#97500=CARTESIAN_POINT('Ctrl Pts',(13.691058719412,602.826004591238,72.0905203676822));
#97501=CARTESIAN_POINT('Ctrl Pts',(13.4325731745126,602.762404239833,71.9369957714403));
#97502=CARTESIAN_POINT('Ctrl Pts',(14.3276327741606,602.031260936065,70.7837383555535));
#97503=CARTESIAN_POINT('Ctrl Pts',(14.3599543505595,602.306311131027,70.7113989853479));
#97504=CARTESIAN_POINT('Ctrl Pts',(14.0995518794942,602.267831951347,70.5995413985153));
#97505=CARTESIAN_POINT('Ctrl Pts',(14.5343332153866,601.876752255328,70.3076585181821));
#97506=CARTESIAN_POINT('Ctrl Pts',(14.5622961369223,602.147552358501,70.2399143740041));
#97507=CARTESIAN_POINT('Ctrl Pts',(14.3029634008898,602.115288534774,70.136985137629));
#97508=CARTESIAN_POINT('Ctrl Pts',(14.9054756223491,601.597383091018,69.3166364965849));
#97509=CARTESIAN_POINT('Ctrl Pts',(14.9241336165254,601.861845857833,69.2600256603411));
#97510=CARTESIAN_POINT('Ctrl Pts',(14.6682015611194,601.839471988102,69.174113632982));
#97511=CARTESIAN_POINT('Ctrl Pts',(15.0666029583495,601.475024328722,68.8100615928647));
#97512=CARTESIAN_POINT('Ctrl Pts',(15.0820212400289,601.736215094156,68.7582297164531));
#97513=CARTESIAN_POINT('Ctrl Pts',(14.8267650211877,601.718669700196,68.6819292751414));
#97514=CARTESIAN_POINT('Ctrl Pts',(15.3369981776382,601.268803317671,67.781486615588));
#97515=CARTESIAN_POINT('Ctrl Pts',(15.345642317407,601.525631362788,67.7418790685988));
#97516=CARTESIAN_POINT('Ctrl Pts',(15.0928587745384,601.51507115203,67.6825720627153));
#97517=CARTESIAN_POINT('Ctrl Pts',(15.4467037685615,601.184606480853,67.2583447276789));
#97518=CARTESIAN_POINT('Ctrl Pts',(15.4531593768323,601.439270686425,67.2238371821344));
#97519=CARTESIAN_POINT('Ctrl Pts',(15.2008187183865,601.431945381811,67.1742916843792));
#97520=CARTESIAN_POINT('Ctrl Pts',(15.5714893985198,601.088632207677,66.4596770533946));
#97521=CARTESIAN_POINT('Ctrl Pts',(15.5750769362233,601.341153963858,66.4333318182824));
#97522=CARTESIAN_POINT('Ctrl Pts',(15.3236190583423,601.337191765776,66.3983126284387));
#97523=CARTESIAN_POINT('Ctrl Pts',(15.6064418001331,601.06170107286,66.191124442761));
#97524=CARTESIAN_POINT('Ctrl Pts',(15.6092008209444,601.313647862235,66.1679286147603));
#97525=CARTESIAN_POINT('Ctrl Pts',(15.3580154032569,601.310603141948,66.1373887935008));
#97526=CARTESIAN_POINT('Ctrl Pts',(15.6626190527797,601.018381804667,65.649189292362));
#97527=CARTESIAN_POINT('Ctrl Pts',(15.6639728424716,601.269466973693,65.6327189571251));
#97528=CARTESIAN_POINT('Ctrl Pts',(15.4132989948751,601.267834762569,65.6108481462777));
#97529=CARTESIAN_POINT('Ctrl Pts',(15.6838311981551,601.002003491397,65.37513074784));
#97530=CARTESIAN_POINT('Ctrl Pts',(15.6846836179855,601.252741847092,65.361885527254));
#97531=CARTESIAN_POINT('Ctrl Pts',(15.4341736765461,601.251664750571,65.3445748221907));
#97532=CARTESIAN_POINT('Ctrl Pts',(15.7535397227803,600.948166401941,64.0126917270571));
#97533=CARTESIAN_POINT('Ctrl Pts',(15.7525074770034,601.197957730567,64.019253662881));
#97534=CARTESIAN_POINT('Ctrl Pts',(15.5027734069943,601.198512215226,64.0208357993163));
#97535=CARTESIAN_POINT('Ctrl Pts',(15.6961577000033,600.992752129991,62.9336548017417));
#97536=CARTESIAN_POINT('Ctrl Pts',(15.6953430710373,601.244369811282,62.9419553492361));
#97537=CARTESIAN_POINT('Ctrl Pts',(15.4463052101678,601.242530165078,62.972460326068));
#97538=CARTESIAN_POINT('Ctrl Pts',(15.4449172446521,601.185978519767,61.3309552205203));
#97539=CARTESIAN_POINT('Ctrl Pts',(15.4514130025606,601.440674321061,61.3655583025674));
#97540=CARTESIAN_POINT('Ctrl Pts',(15.1990606178882,601.433299969603,61.4152823525307));
#97541=CARTESIAN_POINT('Ctrl Pts',(15.3326315846512,601.272148638439,60.7979635436387));
#97542=CARTESIAN_POINT('Ctrl Pts',(15.3413681900166,601.529059099786,60.8377615984788));
#97543=CARTESIAN_POINT('Ctrl Pts',(15.0885616588025,601.5183739204,60.897431997035));
#97544=CARTESIAN_POINT('Ctrl Pts',(15.0597162431557,601.480260879463,59.7656992724498));
#97545=CARTESIAN_POINT('Ctrl Pts',(15.0752901365765,601.741577703714,59.8177577361634));
#97546=CARTESIAN_POINT('Ctrl Pts',(14.8199878745666,601.723839648942,59.894490282593));
#97547=CARTESIAN_POINT('Ctrl Pts',(14.8986984980326,601.602505699219,59.2627428795189));
#97548=CARTESIAN_POINT('Ctrl Pts',(14.9175497152663,601.867063568807,59.3196546068316));
#97549=CARTESIAN_POINT('Ctrl Pts',(14.6615322304544,601.844529468462,59.405821548259));
#97550=CARTESIAN_POINT('Ctrl Pts',(14.5300665302068,601.879941981165,58.2814141988727));
#97551=CARTESIAN_POINT('Ctrl Pts',(14.5581603558448,602.150797938548,58.3493442354962));
#97552=CARTESIAN_POINT('Ctrl Pts',(14.2987645730368,602.118437712548,58.452368034267));
#97553=CARTESIAN_POINT('Ctrl Pts',(14.3223620118629,602.035207147482,57.8028805682137));
#97554=CARTESIAN_POINT('Ctrl Pts',(14.3547106916411,602.310430445876,57.8751573631045));
#97555=CARTESIAN_POINT('Ctrl Pts',(14.0943650477467,602.271727921001,57.987427888935));
#97556=CARTESIAN_POINT('Ctrl Pts',(13.8614639308801,602.375760037317,56.870100046218));
#97557=CARTESIAN_POINT('Ctrl Pts',(13.905352230957,602.6594624201,56.9519457897139));
#97558=CARTESIAN_POINT('Ctrl Pts',(13.6407992303396,602.607950213347,57.0811428907972));
#97559=CARTESIAN_POINT('Ctrl Pts',(13.611788274916,602.558441818736,56.4228707819826));
#97560=CARTESIAN_POINT('Ctrl Pts',(13.660997958786,602.847564244315,56.5087094937084));
#97561=CARTESIAN_POINT('Ctrl Pts',(13.3950963108816,602.788308498489,56.6466171892939));
#97562=CARTESIAN_POINT('Ctrl Pts',(13.0764921418282,602.944386245562,55.5629408541681));
#97563=CARTESIAN_POINT('Ctrl Pts',(13.1390236076535,603.244280565436,55.6564090278324));
#97564=CARTESIAN_POINT('Ctrl Pts',(12.8683162606274,603.169345173769,55.8111128357767));
#97565=CARTESIAN_POINT('Ctrl Pts',(12.7908624053289,603.147665803391,55.1502548367754));
#97566=CARTESIAN_POINT('Ctrl Pts',(12.8594650095397,603.454227818642,55.2468622237164));
#97567=CARTESIAN_POINT('Ctrl Pts',(12.5872314290769,603.370039355094,55.4101487566788));
#97568=CARTESIAN_POINT('Ctrl Pts',(12.1845042755668,603.571151168872,54.3570282351227));
#97569=CARTESIAN_POINT('Ctrl Pts',(12.2679641743712,603.891253550521,54.4591095196187));
#97570=CARTESIAN_POINT('Ctrl Pts',(11.9905202907966,603.788139618472,54.6394524585066));
#97571=CARTESIAN_POINT('Ctrl Pts',(11.8627313233714,603.792069253919,53.9753888666545));
#97572=CARTESIAN_POINT('Ctrl Pts',(11.9529310376215,604.120352293626,54.0796602679055));
#97573=CARTESIAN_POINT('Ctrl Pts',(11.6738674877948,604.006248090623,54.2686527469967));
#97574=CARTESIAN_POINT('Ctrl Pts',(10.8510402072694,604.469985948396,52.8843970456025));
#97575=CARTESIAN_POINT('Ctrl Pts',(10.945265328937,604.837892193095,52.9711566209328));
#97576=CARTESIAN_POINT('Ctrl Pts',(10.6782856421904,604.675535692234,53.2086614405224));
#97577=CARTESIAN_POINT('Ctrl Pts',(10.1231644802855,604.937352782708,52.2355170621796));
#97578=CARTESIAN_POINT('Ctrl Pts',(10.2261851601175,605.328623293813,52.325672618392));
#97579=CARTESIAN_POINT('Ctrl Pts',(9.9619956407393,605.13695811471,52.5782081758289));
#97580=CARTESIAN_POINT('Ctrl Pts',(8.94566114499843,605.634568642711,51.3658592810726));
#97581=CARTESIAN_POINT('Ctrl Pts',(9.09775647626564,606.047668837203,51.4706442472986));
#97582=CARTESIAN_POINT('Ctrl Pts',(8.80321427157987,605.825316635566,51.7332383677212));
#97583=CARTESIAN_POINT('Ctrl Pts',(8.53871075522488,605.866292458671,51.0934261046552));
#97584=CARTESIAN_POINT('Ctrl Pts',(8.69719315797,606.293588447686,51.1963055952873));
#97585=CARTESIAN_POINT('Ctrl Pts',(8.40274055580763,606.054093444861,51.468542205798));
#97586=CARTESIAN_POINT('Ctrl Pts',(7.69242405624649,606.322458739373,50.5832101346318));
#97587=CARTESIAN_POINT('Ctrl Pts',(7.86343028959298,606.781403923533,50.6785875112157));
#97588=CARTESIAN_POINT('Ctrl Pts',(7.56992268932879,606.504457879526,50.9728170395581));
#97589=CARTESIAN_POINT('Ctrl Pts',(7.25341144010781,606.546582345598,50.3459105384044));
#97590=CARTESIAN_POINT('Ctrl Pts',(7.42930129741494,607.022466301498,50.4376325390388));
#97591=CARTESIAN_POINT('Ctrl Pts',(7.13789769244056,606.725731037077,50.7422564476865));
#97592=CARTESIAN_POINT('Ctrl Pts',(5.74078325584115,607.262802253728,49.6195861520783));
#97593=CARTESIAN_POINT('Ctrl Pts',(5.86838675370132,607.833044383481,49.6620231583292));
#97594=CARTESIAN_POINT('Ctrl Pts',(5.64937448274724,607.432827203209,50.036573743915));
#97595=CARTESIAN_POINT('Ctrl Pts',(4.61020627219875,607.711095870914,49.2207424753209));
#97596=CARTESIAN_POINT('Ctrl Pts',(4.73821803523183,608.319969502878,49.262455296545));
#97597=CARTESIAN_POINT('Ctrl Pts',(4.53678997843925,607.875425333392,49.6490480272317));
#97598=CARTESIAN_POINT('Ctrl Pts',(3.37684626304299,608.03198826415,48.9478721491));
#97599=CARTESIAN_POINT('Ctrl Pts',(3.53826781775195,608.671892366682,48.9831770877157));
#97600=CARTESIAN_POINT('Ctrl Pts',(3.32305067588146,608.192239283157,49.3839240770586));
#97601=CARTESIAN_POINT('',(3.445572367957E-11,608.476132031989,80.0177796115133));
#97602=CARTESIAN_POINT('',(3.93978362444746,607.874843764614,49.082928510463));
#97603=CARTESIAN_POINT('Ctrl Pts',(6.891144735914E-11,608.476132031982,
80.0177787907144));
#97604=CARTESIAN_POINT('Ctrl Pts',(0.023608644378443,608.476133391052,80.0177797817517));
#97605=CARTESIAN_POINT('Ctrl Pts',(0.0471977207100223,608.476067912617,
80.0177272377913));
#97606=CARTESIAN_POINT('Ctrl Pts',(0.0707638231545097,608.475935523855,
80.017621142111));
#97607=CARTESIAN_POINT('Ctrl Pts',(0.343491007326588,608.474403407364,80.0163933117468));
#97608=CARTESIAN_POINT('Ctrl Pts',(0.614496441609094,608.464020952774,80.0080814531982));
#97609=CARTESIAN_POINT('Ctrl Pts',(0.883878526644414,608.445171171727,79.992909437795));
#97610=CARTESIAN_POINT('Ctrl Pts',(1.24943310899289,608.419591802421,79.9723208386927));
#97611=CARTESIAN_POINT('Ctrl Pts',(1.61199825335794,608.378394662748,79.9391295369998));
#97612=CARTESIAN_POINT('Ctrl Pts',(1.97182100459186,608.322782114007,79.8936222931225));
#97613=CARTESIAN_POINT('Ctrl Pts',(2.14338863407167,608.296265410646,79.8719239154367));
#97614=CARTESIAN_POINT('Ctrl Pts',(2.31433265226537,608.266470720811,79.8474250872981));
#97615=CARTESIAN_POINT('Ctrl Pts',(2.48467918176857,608.233525031413,79.8201546029834));
#97616=CARTESIAN_POINT('Ctrl Pts',(2.64668359998501,608.202192739179,79.7942195929848));
#97617=CARTESIAN_POINT('Ctrl Pts',(2.80854164377701,608.167910736366,79.7656811760263));
#97618=CARTESIAN_POINT('Ctrl Pts',(2.96931905952992,608.131056409394,79.7347565578901));
#97619=CARTESIAN_POINT('Ctrl Pts',(3.07072240523472,608.107812149364,79.7152522031959));
#97620=CARTESIAN_POINT('Ctrl Pts',(3.17169670908154,608.083545727609,79.6947984620929));
#97621=CARTESIAN_POINT('Ctrl Pts',(3.2720087069542,608.05835117884,79.6734492843488));
#97622=CARTESIAN_POINT('Ctrl Pts',(3.53149735464349,607.993177525359,79.6182228968817));
#97623=CARTESIAN_POINT('Ctrl Pts',(3.78656458821257,607.921882403724,79.5570823750604));
#97624=CARTESIAN_POINT('Ctrl Pts',(4.03770549440548,607.845341550768,79.4903295169232));
#97625=CARTESIAN_POINT('Ctrl Pts',(4.40729347692822,607.732701280996,79.3920936120658));
#97626=CARTESIAN_POINT('Ctrl Pts',(4.76841289982341,607.608751209855,79.2817479196197));
#97627=CARTESIAN_POINT('Ctrl Pts',(5.12226678865739,607.475746685772,79.1597571080133));
#97628=CARTESIAN_POINT('Ctrl Pts',(5.24929534886865,607.427999935689,79.1159641255244));
#97629=CARTESIAN_POINT('Ctrl Pts',(5.37538735229175,607.379086051863,79.0706700669591));
#97630=CARTESIAN_POINT('Ctrl Pts',(5.50059773443485,607.32910861461,79.0238952610022));
#97631=CARTESIAN_POINT('Ctrl Pts',(5.57281046246083,607.300285069613,78.9969187732444));
#97632=CARTESIAN_POINT('Ctrl Pts',(5.64472953797074,607.271107125461,78.9694492784864));
#97633=CARTESIAN_POINT('Ctrl Pts',(5.71636225209787,607.241589948643,78.9414864057523));
#97634=CARTESIAN_POINT('Ctrl Pts',(6.1145430789441,607.077514441875,78.7860507235792));
#97635=CARTESIAN_POINT('Ctrl Pts',(6.50370968196559,606.903036652875,78.6154339417837));
#97636=CARTESIAN_POINT('Ctrl Pts',(6.8848883010362,606.720902758003,78.4297064786912));
#97637=CARTESIAN_POINT('Ctrl Pts',(7.33445681558759,606.506090959885,78.210656365394));
#97638=CARTESIAN_POINT('Ctrl Pts',(7.76935072835595,606.282265744325,77.9721566871374));
#97639=CARTESIAN_POINT('Ctrl Pts',(8.187458217611,606.055505133889,77.7170253648745));
#97640=CARTESIAN_POINT('Ctrl Pts',(8.18746947767835,606.055499026991,77.717018493924));
#97641=CARTESIAN_POINT('Ctrl Pts',(8.18748073773472,606.05549292009,77.7170116229611));
#97642=CARTESIAN_POINT('Ctrl Pts',(8.18749199778011,606.055486813187,77.7170047519856));
#97643=CARTESIAN_POINT('Ctrl Pts',(8.77466513832359,605.737032553591,77.3587067095187));
#97644=CARTESIAN_POINT('Ctrl Pts',(9.33198432025338,605.411622763145,76.9665375838635));
#97645=CARTESIAN_POINT('Ctrl Pts',(9.86244451672601,605.086463613717,76.5388820034507));
#97646=CARTESIAN_POINT('Ctrl Pts',(10.0299804484333,604.983768177915,76.4038149869418));
#97647=CARTESIAN_POINT('Ctrl Pts',(10.1948374650659,604.881097800488,76.2652085139033));
#97648=CARTESIAN_POINT('Ctrl Pts',(10.3571105681779,604.778679548307,76.1230125476067));
#97649=CARTESIAN_POINT('Ctrl Pts',(10.4125855674164,604.743666645041,76.0744011574826));
#97650=CARTESIAN_POINT('Ctrl Pts',(10.4677585361306,604.708682049518,76.0253703145274));
#97651=CARTESIAN_POINT('Ctrl Pts',(10.5226333425913,604.673735097822,75.9759179749725));
#97652=CARTESIAN_POINT('Ctrl Pts',(10.8021362240136,604.495734038209,75.7240342365111));
#97653=CARTESIAN_POINT('Ctrl Pts',(11.0737787493323,604.318624837962,75.4611186031081));
#97654=CARTESIAN_POINT('Ctrl Pts',(11.3375596732538,604.143426989905,75.1864000604821));
#97655=CARTESIAN_POINT('Ctrl Pts',(11.4152479295857,604.091828052703,75.105490477479));
#97656=CARTESIAN_POINT('Ctrl Pts',(11.4922757377262,604.040378802491,75.023534546417));
#97657=CARTESIAN_POINT('Ctrl Pts',(11.5686281331514,603.989114002876,74.9405265476199));
#97658=CARTESIAN_POINT('Ctrl Pts',(11.7428614430267,603.872129648067,74.7511053998486));
#97659=CARTESIAN_POINT('Ctrl Pts',(11.9125329809615,603.756803523413,74.5572877444752));
#97660=CARTESIAN_POINT('Ctrl Pts',(12.0772418647187,603.643694083311,74.3595533209466));
#97661=CARTESIAN_POINT('Ctrl Pts',(12.1335432671765,603.60503059435,74.2919630058106));
#97662=CARTESIAN_POINT('Ctrl Pts',(12.1892651384275,603.566625966915,74.2239153125446));
#97663=CARTESIAN_POINT('Ctrl Pts',(12.2443925060635,603.528501994852,74.1554302041702));
#97664=CARTESIAN_POINT('Ctrl Pts',(12.3387364620062,603.463257335169,74.0382260581302));
#97665=CARTESIAN_POINT('Ctrl Pts',(12.4314151262027,603.398784198907,73.9196466444437));
#97666=CARTESIAN_POINT('Ctrl Pts',(12.5223735539976,603.335175124649,73.7997538153799));
#97667=CARTESIAN_POINT('Ctrl Pts',(12.7691297819514,603.162613487337,73.474503006019));
#97668=CARTESIAN_POINT('Ctrl Pts',(13.003843124458,602.996038420695,73.1391451429734));
#97669=CARTESIAN_POINT('Ctrl Pts',(13.2260892248692,602.836485522975,72.7931543849762));
#97670=CARTESIAN_POINT('Ctrl Pts',(13.4204829916168,602.696928119152,72.4905238930013));
#97671=CARTESIAN_POINT('Ctrl Pts',(13.6053390538352,602.562743113451,72.1797589167256));
#97672=CARTESIAN_POINT('Ctrl Pts',(13.7803977512332,602.434610850826,71.8605255759729));
#97673=CARTESIAN_POINT('Ctrl Pts',(13.8914471872944,602.353329453687,71.6580181713741));
#97674=CARTESIAN_POINT('Ctrl Pts',(13.9985704807448,602.274488846586,71.4520750410271));
#97675=CARTESIAN_POINT('Ctrl Pts',(14.1017118649645,602.198253227673,71.2425913130359));
#97676=CARTESIAN_POINT('Ctrl Pts',(14.2070716057042,602.120377939255,71.0286020260264));
#97677=CARTESIAN_POINT('Ctrl Pts',(14.3082384476158,602.04522874082,70.81089177479));
#97678=CARTESIAN_POINT('Ctrl Pts',(14.4050208561385,601.97303833151,70.5892424956487));
#97679=CARTESIAN_POINT('Ctrl Pts',(14.5157812425591,601.890421689158,70.3355811104625));
#97680=CARTESIAN_POINT('Ctrl Pts',(14.6208678960898,601.811623873729,70.0765942455147));
#97681=CARTESIAN_POINT('Ctrl Pts',(14.7199048617496,601.737072380968,69.8121463246681));
#97682=CARTESIAN_POINT('Ctrl Pts',(14.7921227929364,601.682709300089,69.6193104312928));
#97683=CARTESIAN_POINT('Ctrl Pts',(14.8606224440704,601.630982676328,69.4248390807865));
#97684=CARTESIAN_POINT('Ctrl Pts',(14.9252970870176,601.582022741331,69.2290149637919));
#97685=CARTESIAN_POINT('Ctrl Pts',(15.0269343231625,601.505081420156,68.9212742308732));
#97686=CARTESIAN_POINT('Ctrl Pts',(15.1192104490316,601.434902446505,68.6099443406549));
#97687=CARTESIAN_POINT('Ctrl Pts',(15.2018005707495,601.371913878203,68.2957740937441));
#97688=CARTESIAN_POINT('Ctrl Pts',(15.3370175067359,601.268788697724,67.781413086861));
#97689=CARTESIAN_POINT('Ctrl Pts',(15.4467112583919,601.184600964787,67.2582968021332));
#97690=CARTESIAN_POINT('Ctrl Pts',(15.5298941967001,601.120624070575,66.7258995592193));
#97691=CARTESIAN_POINT('Ctrl Pts',(15.5492380442097,601.105746509011,66.6020927871707));
#97692=CARTESIAN_POINT('Ctrl Pts',(15.567145084157,601.091963469233,66.4777831582835));
#97693=CARTESIAN_POINT('Ctrl Pts',(15.5835932838998,601.079296047254,66.3529610769457));
#97694=CARTESIAN_POINT('Ctrl Pts',(15.6025152015847,601.064723515323,66.2093664474261));
#97695=CARTESIAN_POINT('Ctrl Pts',(15.6195051466467,601.051628333843,66.0651039293665));
#97696=CARTESIAN_POINT('Ctrl Pts',(15.6345304353988,601.040042512501,65.9201567812727));
#97697=CARTESIAN_POINT('Ctrl Pts',(15.6626204963928,601.018382600765,65.6491753513615));
#97698=CARTESIAN_POINT('Ctrl Pts',(15.6838314901426,601.002007634833,65.3751252063361));
#97699=CARTESIAN_POINT('Ctrl Pts',(15.6977729274255,600.991248095703,65.1026424621912));
#97700=CARTESIAN_POINT('Ctrl Pts',(15.7020662908531,600.987934620136,65.0187294893299));
#97701=CARTESIAN_POINT('Ctrl Pts',(15.7056890266772,600.985141168189,64.934880886641));
#97702=CARTESIAN_POINT('Ctrl Pts',(15.7086425189985,600.982866284406,64.8510957582209));
#97703=CARTESIAN_POINT('Ctrl Pts',(15.7263165930932,600.969253090209,64.3497148820873));
#97704=CARTESIAN_POINT('Ctrl Pts',(15.7200248924218,600.974244879535,63.8506118554521));
#97705=CARTESIAN_POINT('Ctrl Pts',(15.690054723568,600.997369844198,63.3537494689464));
#97706=CARTESIAN_POINT('Ctrl Pts',(15.6600845547142,601.020494808862,62.8568870824407));
#97707=CARTESIAN_POINT('Ctrl Pts',(15.6064372952925,601.061755283394,62.3622858632638));
#97708=CARTESIAN_POINT('Ctrl Pts',(15.5294020172295,601.121002544319,61.8699005539026));
#97709=CARTESIAN_POINT('Ctrl Pts',(15.5291562735781,601.121191543938,61.8683298376431));
#97710=CARTESIAN_POINT('Ctrl Pts',(15.5289102911643,601.121380726214,61.8667591390815));
#97711=CARTESIAN_POINT('Ctrl Pts',(15.5286640699994,601.121570091134,61.8651884582589));
#97712=CARTESIAN_POINT('Ctrl Pts',(15.4868770628324,601.153707837259,61.5986230278064));
#97713=CARTESIAN_POINT('Ctrl Pts',(15.4379580369834,601.19128412897,61.3322197252209));
#97714=CARTESIAN_POINT('Ctrl Pts',(15.3824805581734,601.233797688178,61.0681260116062));
#97715=CARTESIAN_POINT('Ctrl Pts',(15.3358122267525,601.269560612406,60.8459671605279));
#97716=CARTESIAN_POINT('Ctrl Pts',(15.2845038713035,601.308816554583,60.625443469707));
#97717=CARTESIAN_POINT('Ctrl Pts',(15.2289186178845,601.351251028551,60.4078240107633));
#97718=CARTESIAN_POINT('Ctrl Pts',(15.2181659569586,601.35945974367,60.3657267258007));
#97719=CARTESIAN_POINT('Ctrl Pts',(15.2072508201014,601.367788808569,60.3237283373609));
#97720=CARTESIAN_POINT('Ctrl Pts',(15.196175503333,601.376236194403,60.2818374278755));
#97721=CARTESIAN_POINT('Ctrl Pts',(15.096781692569,601.452046023291,59.9058935865223));
#97722=CARTESIAN_POINT('Ctrl Pts',(14.9842779945814,601.53754841251,59.536653111409));
#97723=CARTESIAN_POINT('Ctrl Pts',(14.859145984944,601.63209461805,59.1739255762946));
#97724=CARTESIAN_POINT('Ctrl Pts',(14.8126284390042,601.667241959425,59.0390824228346));
#97725=CARTESIAN_POINT('Ctrl Pts',(14.7643660978949,601.703638825262,58.9051391515248));
#97726=CARTESIAN_POINT('Ctrl Pts',(14.7143850694044,601.741250875155,58.7720853460319));
#97727=CARTESIAN_POINT('Ctrl Pts',(14.5736911865015,601.84712675453,58.3975461039397));
#97728=CARTESIAN_POINT('Ctrl Pts',(14.4193228109465,601.962676680985,58.0299622878074));
#97729=CARTESIAN_POINT('Ctrl Pts',(14.2516172400983,602.087194168844,57.6694867820627));
#97730=CARTESIAN_POINT('Ctrl Pts',(14.1996634649568,602.125768639165,57.5578145026341));
#97731=CARTESIAN_POINT('Ctrl Pts',(14.1464260882526,602.165206051972,57.4468157386464));
#97732=CARTESIAN_POINT('Ctrl Pts',(14.0919132979964,602.205485809269,57.3364909682744));
#97733=CARTESIAN_POINT('Ctrl Pts',(13.9337411446871,602.322359957823,57.0163769838124));
#97734=CARTESIAN_POINT('Ctrl Pts',(13.7664884987757,602.445098355549,56.7052436349986));
#97735=CARTESIAN_POINT('Ctrl Pts',(13.5905541920496,602.573008005882,56.4024860662583));
#97736=CARTESIAN_POINT('Ctrl Pts',(13.5102146755005,602.631417304562,56.2642333447919));
#97737=CARTESIAN_POINT('Ctrl Pts',(13.4280641419558,602.690908584722,56.1277259803299));
#97738=CARTESIAN_POINT('Ctrl Pts',(13.3441406912912,602.751416392403,55.9929065938881));
#97739=CARTESIAN_POINT('Ctrl Pts',(13.18094216384,602.869080585599,55.7307352321897));
#97740=CARTESIAN_POINT('Ctrl Pts',(13.0110358717025,602.990595148795,55.474952500565));
#97741=CARTESIAN_POINT('Ctrl Pts',(12.834515971694,603.115539209283,55.2252918717908));
#97742=CARTESIAN_POINT('Ctrl Pts',(12.7215730554199,603.195482301036,55.065551244863));
#97743=CARTESIAN_POINT('Ctrl Pts',(12.6059608809529,603.276803544364,54.9083700535969));
#97744=CARTESIAN_POINT('Ctrl Pts',(12.4876834913282,603.359409062561,54.7536417333293));
#97745=CARTESIAN_POINT('Ctrl Pts',(12.3260424195162,603.472299992445,54.5421858362463));
#97746=CARTESIAN_POINT('Ctrl Pts',(12.1591272633341,603.587791808995,54.3349982249624));
#97747=CARTESIAN_POINT('Ctrl Pts',(11.9873446890175,603.705306278801,54.132457025428));
#97748=CARTESIAN_POINT('Ctrl Pts',(11.8370887041423,603.808094658053,53.9552968708842));
#97749=CARTESIAN_POINT('Ctrl Pts',(11.682992340067,603.912509879882,53.7815611779533));
#97750=CARTESIAN_POINT('Ctrl Pts',(11.5255012613246,604.018042470088,53.6117252605926));
#97751=CARTESIAN_POINT('Ctrl Pts',(11.3711873179765,604.121446105878,53.445315516375));
#97752=CARTESIAN_POINT('Ctrl Pts',(11.2140552717419,604.225670952781,53.2829927429756));
#97753=CARTESIAN_POINT('Ctrl Pts',(11.0542019754069,604.330409538232,53.1247785161059));
#97754=CARTESIAN_POINT('Ctrl Pts',(10.5698058925877,604.647794050629,52.6453492300101));
#97755=CARTESIAN_POINT('Ctrl Pts',(10.0592926797871,604.97065899169,52.2024986105179));
#97756=CARTESIAN_POINT('Ctrl Pts',(9.5214912839734,605.292961601669,51.7931946721202));
#97757=CARTESIAN_POINT('Ctrl Pts',(9.46073141911627,605.329374789098,51.7469522261613));
#97758=CARTESIAN_POINT('Ctrl Pts',(9.39962327601398,605.365780791358,51.7011379286063));
#97759=CARTESIAN_POINT('Ctrl Pts',(9.3381651900171,605.40217089056,51.6557473746705));
#97760=CARTESIAN_POINT('Ctrl Pts',(9.21814549218713,605.473236050488,51.5671054900537));
#97761=CARTESIAN_POINT('Ctrl Pts',(9.09677553395676,605.544236595435,51.4800960735065));
#97762=CARTESIAN_POINT('Ctrl Pts',(8.97400639050295,605.615087250737,51.3947159850713));
#97763=CARTESIAN_POINT('Ctrl Pts',(8.69526626352681,605.775949500807,51.200865510741));
#97764=CARTESIAN_POINT('Ctrl Pts',(8.40931705214077,605.936070716091,51.0154168364813));
#97765=CARTESIAN_POINT('Ctrl Pts',(8.11558835298554,606.094427751649,50.8383307562355));
#97766=CARTESIAN_POINT('Ctrl Pts',(7.69239174854488,606.322584414344,50.5831897772666));
#97767=CARTESIAN_POINT('Ctrl Pts',(7.25336993337879,606.546758860276,50.3458922881572));
#97768=CARTESIAN_POINT('Ctrl Pts',(6.8038425239994,606.759577373996,50.1300393648259));
#97769=CARTESIAN_POINT('Ctrl Pts',(6.73473828265154,606.792293203172,50.0968570667095));
#97770=CARTESIAN_POINT('Ctrl Pts',(6.66535065282465,606.82477352714,50.0641473617017));
#97771=CARTESIAN_POINT('Ctrl Pts',(6.59567017408018,606.856998130578,50.0319141884441));
#97772=CARTESIAN_POINT('Ctrl Pts',(6.03292698896474,607.117245710745,49.7715973979719));
#97773=CARTESIAN_POINT('Ctrl Pts',(5.45113667966419,607.360978280686,49.542387508329));
#97774=CARTESIAN_POINT('Ctrl Pts',(4.8452572739386,607.577752733781,49.3462933887054));
#97775=CARTESIAN_POINT('Ctrl Pts',(4.54937241788851,607.683615843243,49.2505296446191));
#97776=CARTESIAN_POINT('Ctrl Pts',(4.24774282917826,607.783050325799,49.1626636005067));
#97777=CARTESIAN_POINT('Ctrl Pts',(3.93978362444746,607.874843764614,49.082928510463));
#97778=CARTESIAN_POINT('',(3.87712128125394,608.037287038731,49.5149800517143));
#97779=CARTESIAN_POINT('Origin',(3.87712128127698,607.874843764616,49.3249479946959));
#97780=CARTESIAN_POINT('',(-3.85030552837329,608.045280920111,79.0907977188138));
#97781=CARTESIAN_POINT('Ctrl Pts',(3.87712128125394,608.037287038731,49.5149800517143));
#97782=CARTESIAN_POINT('Ctrl Pts',(4.87153021748849,607.739915203809,49.7691795549397));
#97783=CARTESIAN_POINT('Ctrl Pts',(5.79934294385505,607.361106997409,50.1085862160764));
#97784=CARTESIAN_POINT('Ctrl Pts',(7.12166692125997,606.734009856725,50.7337821806858));
#97785=CARTESIAN_POINT('Ctrl Pts',(7.55227759129253,606.513849499917,50.9628773512951));
#97786=CARTESIAN_POINT('Ctrl Pts',(8.38321347944639,606.065233520004,51.4559004400492));
#97787=CARTESIAN_POINT('Ctrl Pts',(8.78304187688083,605.837184142117,51.7192666405192));
#97788=CARTESIAN_POINT('Ctrl Pts',(9.94055760102618,605.150556485895,52.5603722809289));
#97789=CARTESIAN_POINT('Ctrl Pts',(10.6569237854819,604.689665531714,53.1884290403189));
#97790=CARTESIAN_POINT('Ctrl Pts',(11.6536196238761,604.020275142643,54.2454145926918));
#97791=CARTESIAN_POINT('Ctrl Pts',(11.9710603883753,603.801813085304,54.6156007098022));
#97792=CARTESIAN_POINT('Ctrl Pts',(12.5694073935915,603.382876923177,55.385215476498));
#97793=CARTESIAN_POINT('Ctrl Pts',(12.8514309701718,603.181641349324,55.7857953218243));
#97794=CARTESIAN_POINT('Ctrl Pts',(13.3802712808598,602.79932278676,56.6209194460713));
#97795=CARTESIAN_POINT('Ctrl Pts',(13.6270976333542,602.618222784044,57.0554488359468));
#97796=CARTESIAN_POINT('Ctrl Pts',(14.0830317948412,602.280372513136,57.9622402793));
#97797=CARTESIAN_POINT('Ctrl Pts',(14.288866825385,602.126052058398,58.4281588815737));
#97798=CARTESIAN_POINT('Ctrl Pts',(14.6541428180436,601.850313463799,59.3835018865815));
#97799=CARTESIAN_POINT('Ctrl Pts',(14.813802564089,601.728726306764,59.8733378707772));
#97800=CARTESIAN_POINT('Ctrl Pts',(15.0845904681104,601.521591068862,60.8791319779345));
#97801=CARTESIAN_POINT('Ctrl Pts',(15.1961319187924,601.435719945448,61.3988026843396));
#97802=CARTESIAN_POINT('Ctrl Pts',(15.445895886564,601.243012879202,62.9621091081608));
#97803=CARTESIAN_POINT('Ctrl Pts',(15.5031899681929,601.198348388516,64.0148308425101));
#97804=CARTESIAN_POINT('Ctrl Pts',(15.4344186449233,601.251635259198,65.3443173476824));
#97805=CARTESIAN_POINT('Ctrl Pts',(15.4134449473779,601.267882404695,65.6117770146501));
#97806=CARTESIAN_POINT('Ctrl Pts',(15.3578567110548,601.310887267439,66.1405396918101));
#97807=CARTESIAN_POINT('Ctrl Pts',(15.3232550273986,601.337635013737,66.4025181324823));
#97808=CARTESIAN_POINT('Ctrl Pts',(15.1997028143738,601.432969072053,67.1815043824831));
#97809=CARTESIAN_POINT('Ctrl Pts',(15.0910612840211,601.516618757114,67.6915802539796));
#97810=CARTESIAN_POINT('Ctrl Pts',(14.8233372862475,601.721454107234,68.694153518926));
#97811=CARTESIAN_POINT('Ctrl Pts',(14.6637788819681,601.843004162358,69.1878707203431));
#97812=CARTESIAN_POINT('Ctrl Pts',(14.2965526740649,602.120283814448,70.1529519783302));
#97813=CARTESIAN_POINT('Ctrl Pts',(14.0918748017888,602.273750570818,70.6169548967642));
#97814=CARTESIAN_POINT('Ctrl Pts',(13.4200658305586,602.771767364609,71.9594073502309));
#97815=CARTESIAN_POINT('Ctrl Pts',(12.8958575906797,603.153805305363,72.7887618167445));
#97816=CARTESIAN_POINT('Ctrl Pts',(12.0012587128913,603.78090420349,73.9468631187593));
#97817=CARTESIAN_POINT('Ctrl Pts',(11.683780665072,603.999674377738,74.3193541873481));
#97818=CARTESIAN_POINT('Ctrl Pts',(11.0214171690138,604.445181629234,75.0259744723523));
#97819=CARTESIAN_POINT('Ctrl Pts',(10.6774393735486,604.671360763517,75.3595543546866));
#97820=CARTESIAN_POINT('Ctrl Pts',(9.60714722132492,605.353866408868,76.3061032107106));
#97821=CARTESIAN_POINT('Ctrl Pts',(8.84327964705721,605.814723142904,76.865511939863));
#97822=CARTESIAN_POINT('Ctrl Pts',(7.60921202386664,606.484073904586,77.6043583167633));
#97823=CARTESIAN_POINT('Ctrl Pts',(7.1813427653491,606.704199580113,77.8345316034363));
#97824=CARTESIAN_POINT('Ctrl Pts',(6.29818432438025,607.125857945281,78.2566267740411));
#97825=CARTESIAN_POINT('Ctrl Pts',(5.84582286264931,607.326074990086,78.4473366643001));
#97826=CARTESIAN_POINT('Ctrl Pts',(4.91622538701958,607.696478903184,78.7878860584469));
#97827=CARTESIAN_POINT('Ctrl Pts',(4.43900471573538,607.86669051722,78.9377439866561));
#97828=CARTESIAN_POINT('Ctrl Pts',(3.45473183503186,608.165828521108,79.1941909352119));
#97829=CARTESIAN_POINT('Ctrl Pts',(2.94362350959894,608.295390945239,79.3013079500641));
#97830=CARTESIAN_POINT('Ctrl Pts',(1.90950562370682,608.494575880372,79.4634826852088));
#97831=CARTESIAN_POINT('Ctrl Pts',(1.38650131959488,608.564625822707,79.5190163918644));
#97832=CARTESIAN_POINT('Ctrl Pts',(0.592249243454403,608.619578731141,79.5625292223074));
#97833=CARTESIAN_POINT('Ctrl Pts',(0.325874264894089,608.629555363385,79.5703863596371));
#97834=CARTESIAN_POINT('Ctrl Pts',(-0.21025693007535,608.632063664679,79.5723645937365));
#97835=CARTESIAN_POINT('Ctrl Pts',(-0.48111240188688,608.624461420681,79.5663806670725));
#97836=CARTESIAN_POINT('Ctrl Pts',(-1.81787718546613,608.543639087743,79.5024445409065));
#97837=CARTESIAN_POINT('Ctrl Pts',(-2.84910806661434,608.342800223654,79.3448450590357));
#97838=CARTESIAN_POINT('Ctrl Pts',(-3.85030552837329,608.045280920111,79.0907977188138));
#97839=CARTESIAN_POINT('',(-3.91253447320281,607.88294039512,79.5230488432747));
#97840=CARTESIAN_POINT('Origin',(-3.85030552837329,607.88294039512,79.2809175598242));
#97841=CARTESIAN_POINT('Ctrl Pts',(-3.91253447320281,607.88294039512,79.5230488432747));
#97842=CARTESIAN_POINT('Ctrl Pts',(-3.28597810505974,608.068523823524,79.6840769479877));
#97843=CARTESIAN_POINT('Ctrl Pts',(-2.64771851246926,608.217057906509,79.807103090937));
#97844=CARTESIAN_POINT('Ctrl Pts',(-1.67000646568519,608.37000307792,79.9322661229594));
#97845=CARTESIAN_POINT('Ctrl Pts',(-1.34070899812117,608.409338421479,79.9640509087433));
#97846=CARTESIAN_POINT('Ctrl Pts',(-0.674809016948164,608.462436221459,
80.0068322484697));
#97847=CARTESIAN_POINT('Ctrl Pts',(-0.336249102370441,608.476132031997,
80.0177804323122));
#97848=CARTESIAN_POINT('Ctrl Pts',(0.,608.476132031997,80.0177804323122));
#97849=CARTESIAN_POINT('Ctrl Pts',(1.89318255568148,606.702491294468,79.9033522554387));
#97850=CARTESIAN_POINT('Ctrl Pts',(1.88043236474459,606.605433408562,79.9049255377571));
#97851=CARTESIAN_POINT('Ctrl Pts',(1.86306288877797,606.534169754924,79.840079036097));
#97852=CARTESIAN_POINT('Ctrl Pts',(0.820646498012525,606.843220307922,80.0334805824724));
#97853=CARTESIAN_POINT('Ctrl Pts',(0.818743950698483,606.747324662366,80.0328500715449));
#97854=CARTESIAN_POINT('Ctrl Pts',(0.807589904959771,606.67659431856,79.9696785476399));
#97855=CARTESIAN_POINT('Ctrl Pts',(-0.249753392942154,606.864684633585,
80.0523236519829));
#97856=CARTESIAN_POINT('Ctrl Pts',(-0.250591804105095,606.769288903197,
80.0516667261813));
#97857=CARTESIAN_POINT('Ctrl Pts',(-0.24578162409436,606.698317026832,79.9884448322078));
#97858=CARTESIAN_POINT('Ctrl Pts',(-1.85230285694165,606.71760788908,79.9174605062688));
#97859=CARTESIAN_POINT('Ctrl Pts',(-1.84045202787124,606.620669616219,79.9187905906115));
#97860=CARTESIAN_POINT('Ctrl Pts',(-1.82283398292192,606.549468432993,79.8541299127167));
#97861=CARTESIAN_POINT('Ctrl Pts',(-2.38933484362825,606.638031596339,79.8441641306276));
#97862=CARTESIAN_POINT('Ctrl Pts',(-2.37466264357767,606.539938200002,79.8462807686187));
#97863=CARTESIAN_POINT('Ctrl Pts',(-2.35132258925576,606.468933259531,79.7811312873554));
#97864=CARTESIAN_POINT('Ctrl Pts',(-3.43147735551065,606.430320367494,79.6478052879441));
#97865=CARTESIAN_POINT('Ctrl Pts',(-3.4101627228699,606.329716176394,79.6525292086393));
#97866=CARTESIAN_POINT('Ctrl Pts',(-3.37688542676327,606.258719512165,79.5855704382192));
#97867=CARTESIAN_POINT('Ctrl Pts',(-3.93983799323764,606.302315894287,79.524834163758));
#97868=CARTESIAN_POINT('Ctrl Pts',(-3.91596185111129,606.19983418155,79.5308660063145));
#97869=CARTESIAN_POINT('Ctrl Pts',(-3.87715892282217,606.12917261973,79.4630988338053));
#97870=CARTESIAN_POINT('Ctrl Pts',(-4.93450429122366,606.007958107776,79.2321422141563));
#97871=CARTESIAN_POINT('Ctrl Pts',(-4.9048700052628,605.901729272729,79.2419298822336));
#97872=CARTESIAN_POINT('Ctrl Pts',(-4.85600136127738,605.831268332999,79.1715962336162));
#97873=CARTESIAN_POINT('Ctrl Pts',(-5.42323859046886,605.840637330157,79.0613640029475));
#97874=CARTESIAN_POINT('Ctrl Pts',(-5.3913805012487,605.731886424723,79.0729171785271));
#97875=CARTESIAN_POINT('Ctrl Pts',(-5.33696096117466,605.661931391049,79.0015116750124));
#97876=CARTESIAN_POINT('Ctrl Pts',(-6.36814164931806,605.481318537322,78.6790317667906));
#97877=CARTESIAN_POINT('Ctrl Pts',(-6.33161473347315,605.367659836615,78.6952414948338));
#97878=CARTESIAN_POINT('Ctrl Pts',(-6.26683249734681,605.298283329195,78.6207327915938));
#97879=CARTESIAN_POINT('Ctrl Pts',(-6.8234072526896,605.289965981239,78.4682119648795));
#97880=CARTESIAN_POINT('Ctrl Pts',(-6.78508370064266,605.17331911893,78.4865227570079));
#97881=CARTESIAN_POINT('Ctrl Pts',(-6.71485606394656,605.104625043036,78.4107691833072));
#97882=CARTESIAN_POINT('Ctrl Pts',(-8.14524394474732,604.693296470928,77.7793700065673));
#97883=CARTESIAN_POINT('Ctrl Pts',(-8.10998737994438,604.564036856332,77.80127117446));
#97884=CARTESIAN_POINT('Ctrl Pts',(-8.01567130514643,604.500763916929,77.7247225905372));
#97885=CARTESIAN_POINT('Ctrl Pts',(-8.96853196172094,604.265846804672,77.2457034968301));
#97886=CARTESIAN_POINT('Ctrl Pts',(-8.93226681233894,604.127883129672,77.269520633413));
#97887=CARTESIAN_POINT('Ctrl Pts',(-8.82586458852353,604.068162696145,77.1932211322336));
#97888=CARTESIAN_POINT('Ctrl Pts',(-10.1303565945194,603.615007657105,76.327964798955));
#97889=CARTESIAN_POINT('Ctrl Pts',(-10.0844043143262,603.470213448972,76.3668461206142));
#97890=CARTESIAN_POINT('Ctrl Pts',(-9.96920498164766,603.409484218181,76.2792128579425));
#97891=CARTESIAN_POINT('Ctrl Pts',(-10.5047617063463,603.396503758538,76.0023613348043));
#97892=CARTESIAN_POINT('Ctrl Pts',(-10.4588442149254,603.247407263905,76.0434598022962));
#97893=CARTESIAN_POINT('Ctrl Pts',(-10.3376554216138,603.18834726738,75.9549308895933));
#97894=CARTESIAN_POINT('Ctrl Pts',(-11.2166306018809,602.968484050211,75.3219412047775));
#97895=CARTESIAN_POINT('Ctrl Pts',(-11.1717706789499,602.810553673284,75.3678438460831));
#97896=CARTESIAN_POINT('Ctrl Pts',(-11.0382031181792,602.755169692434,75.2772723636161));
#97897=CARTESIAN_POINT('Ctrl Pts',(-11.5558920129996,602.757959408171,74.96577030963));
#97898=CARTESIAN_POINT('Ctrl Pts',(-11.5117299914059,602.595452945654,75.0135259579074));
#97899=CARTESIAN_POINT('Ctrl Pts',(-11.3720692100036,602.542108069546,74.9225466233422));
#97900=CARTESIAN_POINT('Ctrl Pts',(-12.5250601941573,602.142743928326,73.8473239435239));
#97901=CARTESIAN_POINT('Ctrl Pts',(-12.4934838485426,601.960237519276,73.890709901465));
#97902=CARTESIAN_POINT('Ctrl Pts',(-12.3258306637108,601.91947521679,73.8086323110397));
#97903=CARTESIAN_POINT('Ctrl Pts',(-13.1077845770232,601.753730803073,73.0346961932179));
#97904=CARTESIAN_POINT('Ctrl Pts',(-13.077744970774,601.562117682642,73.078286707878));
#97905=CARTESIAN_POINT('Ctrl Pts',(-12.8992879967844,601.525774448587,72.9992994563982));
#97906=CARTESIAN_POINT('Ctrl Pts',(-14.1322077025265,601.0526083829,71.2563976137341));
#97907=CARTESIAN_POINT('Ctrl Pts',(-14.1129332121865,600.839741480705,71.2991153875746));
#97908=CARTESIAN_POINT('Ctrl Pts',(-13.9074241048782,600.816201428823,71.2282105920088));
#97909=CARTESIAN_POINT('Ctrl Pts',(-14.5579479788688,600.751472223843,70.3184194820127));
#97910=CARTESIAN_POINT('Ctrl Pts',(-14.540191874148,600.531314919786,70.3605898861845));
#97911=CARTESIAN_POINT('Ctrl Pts',(-14.3263939594619,600.511437089383,70.2940353094581));
#97912=CARTESIAN_POINT('Ctrl Pts',(-15.0602487335032,600.392181562599,68.8302748068456));
#97913=CARTESIAN_POINT('Ctrl Pts',(-15.0476696916696,600.161090211342,68.873414318539));
#97914=CARTESIAN_POINT('Ctrl Pts',(-14.8207085214835,600.147816634657,68.8119251561665));
#97915=CARTESIAN_POINT('Ctrl Pts',(-15.2051396204071,600.287604348783,68.318981400867));
#97916=CARTESIAN_POINT('Ctrl Pts',(-15.1947954692115,600.052766952685,68.3589101018559));
#97917=CARTESIAN_POINT('Ctrl Pts',(-14.9632961223424,600.041978928605,68.3027032249751));
#97918=CARTESIAN_POINT('Ctrl Pts',(-15.443724690614,600.114666560778,67.273372933676));
#97919=CARTESIAN_POINT('Ctrl Pts',(-15.438260005894,599.87275398679,67.3038920930527));
#97920=CARTESIAN_POINT('Ctrl Pts',(-15.1980890660801,599.866956287625,67.2613296018157));
#97921=CARTESIAN_POINT('Ctrl Pts',(-15.535710856414,600.047555866634,66.7472152886528));
#97922=CARTESIAN_POINT('Ctrl Pts',(-15.5318361040902,599.803106749797,66.7735722504368));
#97923=CARTESIAN_POINT('Ctrl Pts',(-15.2886130183545,599.799036681608,66.7373033136078));
#97924=CARTESIAN_POINT('Ctrl Pts',(-15.6659206532499,599.95240616771,65.6882422743292));
#97925=CARTESIAN_POINT('Ctrl Pts',(-15.6650029770329,599.703836396114,65.702986948441));
#97926=CARTESIAN_POINT('Ctrl Pts',(-15.416753347311,599.702739853292,65.6826183891459));
#97927=CARTESIAN_POINT('Ctrl Pts',(-15.7041440786651,599.924364187608,65.1554257032332));
#97928=CARTESIAN_POINT('Ctrl Pts',(-15.7039435893066,599.674691055738,65.1652840040138));
#97929=CARTESIAN_POINT('Ctrl Pts',(-15.4543691947642,599.674359863803,65.1519598739898));
#97930=CARTESIAN_POINT('Ctrl Pts',(-15.725963719193,599.908367606241,64.0830042219837));
#97931=CARTESIAN_POINT('Ctrl Pts',(-15.7262805762302,599.657984756203,64.0801660974849));
#97932=CARTESIAN_POINT('Ctrl Pts',(-15.4758420566949,599.658170422961,64.0838805525614));
#97933=CARTESIAN_POINT('Ctrl Pts',(-15.7093838004202,599.920543415892,63.5413158590829));
#97934=CARTESIAN_POINT('Ctrl Pts',(-15.7093899474743,599.670639481593,63.533432145575));
#97935=CARTESIAN_POINT('Ctrl Pts',(-15.4595256835684,599.67049299479,63.5443861522047));
#97936=CARTESIAN_POINT('Ctrl Pts',(-15.5748761636817,600.019013261713,61.9191477303746));
#97937=CARTESIAN_POINT('Ctrl Pts',(-15.5720423635036,599.773215559694,61.8961392504176));
#97938=CARTESIAN_POINT('Ctrl Pts',(-15.3271559384047,599.770149902152,61.9287880982582));
#97939=CARTESIAN_POINT('Ctrl Pts',(-15.3766850183768,600.164210165805,60.8731529828927));
#97940=CARTESIAN_POINT('Ctrl Pts',(-15.3728291173236,599.922150618853,60.8481294183498));
#97941=CARTESIAN_POINT('Ctrl Pts',(-15.1321164848615,599.917095981418,60.8870337307209));
#97942=CARTESIAN_POINT('Ctrl Pts',(-14.9288646952281,600.486393343205,59.3524144284031));
#97943=CARTESIAN_POINT('Ctrl Pts',(-14.9137106754242,600.259060007561,59.3061798598269));
#97944=CARTESIAN_POINT('Ctrl Pts',(-14.6914127541727,600.24316421183,59.3724502436072));
#97945=CARTESIAN_POINT('Ctrl Pts',(-14.7530559724391,600.612143493662,58.8510846321664));
#97946=CARTESIAN_POINT('Ctrl Pts',(-14.735492592348,600.389087069143,58.8024640384097));
#97947=CARTESIAN_POINT('Ctrl Pts',(-14.5183989336226,600.370430015253,58.8731518928978));
#97948=CARTESIAN_POINT('Ctrl Pts',(-14.359091214726,600.890882373311,57.8843269848985));
#97949=CARTESIAN_POINT('Ctrl Pts',(-14.3355486906423,600.677666788424,57.831412861111));
#97950=CARTESIAN_POINT('Ctrl Pts',(-14.1306968197733,600.652528873856,57.9103117242868));
#97951=CARTESIAN_POINT('Ctrl Pts',(-14.1407177531074,601.044041513339,57.4171203625588));
#97952=CARTESIAN_POINT('Ctrl Pts',(-14.1147768511432,600.835594442267,57.3630755463199));
#97953=CARTESIAN_POINT('Ctrl Pts',(-13.9157951809153,600.807533961072,57.4449987770471));
#97954=CARTESIAN_POINT('Ctrl Pts',(-13.6634366702206,601.374137201052,56.5124852728989));
#97955=CARTESIAN_POINT('Ctrl Pts',(-13.6319576862835,601.176086556912,56.4571863827656));
#97956=CARTESIAN_POINT('Ctrl Pts',(-13.4461019523439,601.141608393448,56.5440307949745));
#97957=CARTESIAN_POINT('Ctrl Pts',(-13.4045217018066,601.551087874668,56.0750652474453));
#97958=CARTESIAN_POINT('Ctrl Pts',(-13.3709792891119,601.357985213843,56.0198511196711));
#97959=CARTESIAN_POINT('Ctrl Pts',(-13.1913037235795,601.320691655312,56.1083842943529));
#97960=CARTESIAN_POINT('Ctrl Pts',(-12.8467572513285,601.925479899478,55.2284798584221));
#97961=CARTESIAN_POINT('Ctrl Pts',(-12.8086534652092,601.742797603221,55.1745452490493));
#97962=CARTESIAN_POINT('Ctrl Pts',(-12.64240759359,601.699596004276,55.2652320085852));
#97963=CARTESIAN_POINT('Ctrl Pts',(-12.5479044351808,602.122879885018,54.8198060554334));
#97964=CARTESIAN_POINT('Ctrl Pts',(-12.5081763747874,601.945188305703,54.7668256888035));
#97965=CARTESIAN_POINT('Ctrl Pts',(-12.3483069071172,601.899374950781,54.8582156625017));
#97966=CARTESIAN_POINT('Ctrl Pts',(-11.6083463397431,602.729536752221,53.6549020913345));
#97967=CARTESIAN_POINT('Ctrl Pts',(-11.5721545818985,602.561244927479,53.6169046527624));
#97968=CARTESIAN_POINT('Ctrl Pts',(-11.4236939741492,602.513339744895,53.6980435355989));
#97969=CARTESIAN_POINT('Ctrl Pts',(-10.9203783533487,603.156822706136,52.9511800330592));
#97970=CARTESIAN_POINT('Ctrl Pts',(-10.8838506687482,602.997717916532,52.9147405141667));
#97971=CARTESIAN_POINT('Ctrl Pts',(-10.7466675601512,602.945774750955,52.9971756449448));
#97972=CARTESIAN_POINT('Ctrl Pts',(-9.79188180091539,603.807239137665,51.9938845551591));
#97973=CARTESIAN_POINT('Ctrl Pts',(-9.74600809350948,603.666006770914,51.9575122012219));
#97974=CARTESIAN_POINT('Ctrl Pts',(-9.63611348815389,603.604032067193,52.043761533861));
#97975=CARTESIAN_POINT('Ctrl Pts',(-9.39789698724152,604.026363466371,51.6904175829392));
#97976=CARTESIAN_POINT('Ctrl Pts',(-9.35238143885824,603.889218513118,51.6563518525185));
#97977=CARTESIAN_POINT('Ctrl Pts',(-9.24839501364177,603.825796888994,51.7415264001437));
#97978=CARTESIAN_POINT('Ctrl Pts',(-8.5882707639602,604.455409354432,51.1256218197328));
#97979=CARTESIAN_POINT('Ctrl Pts',(-8.54421880589914,604.325589629118,51.0970442175137));
#97980=CARTESIAN_POINT('Ctrl Pts',(-8.45164641908639,604.260012585311,51.1790240815796));
#97981=CARTESIAN_POINT('Ctrl Pts',(-8.17152248677756,604.666045668114,50.863137499133));
#97982=CARTESIAN_POINT('Ctrl Pts',(-8.12841996224356,604.539860982956,50.8368346325361));
#97983=CARTESIAN_POINT('Ctrl Pts',(-8.04152694278709,604.473187063978,50.9176054756285));
#97984=CARTESIAN_POINT('Ctrl Pts',(-6.8824505977745,605.277521007612,50.1335953878553));
#97985=CARTESIAN_POINT('Ctrl Pts',(-6.85180078127635,605.15681962248,50.1198420410442));
#97986=CARTESIAN_POINT('Ctrl Pts',(-6.77296527985932,605.092027537154,50.1910295542293));
#97987=CARTESIAN_POINT('Ctrl Pts',(-5.97236940852388,605.659075019653,49.7234080275098));
#97988=CARTESIAN_POINT('Ctrl Pts',(-5.94378154267043,605.545965583367,49.7114424968018));
#97989=CARTESIAN_POINT('Ctrl Pts',(-5.87736007948177,605.478180238876,49.7825065974709));
#97990=CARTESIAN_POINT('Ctrl Pts',(-4.50406198106329,606.142293047406,49.2314609330919));
#97991=CARTESIAN_POINT('Ctrl Pts',(-4.47704379275699,606.03766895215,49.2235345335548));
#97992=CARTESIAN_POINT('Ctrl Pts',(-4.43240690450128,605.967221696673,49.2925569652473));
#97993=CARTESIAN_POINT('Ctrl Pts',(-3.99670954179865,606.287879162115,49.088694597554));
#97994=CARTESIAN_POINT('Ctrl Pts',(-3.97216443006434,606.185409069474,49.0822732722215));
#97995=CARTESIAN_POINT('Ctrl Pts',(-3.93312549027658,606.114562082292,49.1503705419181));
#97996=CARTESIAN_POINT('Ctrl Pts',(-2.85259747095036,606.558470894243,48.8286226638388));
#97997=CARTESIAN_POINT('Ctrl Pts',(-2.83595961871912,606.459127596936,48.8258047037337));
#97998=CARTESIAN_POINT('Ctrl Pts',(-2.80721571937531,606.388413802999,48.8913556172026));
#97999=CARTESIAN_POINT('Ctrl Pts',(-2.20802541233332,606.672670497811,48.7229986861156));
#98000=CARTESIAN_POINT('Ctrl Pts',(-2.19436435103283,606.575165993762,48.7211342965073));
#98001=CARTESIAN_POINT('Ctrl Pts',(-2.17289772765275,606.50398958997,48.7861606117232));
#98002=CARTESIAN_POINT('Ctrl Pts',(-1.548495767235,606.743661819472,48.6576047836375));
#98003=CARTESIAN_POINT('Ctrl Pts',(-1.53802701918798,606.647079799347,48.6565547220104));
#98004=CARTESIAN_POINT('Ctrl Pts',(-1.52385975718171,606.575836310594,48.7210323974217));
#98005=CARTESIAN_POINT('',(1.49247642388117E-9,606.827127123144,80.0178253754844));
#98006=CARTESIAN_POINT('',(-1.91941230150446,606.698958856847,48.698800681464));
#98007=CARTESIAN_POINT('Ctrl Pts',(0.,606.827186486861,80.0177804323122));
#98008=CARTESIAN_POINT('Ctrl Pts',(-0.523838402099614,606.827186486861,
80.0177804323122));
#98009=CARTESIAN_POINT('Ctrl Pts',(-1.04370866617181,606.798326811839,79.9916639229812));
#98010=CARTESIAN_POINT('Ctrl Pts',(-2.07588373512256,606.686421518492,79.8887286024128));
#98011=CARTESIAN_POINT('Ctrl Pts',(-2.58884491618879,606.602944672362,79.8114551737427));
#98012=CARTESIAN_POINT('Ctrl Pts',(-3.58593453053115,606.392664702315,79.6117158816492));
#98013=CARTESIAN_POINT('Ctrl Pts',(-4.0730770151066,606.265685908356,79.4890655970438));
#98014=CARTESIAN_POINT('Ctrl Pts',(-5.02736864376844,605.97675047939,79.2004542940851));
#98015=CARTESIAN_POINT('Ctrl Pts',(-5.49684127598253,605.813849430916,79.0334559601684));
#98016=CARTESIAN_POINT('Ctrl Pts',(-6.85808462896243,605.292109959681,78.4766795782573));
#98017=CARTESIAN_POINT('Ctrl Pts',(-7.70355359238228,604.902197691963,78.0333468553696));
#98018=CARTESIAN_POINT('Ctrl Pts',(-8.89973254356871,604.293516577598,77.2642195998673));
#98019=CARTESIAN_POINT('Ctrl Pts',(-9.28623993692406,604.086441118006,76.9902938266832));
#98020=CARTESIAN_POINT('Ctrl Pts',(-10.0362291980326,603.668698110008,76.4058881437883));
#98021=CARTESIAN_POINT('Ctrl Pts',(-10.4000435824971,603.457751878295,76.0948005375614));
#98022=CARTESIAN_POINT('Ctrl Pts',(-11.4396209671232,602.83682855148,75.1208482803277));
#98023=CARTESIAN_POINT('Ctrl Pts',(-12.0708675035256,602.435159887223,74.4129443846916));
#98024=CARTESIAN_POINT('Ctrl Pts',(-12.9272407039081,601.871954972911,73.2539335615611));
#98025=CARTESIAN_POINT('Ctrl Pts',(-13.1974645163444,601.690741457398,72.8512918153461));
#98026=CARTESIAN_POINT('Ctrl Pts',(-13.705907162251,601.344998141025,72.0101656887144));
#98027=CARTESIAN_POINT('Ctrl Pts',(-13.9424367491172,601.181602019743,71.5740025956755));
#98028=CARTESIAN_POINT('Ctrl Pts',(-14.5877396657579,600.731202865487,70.2361076880824));
#98029=CARTESIAN_POINT('Ctrl Pts',(-14.9374786600809,600.48060273398,69.2981314957323));
#98030=CARTESIAN_POINT('Ctrl Pts',(-15.2640367599687,600.244791441604,68.0597854794833));
#98031=CARTESIAN_POINT('Ctrl Pts',(-15.3238781708752,600.201438975219,67.8080648198323));
#98032=CARTESIAN_POINT('Ctrl Pts',(-15.4305740793169,600.123978935667,67.3042760285323));
#98033=CARTESIAN_POINT('Ctrl Pts',(-15.4776212824142,600.089732808377,67.0516154405275));
#98034=CARTESIAN_POINT('Ctrl Pts',(-15.6000369014761,600.0004912733,66.2913465819385));
#98035=CARTESIAN_POINT('Ctrl Pts',(-15.6567243462522,599.958974605742,65.7814558786312));
#98036=CARTESIAN_POINT('Ctrl Pts',(-15.7200921410461,599.912552918423,64.7555336881403));
#98037=CARTESIAN_POINT('Ctrl Pts',(-15.7267764511932,599.907644658805,64.2395027071171));
#98038=CARTESIAN_POINT('Ctrl Pts',(-15.6884879697056,599.935709166568,63.2010937639321));
#98039=CARTESIAN_POINT('Ctrl Pts',(-15.6429785458214,599.969074428584,62.6781815568624));
#98040=CARTESIAN_POINT('Ctrl Pts',(-15.4329805623442,600.122406036859,61.1446179884831));
#98041=CARTESIAN_POINT('Ctrl Pts',(-15.1957463219534,600.295330691334,60.1535682172885));
#98042=CARTESIAN_POINT('Ctrl Pts',(-14.7000874693409,600.64956243217,58.7109944575794));
#98043=CARTESIAN_POINT('Ctrl Pts',(-14.5127468230508,600.782527387899,58.242003763886));
#98044=CARTESIAN_POINT('Ctrl Pts',(-14.1005377299408,601.071729059695,57.3361700731209));
#98045=CARTESIAN_POINT('Ctrl Pts',(-13.8750752636248,601.228396330728,56.8975962595972));
#98046=CARTESIAN_POINT('Ctrl Pts',(-13.1426912261625,601.729855835972,55.6221334704683));
#98047=CARTESIAN_POINT('Ctrl Pts',(-12.5757171471258,602.108922153606,54.8214953487566));
#98048=CARTESIAN_POINT('Ctrl Pts',(-11.3331559325469,602.900605352485,53.3660245246631));
#98049=CARTESIAN_POINT('Ctrl Pts',(-10.6547752361309,603.31564013608,52.7042730339687));
#98050=CARTESIAN_POINT('Ctrl Pts',(-9.54585906942516,603.944213997349,51.8027276685537));
#98051=CARTESIAN_POINT('Ctrl Pts',(-9.16098839272779,604.154506913516,51.5179512580578));
#98052=CARTESIAN_POINT('Ctrl Pts',(-8.37201911995265,604.565048924592,50.9878126575492));
#98053=CARTESIAN_POINT('Ctrl Pts',(-7.96635410967427,604.766222133218,50.7411093620899));
#98054=CARTESIAN_POINT('Ctrl Pts',(-6.71291294709257,605.349307836359,50.0548419703803));
#98055=CARTESIAN_POINT('Ctrl Pts',(-5.82961165971477,605.711811288536,49.6681929464691));
#98056=CARTESIAN_POINT('Ctrl Pts',(-4.40836677555933,606.170246586049,49.2037840375558));
#98057=CARTESIAN_POINT('Ctrl Pts',(-3.91938654325121,606.30783645178,49.0692534214259));
#98058=CARTESIAN_POINT('Ctrl Pts',(-2.93166846065344,606.537737419501,48.8486963579089));
#98059=CARTESIAN_POINT('Ctrl Pts',(-2.42992069874045,606.63106204052,48.7616105405085));
#98060=CARTESIAN_POINT('Ctrl Pts',(-1.91941230150446,606.698958856847,48.698800681464));
#98061=CARTESIAN_POINT('',(-1.8888840075986,606.53066176659,48.7620619651123));
#98062=CARTESIAN_POINT('Origin',(-1.88888400761935,606.698958856848,48.9469297270682));
#98063=CARTESIAN_POINT('',(1.86306288877797,606.534169754924,79.840079036097));
#98064=CARTESIAN_POINT('Ctrl Pts',(-1.8888840075986,606.53066176659,48.7620619651123));
#98065=CARTESIAN_POINT('Ctrl Pts',(-2.41149695900853,606.45918119815,48.8271353535257));
#98066=CARTESIAN_POINT('Ctrl Pts',(-2.9244450266129,606.359900440675,48.9183242031726));
#98067=CARTESIAN_POINT('Ctrl Pts',(-3.42867105811377,606.237260990053,49.0343192413469));
#98068=CARTESIAN_POINT('Ctrl Pts',(-3.43116315307001,606.236654854834,49.0348925371141));
#98069=CARTESIAN_POINT('Ctrl Pts',(-3.43365511556903,606.236048119746,49.0354664692823));
#98070=CARTESIAN_POINT('Ctrl Pts',(-3.43614694410228,606.235440785882,49.0360410372358));
#98071=CARTESIAN_POINT('Ctrl Pts',(-3.82123395676472,606.141583451774,49.1248347298391));
#98072=CARTESIAN_POINT('Ctrl Pts',(-4.20323008343107,606.033396925328,49.2288408126609));
#98073=CARTESIAN_POINT('Ctrl Pts',(-4.57646776406636,605.914924717136,49.3457763159031));
#98074=CARTESIAN_POINT('Ctrl Pts',(-4.68985979718866,605.878932090313,49.381302081775));
#98075=CARTESIAN_POINT('Ctrl Pts',(-4.80244368080559,605.841990257397,49.4180209911653));
#98076=CARTESIAN_POINT('Ctrl Pts',(-4.91406129959471,605.804212857108,49.4558685205457));
#98077=CARTESIAN_POINT('Ctrl Pts',(-4.91843568064348,605.802732331492,49.4573517945759));
#98078=CARTESIAN_POINT('Ctrl Pts',(-4.92280863589928,605.801250575485,49.4588367478035));
#98079=CARTESIAN_POINT('Ctrl Pts',(-4.92718016685644,605.799767592365,49.4603233795273));
#98080=CARTESIAN_POINT('Ctrl Pts',(-5.42040916321487,605.632446284766,49.6280563500277));
#98081=CARTESIAN_POINT('Ctrl Pts',(-5.89557048330097,605.449497266521,49.8171650183942));
#98082=CARTESIAN_POINT('Ctrl Pts',(-6.35515504475826,605.255478405036,50.0267811577471));
#98083=CARTESIAN_POINT('Ctrl Pts',(-6.78955134201509,605.072093056409,50.2249089505768));
#98084=CARTESIAN_POINT('Ctrl Pts',(-7.21003104626367,604.878817257618,50.4413581653025));
#98085=CARTESIAN_POINT('Ctrl Pts',(-7.61867416252443,604.679468187595,50.6754123677936));
#98086=CARTESIAN_POINT('Ctrl Pts',(-7.62456670988117,604.676593616144,50.6787873799187));
#98087=CARTESIAN_POINT('Ctrl Pts',(-7.63045674519379,604.673717724625,50.682166103682));
#98088=CARTESIAN_POINT('Ctrl Pts',(-7.63634427132602,604.670840521053,50.6855485406359));
#98089=CARTESIAN_POINT('Ctrl Pts',(-8.05314726616496,604.467151053103,50.9250056267778));
#98090=CARTESIAN_POINT('Ctrl Pts',(-8.45740792076493,604.256872635283,51.1830917656922));
#98091=CARTESIAN_POINT('Ctrl Pts',(-8.85002243750457,604.042905930577,51.4602736948679));
#98092=CARTESIAN_POINT('Ctrl Pts',(-8.85593145106616,604.039685641704,51.4644453994501));
#98093=CARTESIAN_POINT('Ctrl Pts',(-8.86183806655528,604.036464358004,51.4686216821428));
#98094=CARTESIAN_POINT('Ctrl Pts',(-8.8677422613673,604.033242102544,51.4728025248131));
#98095=CARTESIAN_POINT('Ctrl Pts',(-9.23018926554603,603.835434124481,51.7294563021764));
#98096=CARTESIAN_POINT('Ctrl Pts',(-9.58363022322654,603.633898543708,52.0033825468461));
#98097=CARTESIAN_POINT('Ctrl Pts',(-9.92280720323148,603.433969241314,52.2903964742726));
#98098=CARTESIAN_POINT('Ctrl Pts',(-9.95073667621177,603.417506095587,52.3140305892144));
#98099=CARTESIAN_POINT('Ctrl Pts',(-9.97856945642496,603.401053828896,52.3377534407258));
#98100=CARTESIAN_POINT('Ctrl Pts',(-10.0063026234584,603.384615411585,52.3615626894153));
#98101=CARTESIAN_POINT('Ctrl Pts',(-10.0117904989737,603.381362555978,52.3662740948153));
#98102=CARTESIAN_POINT('Ctrl Pts',(-10.0172748471287,603.378110078954,52.3709890470135));
#98103=CARTESIAN_POINT('Ctrl Pts',(-10.0227556688064,603.374857987524,52.3757075484961));
#98104=CARTESIAN_POINT('Ctrl Pts',(-10.4844704326174,603.10089566681,52.7732030200994));
#98105=CARTESIAN_POINT('Ctrl Pts',(-10.9212653118694,602.829618351376,53.1959678505452));
#98106=CARTESIAN_POINT('Ctrl Pts',(-11.3338346746107,602.565105027701,53.6456472273239));
#98107=CARTESIAN_POINT('Ctrl Pts',(-11.5776710652414,602.408772590193,53.911416346597));
#98108=CARTESIAN_POINT('Ctrl Pts',(-11.8130457209473,602.254802291871,54.1865861674907));
#98109=CARTESIAN_POINT('Ctrl Pts',(-12.040104661015,602.104030570697,54.4714903191273));
#98110=CARTESIAN_POINT('Ctrl Pts',(-12.0438323006949,602.101555342677,54.4761676069729));
#98111=CARTESIAN_POINT('Ctrl Pts',(-12.0475578528827,602.099080844204,54.4808478324097));
#98112=CARTESIAN_POINT('Ctrl Pts',(-12.0512813078029,602.096607084918,54.4855309851298));
#98113=CARTESIAN_POINT('Ctrl Pts',(-12.3319606431896,601.910131586404,54.8385537076184));
#98114=CARTESIAN_POINT('Ctrl Pts',(-12.6007933233764,601.727806201388,55.2083103080585));
#98115=CARTESIAN_POINT('Ctrl Pts',(-12.8535510646359,601.553786258449,55.5903491042369));
#98116=CARTESIAN_POINT('Ctrl Pts',(-12.8747668387784,601.539179513716,55.6224163666401));
#98117=CARTESIAN_POINT('Ctrl Pts',(-12.8958693833388,601.524631267288,55.6545701590746));
#98118=CARTESIAN_POINT('Ctrl Pts',(-12.9168562126465,601.510143966277,55.6868078477631));
#98119=CARTESIAN_POINT('Ctrl Pts',(-12.9194398545994,601.50836046682,55.6907765580309));
#98120=CARTESIAN_POINT('Ctrl Pts',(-12.922021743077,601.506577894755,55.6947464964152));
#98121=CARTESIAN_POINT('Ctrl Pts',(-12.9246018778219,601.504796251497,55.6987176634258));
#98122=CARTESIAN_POINT('Ctrl Pts',(-13.1962036721651,601.31724887374,56.1167485774522));
#98123=CARTESIAN_POINT('Ctrl Pts',(-13.4484034732778,601.139972120339,56.5484436861926));
#98124=CARTESIAN_POINT('Ctrl Pts',(-13.680948979807,600.974571248321,56.9945145943681));
#98125=CARTESIAN_POINT('Ctrl Pts',(-13.6823423951751,600.97358016438,56.9971874564155));
#98126=CARTESIAN_POINT('Ctrl Pts',(-13.6837351051094,600.972589506321,56.9998608343006));
#98127=CARTESIAN_POINT('Ctrl Pts',(-13.6851271093878,600.97159927454,57.0025347282826));
#98128=CARTESIAN_POINT('Ctrl Pts',(-13.9184371521736,600.805629224882,57.4506988101028));
#98129=CARTESIAN_POINT('Ctrl Pts',(-14.1319267819666,600.651633932193,57.9133662944617));
#98130=CARTESIAN_POINT('Ctrl Pts',(-14.3245484115035,600.511479503361,58.3917316078811));
#98131=CARTESIAN_POINT('Ctrl Pts',(-14.3248720257519,600.51124403671,58.3925352862205));
#98132=CARTESIAN_POINT('Ctrl Pts',(-14.3251955816966,600.511008608642,58.393339013801));
#98133=CARTESIAN_POINT('Ctrl Pts',(-14.3255190793133,600.51077321918,58.3941427905652));
#98134=CARTESIAN_POINT('Ctrl Pts',(-14.5183947849969,600.37042934596,58.8733704651744));
#98135=CARTESIAN_POINT('Ctrl Pts',(-14.6905438911395,600.243803913954,59.3700945593781));
#98136=CARTESIAN_POINT('Ctrl Pts',(-14.8368369280143,600.135568860125,59.8722326143599));
#98137=CARTESIAN_POINT('Ctrl Pts',(-14.8373300871407,600.135203995838,59.8739253399318));
#98138=CARTESIAN_POINT('Ctrl Pts',(-14.8378229525661,600.134839340462,59.8756181274375));
#98139=CARTESIAN_POINT('Ctrl Pts',(-14.8383155240927,600.134474894177,59.8773109764116));
#98140=CARTESIAN_POINT('Ctrl Pts',(-15.0414396046863,599.984186433293,60.5753992192415));
#98141=CARTESIAN_POINT('Ctrl Pts',(-15.1973006598741,599.867605992967,61.2886164434837));
#98142=CARTESIAN_POINT('Ctrl Pts',(-15.3033244732793,599.788005372271,62.0179657611667));
#98143=CARTESIAN_POINT('Ctrl Pts',(-15.3495814983162,599.753276495935,62.3361728560179));
#98144=CARTESIAN_POINT('Ctrl Pts',(-15.3863525773886,599.725586246286,62.6574505117789));
#98145=CARTESIAN_POINT('Ctrl Pts',(-15.4134262294948,599.705204325428,62.9818812830931));
#98146=CARTESIAN_POINT('Ctrl Pts',(-15.4140928759569,599.704702452412,62.989869884891));
#98147=CARTESIAN_POINT('Ctrl Pts',(-15.4147536449623,599.704205007555,62.997860444859));
#98148=CARTESIAN_POINT('Ctrl Pts',(-15.4154085331436,599.703711995057,63.0058529638405));
#98149=CARTESIAN_POINT('Ctrl Pts',(-15.4549862599016,599.673917116299,63.4888754727571));
#98150=CARTESIAN_POINT('Ctrl Pts',(-15.4721900515042,599.660932130311,63.9727246693828));
#98151=CARTESIAN_POINT('Ctrl Pts',(-15.4675657250193,599.664413653428,64.4526573526759));
#98152=CARTESIAN_POINT('Ctrl Pts',(-15.4671428394911,599.664732031844,64.496546249141));
#98153=CARTESIAN_POINT('Ctrl Pts',(-15.4665374395127,599.665188093949,64.5404023977502));
#98154=CARTESIAN_POINT('Ctrl Pts',(-15.465749959502,599.665781564301,64.5842221752744));
#98155=CARTESIAN_POINT('Ctrl Pts',(-15.4655480571059,599.665933724463,64.5954571500792));
#98156=CARTESIAN_POINT('Ctrl Pts',(-15.4653341842431,599.666094919118,64.6066898685709));
#98157=CARTESIAN_POINT('Ctrl Pts',(-15.4651083473515,599.666265144236,64.6179202686375));
#98158=CARTESIAN_POINT('Ctrl Pts',(-15.4565102683663,599.672745967626,65.0454848978372));
#98159=CARTESIAN_POINT('Ctrl Pts',(-15.4306782059201,599.692234295056,65.4710177591388));
#98160=CARTESIAN_POINT('Ctrl Pts',(-15.3878202693317,599.724471888615,65.8944225395669));
#98161=CARTESIAN_POINT('Ctrl Pts',(-15.3786070250364,599.731402059515,65.9854425929899));
#98162=CARTESIAN_POINT('Ctrl Pts',(-15.3686071189849,599.738921295213,66.0763643200901));
#98163=CARTESIAN_POINT('Ctrl Pts',(-15.3578228674146,599.747026843009,66.1671867939494));
#98164=CARTESIAN_POINT('Ctrl Pts',(-15.3561295795732,599.74829953453,66.1814472727328));
#98165=CARTESIAN_POINT('Ctrl Pts',(-15.3544169428895,599.749586685959,66.1957053639419));
#98166=CARTESIAN_POINT('Ctrl Pts',(-15.3526849656753,599.750888287307,66.209961068781));
#98167=CARTESIAN_POINT('Ctrl Pts',(-15.2907263898706,599.797450889354,66.7199349654947));
#98168=CARTESIAN_POINT('Ctrl Pts',(-15.2040176992693,599.862508071703,67.2268545417177));
#98169=CARTESIAN_POINT('Ctrl Pts',(-15.0921759771049,599.945907616897,67.7306968564119));
#98170=CARTESIAN_POINT('Ctrl Pts',(-15.0883779410082,599.948739784329,67.7478068513332));
#98171=CARTESIAN_POINT('Ctrl Pts',(-15.0845508622971,599.951593143233,67.7649135318261));
#98172=CARTESIAN_POINT('Ctrl Pts',(-15.0806947254962,599.954467687614,67.7820168863499));
#98173=CARTESIAN_POINT('Ctrl Pts',(-14.9906512622063,600.0215902885,68.18139205241));
#98174=CARTESIAN_POINT('Ctrl Pts',(-14.8857494405989,600.099522550423,68.5741722445984));
#98175=CARTESIAN_POINT('Ctrl Pts',(-14.7673626316929,600.186916360206,68.9585381212224));
#98176=CARTESIAN_POINT('Ctrl Pts',(-14.7373499494797,600.209071891423,69.0559801505778));
#98177=CARTESIAN_POINT('Ctrl Pts',(-14.7064707999309,600.231835360312,69.152881479814));
#98178=CARTESIAN_POINT('Ctrl Pts',(-14.6747479525069,600.255184517968,69.2492126559159));
#98179=CARTESIAN_POINT('Ctrl Pts',(-14.6685113493146,600.259774882422,69.2681510353232));
#98180=CARTESIAN_POINT('Ctrl Pts',(-14.6622419924248,600.264387994604,69.2870678366535));
#98181=CARTESIAN_POINT('Ctrl Pts',(-14.6559400474473,600.269023690891,69.3059628438942));
#98182=CARTESIAN_POINT('Ctrl Pts',(-14.4881365257408,600.392459577008,69.8090850972572));
#98183=CARTESIAN_POINT('Ctrl Pts',(-14.2970453980955,600.532137247967,70.2985271979679));
#98184=CARTESIAN_POINT('Ctrl Pts',(-14.0832076583593,600.686446678114,70.7748546652877));
#98185=CARTESIAN_POINT('Ctrl Pts',(-13.8873140841882,600.827807252899,71.2112111763704));
#98186=CARTESIAN_POINT('Ctrl Pts',(-13.672331791668,600.981446349243,71.6365621257633));
#98187=CARTESIAN_POINT('Ctrl Pts',(-13.4387032223677,601.146104556008,72.0513594656846));
#98188=CARTESIAN_POINT('Ctrl Pts',(-13.4269732670318,601.154371667418,72.0721854900244));
#98189=CARTESIAN_POINT('Ctrl Pts',(-13.4151954394702,601.162667108948,72.0929863162258));
#98190=CARTESIAN_POINT('Ctrl Pts',(-13.4033698516022,601.170990683808,72.1137618746436));
#98191=CARTESIAN_POINT('Ctrl Pts',(-13.2658603218258,601.267778334276,72.3553428683983));
#98192=CARTESIAN_POINT('Ctrl Pts',(-13.1230592827393,601.367544932225,72.5914514645205));
#98193=CARTESIAN_POINT('Ctrl Pts',(-12.9752216473718,601.469860105797,72.8220741360305));
#98194=CARTESIAN_POINT('Ctrl Pts',(-12.8657608690502,601.545615501272,72.9928299591965));
#98195=CARTESIAN_POINT('Ctrl Pts',(-12.7535396983437,601.622767571966,73.1605791986362));
#98196=CARTESIAN_POINT('Ctrl Pts',(-12.6386729408157,601.701135811342,73.3253295048864));
#98197=CARTESIAN_POINT('Ctrl Pts',(-12.4290296027772,601.844165697905,73.6260153158943));
#98198=CARTESIAN_POINT('Ctrl Pts',(-12.2103932272426,601.991362007103,73.9169651025679));
#98199=CARTESIAN_POINT('Ctrl Pts',(-11.9829905178613,602.141928579844,74.1987899101));
#98200=CARTESIAN_POINT('Ctrl Pts',(-11.9030428234133,602.194863087019,74.2978707155211));
#98201=CARTESIAN_POINT('Ctrl Pts',(-11.8220112796174,602.24821427354,74.3958233320019));
#98202=CARTESIAN_POINT('Ctrl Pts',(-11.7399047075142,602.301947835157,74.4926732578091));
#98203=CARTESIAN_POINT('Ctrl Pts',(-11.723313317863,602.312805850968,74.512243857526));
#98204=CARTESIAN_POINT('Ctrl Pts',(-11.7066783200462,602.323679189369,74.5317689045803));
#98205=CARTESIAN_POINT('Ctrl Pts',(-11.6899998492773,602.3345675332,74.5512485570586));
#98206=CARTESIAN_POINT('Ctrl Pts',(-11.3893716288856,602.530829137398,74.9023678736653));
#98207=CARTESIAN_POINT('Ctrl Pts',(-11.0743064696377,602.732118822314,75.2388277121095));
#98208=CARTESIAN_POINT('Ctrl Pts',(-10.7444640677328,602.936745911554,75.5611408646035));
#98209=CARTESIAN_POINT('Ctrl Pts',(-10.7256680559147,602.94840655059,75.5795078234554));
#98210=CARTESIAN_POINT('Ctrl Pts',(-10.706824102173,602.960077953694,75.5978287367274));
#98211=CARTESIAN_POINT('Ctrl Pts',(-10.687932101418,602.97175982427,75.6161037296602));
#98212=CARTESIAN_POINT('Ctrl Pts',(-10.391643904776,603.154969660612,75.9027152310002));
#98213=CARTESIAN_POINT('Ctrl Pts',(-10.0822730964368,603.341485904188,76.1790010607769));
#98214=CARTESIAN_POINT('Ctrl Pts',(-9.76302160159852,603.527656477313,76.4419445958769));
#98215=CARTESIAN_POINT('Ctrl Pts',(-9.72558983078315,603.549484704708,76.472774340772));
#98216=CARTESIAN_POINT('Ctrl Pts',(-9.68802222053652,603.571308158203,76.503420611066));
#98217=CARTESIAN_POINT('Ctrl Pts',(-9.65032392871191,603.593120930745,76.5338784979795));
#98218=CARTESIAN_POINT('Ctrl Pts',(-9.62962043291993,603.605100270462,76.5506056413864));
#98219=CARTESIAN_POINT('Ctrl Pts',(-9.60887807747269,603.617076106053,76.5672755719517));
#98220=CARTESIAN_POINT('Ctrl Pts',(-9.58809774349921,603.629047449649,76.5838874705586));
#98221=CARTESIAN_POINT('Ctrl Pts',(-9.17209645664058,603.868701650953,76.9164408937348));
#98222=CARTESIAN_POINT('Ctrl Pts',(-8.74167731913442,604.106495599033,77.2259224192872));
#98223=CARTESIAN_POINT('Ctrl Pts',(-8.29525516685564,604.338636728732,77.5129331902665));
#98224=CARTESIAN_POINT('Ctrl Pts',(-7.94596840716844,604.520267103858,77.7374943185145));
#98225=CARTESIAN_POINT('Ctrl Pts',(-7.58688458985845,604.698436781484,77.9482988748373));
#98226=CARTESIAN_POINT('Ctrl Pts',(-7.21723077844874,604.871316351623,78.1456225473664));
#98227=CARTESIAN_POINT('Ctrl Pts',(-7.19435330607696,604.882015680204,78.1578346948602));
#98228=CARTESIAN_POINT('Ctrl Pts',(-7.17143531739344,604.89269462405,78.1699950695054));
#98229=CARTESIAN_POINT('Ctrl Pts',(-7.1484766436231,604.903352752914,78.1821037431292));
#98230=CARTESIAN_POINT('Ctrl Pts',(-6.75967649946682,605.083845845844,78.3871614959228));
#98231=CARTESIAN_POINT('Ctrl Pts',(-6.35908010474382,605.258272755171,78.5772453811039));
#98232=CARTESIAN_POINT('Ctrl Pts',(-5.94486173928286,605.423622180316,78.7517442440193));
#98233=CARTESIAN_POINT('Ctrl Pts',(-5.92075101065575,605.433246802136,78.7619014342366));
#98234=CARTESIAN_POINT('Ctrl Pts',(-5.89659411591536,605.442840663064,78.7720058150056));
#98235=CARTESIAN_POINT('Ctrl Pts',(-5.87239069016909,605.452403167251,78.7820572638862));
#98236=CARTESIAN_POINT('Ctrl Pts',(-5.8489383682211,605.461668918686,78.7917967866158));
#98237=CARTESIAN_POINT('Ctrl Pts',(-5.82544172188546,605.470905403857,78.801486795087));
#98238=CARTESIAN_POINT('Ctrl Pts',(-5.8019005095584,605.480112026635,78.8111271194742));
#98239=CARTESIAN_POINT('Ctrl Pts',(-5.52092170778195,605.589998713896,78.9261903013284));
#98240=CARTESIAN_POINT('Ctrl Pts',(-5.23391572238947,605.695391403333,79.0339059074638));
#98241=CARTESIAN_POINT('Ctrl Pts',(-4.9427116750574,605.794468591044,79.1333013998922));
#98242=CARTESIAN_POINT('Ctrl Pts',(-4.77501441594139,605.851524710189,79.1905408229065));
#98243=CARTESIAN_POINT('Ctrl Pts',(-4.60592561275599,605.906486672614,79.2450216198832));
#98244=CARTESIAN_POINT('Ctrl Pts',(-4.43579829675243,605.959010640085,79.296563818299));
#98245=CARTESIAN_POINT('Ctrl Pts',(-4.41274763656984,605.966127146441,79.3035473041298));
#98246=CARTESIAN_POINT('Ctrl Pts',(-4.38967592729236,605.973199574385,79.3104775101188));
#98247=CARTESIAN_POINT('Ctrl Pts',(-4.36658401678448,605.980227058812,79.3173539744283));
#98248=CARTESIAN_POINT('Ctrl Pts',(-4.04882336544269,606.076930102417,79.4119788768226));
#98249=CARTESIAN_POINT('Ctrl Pts',(-3.72622839314485,606.165533628874,79.4968684248683));
#98250=CARTESIAN_POINT('Ctrl Pts',(-3.39848998478872,606.244581226598,79.5715572830011));
#98251=CARTESIAN_POINT('Ctrl Pts',(-3.24344222817048,606.281977370537,79.6068913775186));
#98252=CARTESIAN_POINT('Ctrl Pts',(-3.0872435683354,606.317235184592,79.6399430181275));
#98253=CARTESIAN_POINT('Ctrl Pts',(-2.92986272136945,606.350202891215,79.670666001624));
#98254=CARTESIAN_POINT('Ctrl Pts',(-2.90796583102345,606.354789791533,79.6749405865795));
#98255=CARTESIAN_POINT('Ctrl Pts',(-2.8860468670402,606.359332262393,79.6791700030137));
#98256=CARTESIAN_POINT('Ctrl Pts',(-2.86410536448453,606.36382997616,79.6833542027662));
#98257=CARTESIAN_POINT('Ctrl Pts',(-2.67077137140168,606.403460851943,79.7202226006324));
#98258=CARTESIAN_POINT('Ctrl Pts',(-2.47523365108864,606.439601026273,79.7535703438643));
#98259=CARTESIAN_POINT('Ctrl Pts',(-2.27824761486158,606.471936730464,79.7832366450388));
#98260=CARTESIAN_POINT('Ctrl Pts',(-2.09244054750841,606.502437381585,79.811219381917));
#98261=CARTESIAN_POINT('Ctrl Pts',(-1.9053436242915,606.529553234617,79.8359266171057));
#98262=CARTESIAN_POINT('Ctrl Pts',(-1.71759256271035,606.552987944339,79.857193117338));
#98263=CARTESIAN_POINT('Ctrl Pts',(-1.59648021957914,606.568104943312,79.8709114721193));
#98264=CARTESIAN_POINT('Ctrl Pts',(-1.47509576548736,606.581689501849,79.8831974849582));
#98265=CARTESIAN_POINT('Ctrl Pts',(-1.35361376683637,606.593653739294,79.8939995839849));
#98266=CARTESIAN_POINT('Ctrl Pts',(-1.3347974152013,606.595506880511,79.8956727215357));
#98267=CARTESIAN_POINT('Ctrl Pts',(-1.31597645205385,606.597321531768,79.8973106052341));
#98268=CARTESIAN_POINT('Ctrl Pts',(-1.29715200364571,606.599097281125,79.8989129667661));
#98269=CARTESIAN_POINT('Ctrl Pts',(-1.11523121238239,606.616258247602,79.9143983011279));
#98270=CARTESIAN_POINT('Ctrl Pts',(-0.932588982072346,606.629864250476,
79.9267009011115));
#98271=CARTESIAN_POINT('Ctrl Pts',(-0.749467854777604,606.639830437194,
79.9357300191261));
#98272=CARTESIAN_POINT('Ctrl Pts',(-0.683607177593734,606.643414839584,
79.9389773988009));
#98273=CARTESIAN_POINT('Ctrl Pts',(-0.617684568111035,606.646528786564,
79.9418016685007));
#98274=CARTESIAN_POINT('Ctrl Pts',(-0.551711358599842,606.649169564796,
79.9441997051945));
#98275=CARTESIAN_POINT('Ctrl Pts',(-0.345342966588009,606.657430086932,
79.9517009163702));
#98276=CARTESIAN_POINT('Ctrl Pts',(-0.138423353440868,606.661078221085,
79.9550471976344));
#98277=CARTESIAN_POINT('Ctrl Pts',(0.0688418019391206,606.660027049308,
79.9541394471178));
#98278=CARTESIAN_POINT('Ctrl Pts',(0.131131170307284,606.6597111408,79.953866640981));
#98279=CARTESIAN_POINT('Ctrl Pts',(0.193451665010783,606.658971058177,79.9532098508916));
#98280=CARTESIAN_POINT('Ctrl Pts',(0.255797490386203,606.657805108831,79.9521669823773));
#98281=CARTESIAN_POINT('Ctrl Pts',(0.666136198923766,606.650131232575,79.945303181686));
#98282=CARTESIAN_POINT('Ctrl Pts',(1.07421972549342,606.624141270417,79.921831977901));
#98283=CARTESIAN_POINT('Ctrl Pts',(1.48012296273393,606.580564567151,79.8822570048524));
#98284=CARTESIAN_POINT('Ctrl Pts',(1.60798473410058,606.566837663893,79.8697906688108));
#98285=CARTESIAN_POINT('Ctrl Pts',(1.73563038646646,606.551365380786,79.8557262296395));
#98286=CARTESIAN_POINT('Ctrl Pts',(1.86306288877797,606.534169754924,79.840079036097));
#98287=CARTESIAN_POINT('',(1.89317385967765,606.70242510632,79.9033533194805));
#98288=CARTESIAN_POINT('Origin',(1.86306288877797,606.70242510632,79.6551732851678));
#98289=CARTESIAN_POINT('Ctrl Pts',(1.89317385967764,606.70242510632,79.9033533194805));
#98290=CARTESIAN_POINT('Ctrl Pts',(1.58012448505219,606.743501216302,79.9413347011642));
#98291=CARTESIAN_POINT('Ctrl Pts',(1.26585353386947,606.774601642493,79.9700061023909));
#98292=CARTESIAN_POINT('Ctrl Pts',(0.950335111694906,606.795445530877,79.9891761306859));
#98293=CARTESIAN_POINT('Ctrl Pts',(0.78817740514306,606.806158050014,79.9990283852751));
#98294=CARTESIAN_POINT('Ctrl Pts',(0.625503300952601,606.814170420382,80.0063792748621));
#98295=CARTESIAN_POINT('Ctrl Pts',(0.462595958335336,606.819424912887,80.0111851918326));
#98296=CARTESIAN_POINT('Ctrl Pts',(0.308526274104866,606.824394351269,80.0157303897235));
#98297=CARTESIAN_POINT('Ctrl Pts',(0.154247965606297,606.826897303316,80.0179995314596));
#98298=CARTESIAN_POINT('Ctrl Pts',(6.79067047038018E-9,606.826916385848,
80.0179849207937));
#98299=CARTESIAN_POINT('Ctrl Pts',(-0.247612686332898,604.134451125088,
76.5969814761947));
#98300=CARTESIAN_POINT('Ctrl Pts',(-0.239928764978578,603.631174020018,
76.5971361934352));
#98301=CARTESIAN_POINT('Ctrl Pts',(-0.252645464510396,603.935273498433,
76.9980210944396));
#98302=CARTESIAN_POINT('Ctrl Pts',(0.587407127222549,604.147464416195,76.613794761412));
#98303=CARTESIAN_POINT('Ctrl Pts',(0.570806075610003,603.642504151856,76.6129375177081));
#98304=CARTESIAN_POINT('Ctrl Pts',(0.599346104179961,603.948443486134,77.0153826803362));
#98305=CARTESIAN_POINT('Ctrl Pts',(1.40663729476956,604.094168032195,76.5461272140149));
#98306=CARTESIAN_POINT('Ctrl Pts',(1.3489476199593,603.598226411249,76.5522413898123));
#98307=CARTESIAN_POINT('Ctrl Pts',(1.43522748368769,603.894505336773,76.9455084004709));
#98308=CARTESIAN_POINT('Ctrl Pts',(2.61366069407739,603.927699846335,76.3255317586155));
#98309=CARTESIAN_POINT('Ctrl Pts',(2.53731328870643,603.450528037425,76.3416431735781));
#98310=CARTESIAN_POINT('Ctrl Pts',(2.66678387891633,603.726032622645,76.7177190065359));
#98311=CARTESIAN_POINT('Ctrl Pts',(3.01445595206078,603.857371670206,76.2313414391483));
#98312=CARTESIAN_POINT('Ctrl Pts',(2.92857212557764,603.388846213913,76.2529152101653));
#98313=CARTESIAN_POINT('Ctrl Pts',(3.07572538189221,603.654857589732,76.6204570030234));
#98314=CARTESIAN_POINT('Ctrl Pts',(3.7983954194345,603.69287182511,76.0053954703534));
#98315=CARTESIAN_POINT('Ctrl Pts',(3.70006557576271,603.242083137045,76.0368396544836));
#98316=CARTESIAN_POINT('Ctrl Pts',(3.8755985784546,603.488376918241,76.3871426082101));
#98317=CARTESIAN_POINT('Ctrl Pts',(4.17984986817795,603.599268233769,75.874409667253));
#98318=CARTESIAN_POINT('Ctrl Pts',(4.07641784659729,603.158465786143,75.9117507781356));
#98319=CARTESIAN_POINT('Ctrl Pts',(4.26480616625281,603.393646199154,76.2518851665813));
#98320=CARTESIAN_POINT('Ctrl Pts',(4.92370189566428,603.394079103706,75.5781015854782));
#98321=CARTESIAN_POINT('Ctrl Pts',(4.81486847221986,602.972538673971,75.6252072189681));
#98322=CARTESIAN_POINT('Ctrl Pts',(5.02377713750492,603.185986282303,75.9459140475635));
#98323=CARTESIAN_POINT('Ctrl Pts',(5.28609505655054,603.282487531454,75.4127725629522));
#98324=CARTESIAN_POINT('Ctrl Pts',(5.17578544904304,602.871110243873,75.4653304964425));
#98325=CARTESIAN_POINT('Ctrl Pts',(5.39353601298289,603.073050979998,75.7751934044062));
#98326=CARTESIAN_POINT('Ctrl Pts',(5.99304821798366,603.045463077024,75.0480357125633));
#98327=CARTESIAN_POINT('Ctrl Pts',(5.88314832657038,602.653172554016,75.1089592769933));
#98328=CARTESIAN_POINT('Ctrl Pts',(6.11485814111501,602.833172393456,75.398561954746));
#98329=CARTESIAN_POINT('Ctrl Pts',(6.33872452185387,602.919536364403,74.8477580011569));
#98330=CARTESIAN_POINT('Ctrl Pts',(6.23031283838703,602.536883703424,74.9130743719703));
#98331=CARTESIAN_POINT('Ctrl Pts',(6.46756038601705,602.705729334106,75.1917528950879));
#98332=CARTESIAN_POINT('Ctrl Pts',(7.33337757366972,602.533334747895,74.2057580358069));
#98333=CARTESIAN_POINT('Ctrl Pts',(7.21704842590842,602.182602812065,74.2897410752272));
#98334=CARTESIAN_POINT('Ctrl Pts',(7.48242996358273,602.314877267486,74.5288163772505));
#98335=CARTESIAN_POINT('Ctrl Pts',(7.94559727067024,602.263368546861,73.721359506763));
#98336=CARTESIAN_POINT('Ctrl Pts',(7.84051708959433,601.928604105213,73.8120742692735));
#98337=CARTESIAN_POINT('Ctrl Pts',(8.10709315029709,602.041660267919,74.028620906189));
#98338=CARTESIAN_POINT('Ctrl Pts',(8.79441170737145,601.860736855362,72.9077220474778));
#98339=CARTESIAN_POINT('Ctrl Pts',(8.71531793774959,601.540974637517,72.9883352789045));
#98340=CARTESIAN_POINT('Ctrl Pts',(8.97315991273498,601.634180283339,73.188449545123));
#98341=CARTESIAN_POINT('Ctrl Pts',(9.06684564649771,601.726233572703,72.6204124471552));
#98342=CARTESIAN_POINT('Ctrl Pts',(8.99305377021651,601.412739404795,72.7011730151351));
#98343=CARTESIAN_POINT('Ctrl Pts',(9.25113112703224,601.498057379104,72.8917703602215));
#98344=CARTESIAN_POINT('Ctrl Pts',(9.58153921876773,601.464380717656,72.0221557047211));
#98345=CARTESIAN_POINT('Ctrl Pts',(9.51738335439514,601.162565769111,72.1016116954675));
#98346=CARTESIAN_POINT('Ctrl Pts',(9.77628595094184,601.233051420721,72.2740035948496));
#98347=CARTESIAN_POINT('Ctrl Pts',(9.82332486871901,601.337330579973,71.7120858574342));
#98348=CARTESIAN_POINT('Ctrl Pts',(9.76463235697413,601.040586840631,71.7902694724233));
#98349=CARTESIAN_POINT('Ctrl Pts',(10.0229859433045,601.104471408494,71.9538219181877));
#98350=CARTESIAN_POINT('Ctrl Pts',(10.5032304581882,600.971778124982,70.7485243138466));
#98351=CARTESIAN_POINT('Ctrl Pts',(10.4508934408169,600.693428016039,70.8323532494638));
#98352=CARTESIAN_POINT('Ctrl Pts',(10.7167107520177,600.734517150472,70.9588372302021));
#98353=CARTESIAN_POINT('Ctrl Pts',(10.8964735613622,600.748744139839,70.0620801831889));
#98354=CARTESIAN_POINT('Ctrl Pts',(10.8576198832383,600.476090849664,70.138628472291));
#98355=CARTESIAN_POINT('Ctrl Pts',(11.1179466017888,600.508797501419,70.250007157043));
#98356=CARTESIAN_POINT('Ctrl Pts',(11.390954790485,600.461487996467,68.957675482628));
#98357=CARTESIAN_POINT('Ctrl Pts',(11.3677587268443,600.195940392519,69.014472786789));
#98358=CARTESIAN_POINT('Ctrl Pts',(11.6224782615555,600.218082360239,69.109586211324));
#98359=CARTESIAN_POINT('Ctrl Pts',(11.5400169509314,600.373465765884,68.5753485881025));
#98360=CARTESIAN_POINT('Ctrl Pts',(11.520855565674,600.110410221362,68.6277463485386));
#98361=CARTESIAN_POINT('Ctrl Pts',(11.7745701409246,600.129000209871,68.714791080186));
#98362=CARTESIAN_POINT('Ctrl Pts',(11.7970486078528,600.220248563911,67.804433162233));
#98363=CARTESIAN_POINT('Ctrl Pts',(11.7840009883711,599.961885843497,67.8485756225846));
#98364=CARTESIAN_POINT('Ctrl Pts',(12.036826018648,599.973938041764,67.9187349800865));
#98365=CARTESIAN_POINT('Ctrl Pts',(11.906165321538,600.154392365188,67.4136688048127));
#98366=CARTESIAN_POINT('Ctrl Pts',(11.8961680044815,599.897744992462,67.4527537325953));
#98367=CARTESIAN_POINT('Ctrl Pts',(12.1481605517107,599.907288835447,67.5152272280643));
#98368=CARTESIAN_POINT('Ctrl Pts',(12.0856804087928,600.045433573986,66.6213936503897));
#98369=CARTESIAN_POINT('Ctrl Pts',(12.0800305729695,599.791959022311,66.6513216880366));
#98370=CARTESIAN_POINT('Ctrl Pts',(12.3313243194805,599.79701801597,66.6971148274926));
#98371=CARTESIAN_POINT('Ctrl Pts',(12.1560806850811,600.002326913111,66.2198837351635));
#98372=CARTESIAN_POINT('Ctrl Pts',(12.1524261846195,599.749918292424,66.2443008543885));
#98373=CARTESIAN_POINT('Ctrl Pts',(12.4031554959512,599.753392286295,66.2825110894363));
#98374=CARTESIAN_POINT('Ctrl Pts',(12.257019799162,599.940372122965,65.405700320617));
#98375=CARTESIAN_POINT('Ctrl Pts',(12.2558350970482,599.689710423845,65.4202915379704));
#98376=CARTESIAN_POINT('Ctrl Pts',(12.5061462176465,599.690691466762,65.4417759684511));
#98377=CARTESIAN_POINT('Ctrl Pts',(12.2875921822733,599.921503557896,64.9916064252471));
#98378=CARTESIAN_POINT('Ctrl Pts',(12.2872829443278,599.671293324974,65.0003000739761));
#98379=CARTESIAN_POINT('Ctrl Pts',(12.5373399906064,599.671595695793,65.0141778683388));
#98380=CARTESIAN_POINT('Ctrl Pts',(12.3155824582831,599.904242740066,63.7406324714832));
#98381=CARTESIAN_POINT('Ctrl Pts',(12.3159477798069,599.654520254612,63.7345453497792));
#98382=CARTESIAN_POINT('Ctrl Pts',(12.5658991754142,599.654127032142,63.7224078328247));
#98383=CARTESIAN_POINT('Ctrl Pts',(12.2499433960128,599.945028255623,62.9203303339275));
#98384=CARTESIAN_POINT('Ctrl Pts',(12.2476351021315,599.694804185309,62.8975114326958));
#98385=CARTESIAN_POINT('Ctrl Pts',(12.4989259854136,599.695403666325,62.8753544483646));
#98386=CARTESIAN_POINT('Ctrl Pts',(12.0311680098947,600.078586517253,61.7092455282533));
#98387=CARTESIAN_POINT('Ctrl Pts',(12.02433270669,599.824074107251,61.6764817660471));
#98388=CARTESIAN_POINT('Ctrl Pts',(12.2757039450297,599.83057017083,61.6247744041512));
#98389=CARTESIAN_POINT('Ctrl Pts',(11.9376414045012,600.135444418401,61.3074767223547));
#98390=CARTESIAN_POINT('Ctrl Pts',(11.9281609256542,599.879495717932,61.269319855613));
#98391=CARTESIAN_POINT('Ctrl Pts',(12.1802763920905,599.888112726373,61.2099033326353));
#98392=CARTESIAN_POINT('Ctrl Pts',(11.710977576111,600.271739313276,60.5163094405145));
#98393=CARTESIAN_POINT('Ctrl Pts',(11.6960573690714,600.011715656205,60.4693531862596));
#98394=CARTESIAN_POINT('Ctrl Pts',(11.9490055759325,600.026048817743,60.3929349339052));
#98395=CARTESIAN_POINT('Ctrl Pts',(11.5792520747703,600.35032371235,60.1312636317803));
#98396=CARTESIAN_POINT('Ctrl Pts',(11.5607302358161,600.088147945631,60.0796799798351));
#98397=CARTESIAN_POINT('Ctrl Pts',(11.8146027265403,600.105579490779,59.9953322208473));
#98398=CARTESIAN_POINT('Ctrl Pts',(11.280933108072,600.525733694853,59.3807745414427));
#98399=CARTESIAN_POINT('Ctrl Pts',(11.2554200175323,600.257981891559,59.3216529465386));
#98400=CARTESIAN_POINT('Ctrl Pts',(11.5102203665223,600.283101674251,59.220368588735));
#98401=CARTESIAN_POINT('Ctrl Pts',(11.1143334927416,600.622567061909,59.0153358225178));
#98402=CARTESIAN_POINT('Ctrl Pts',(11.0844074462808,600.351921242835,58.9523736714234));
#98403=CARTESIAN_POINT('Ctrl Pts',(11.340234579966,600.381101060427,58.8430123811434));
#98404=CARTESIAN_POINT('Ctrl Pts',(10.7468891809611,600.832177942095,58.3032336718348));
#98405=CARTESIAN_POINT('Ctrl Pts',(10.7086606118733,600.554322751232,58.2342052329224));
#98406=CARTESIAN_POINT('Ctrl Pts',(10.9653218879177,600.593235971834,58.1076875427682));
#98407=CARTESIAN_POINT('Ctrl Pts',(10.5450918351581,600.945481422084,57.9551454984287));
#98408=CARTESIAN_POINT('Ctrl Pts',(10.5017718495429,600.663853925032,57.8832035358986));
#98409=CARTESIAN_POINT('Ctrl Pts',(10.7594229698032,600.707903795814,57.748247707264));
#98410=CARTESIAN_POINT('Ctrl Pts',(9.89450525281217,601.302185996578,56.9491928643266));
#98411=CARTESIAN_POINT('Ctrl Pts',(9.82988413289725,601.010868747812,56.8595245434182));
#98412=CARTESIAN_POINT('Ctrl Pts',(10.0956130835857,601.068903631842,56.7094894932663));
#98413=CARTESIAN_POINT('Ctrl Pts',(9.40533537943261,601.560087977633,56.3342751495656));
#98414=CARTESIAN_POINT('Ctrl Pts',(9.32615145971497,601.259629550472,56.2424874391652));
#98415=CARTESIAN_POINT('Ctrl Pts',(9.5965007327143,601.329911139954,56.0745184163995));
#98416=CARTESIAN_POINT('Ctrl Pts',(8.31786154047716,602.092338504356,55.2045355438743));
#98417=CARTESIAN_POINT('Ctrl Pts',(8.21935109391615,601.766545930577,55.1122541884108));
#98418=CARTESIAN_POINT('Ctrl Pts',(8.48692376686844,601.868570765985,54.9079363581114));
#98419=CARTESIAN_POINT('Ctrl Pts',(7.71423400494031,602.368763849128,54.687263637379));
#98420=CARTESIAN_POINT('Ctrl Pts',(7.60328278950778,602.027967838335,54.6002522073219));
#98421=CARTESIAN_POINT('Ctrl Pts',(7.87102737898878,602.148324687105,54.3737954611148));
#98422=CARTESIAN_POINT('Ctrl Pts',(6.43211894031247,602.891956348124,53.786061608348));
#98423=CARTESIAN_POINT('Ctrl Pts',(6.30828894600969,602.517777832124,53.7086110751252));
#98424=CARTESIAN_POINT('Ctrl Pts',(6.56285306515126,602.677817213243,53.4432039225965));
#98425=CARTESIAN_POINT('Ctrl Pts',(5.75022841332413,603.140946661166,53.3970489773778));
#98426=CARTESIAN_POINT('Ctrl Pts',(5.62291561811055,602.745988465143,53.3322766970217));
#98427=CARTESIAN_POINT('Ctrl Pts',(5.86710297479519,602.929805743566,53.0415050222643));
#98428=CARTESIAN_POINT('Ctrl Pts',(4.65647911755443,603.471153411197,52.9079552143514));
#98429=CARTESIAN_POINT('Ctrl Pts',(4.54890972975399,603.042807841159,52.8639499834371));
#98430=CARTESIAN_POINT('Ctrl Pts',(4.75112300194525,603.263988681109,52.5364612008833));
#98431=CARTESIAN_POINT('Ctrl Pts',(4.27753470189083,603.574456560643,52.760103963041));
#98432=CARTESIAN_POINT('Ctrl Pts',(4.17347758256706,603.135790146889,52.7219730108443));
#98433=CARTESIAN_POINT('Ctrl Pts',(4.36447646411708,603.368535755551,52.3837883044384));
#98434=CARTESIAN_POINT('Ctrl Pts',(3.5083765892915,603.757724414251,52.503472235072));
#98435=CARTESIAN_POINT('Ctrl Pts',(3.41373149403426,603.300363485533,52.4753963396111));
#98436=CARTESIAN_POINT('Ctrl Pts',(3.57968505656083,603.554010430754,52.118787442565));
#98437=CARTESIAN_POINT('Ctrl Pts',(3.11779861057926,603.837956243184,52.3942248829386));
#98438=CARTESIAN_POINT('Ctrl Pts',(3.0308328190885,603.37125022269,52.3719224428149));
#98439=CARTESIAN_POINT('Ctrl Pts',(3.18116850106493,603.635208371282,52.005977374802));
#98440=CARTESIAN_POINT('Ctrl Pts',(1.92712773112881,604.03906916062,52.1241430466814));
#98441=CARTESIAN_POINT('Ctrl Pts',(1.85276789715343,603.550990732668,52.1125876973074));
#98442=CARTESIAN_POINT('Ctrl Pts',(1.96629699390316,603.838742991852,51.7270877774893));
#98443=CARTESIAN_POINT('Ctrl Pts',(1.10486896435858,604.120172016418,52.0204162706371));
#98444=CARTESIAN_POINT('Ctrl Pts',(1.06865977295132,603.618795371852,52.0190762779579));
#98445=CARTESIAN_POINT('Ctrl Pts',(1.12732576421391,603.920822446017,51.6199783226107));
#98446=CARTESIAN_POINT('Ctrl Pts',(0.264827872760487,604.134173512545,52.0023253862613));
#98447=CARTESIAN_POINT('Ctrl Pts',(0.256610940649088,603.630932780795,52.0021484287645));
#98448=CARTESIAN_POINT('Ctrl Pts',(0.270210553101147,603.934992543017,51.6012974652903));
#98449=CARTESIAN_POINT('',(-3.86212964915782E-9,604.136374737192,76.5994959777072));
#98450=CARTESIAN_POINT('',(0.264827872760508,604.134173512545,52.0023253862613));
#98451=CARTESIAN_POINT('Ctrl Pts',(-3.25135887657702E-9,604.136374737192,
76.5994959777073));
#98452=CARTESIAN_POINT('Ctrl Pts',(0.310528165472252,604.136361525075,76.5995448311342));
#98453=CARTESIAN_POINT('Ctrl Pts',(0.618777498407439,604.127218112862,76.5878893241729));
#98454=CARTESIAN_POINT('Ctrl Pts',(0.924673649407594,604.109433246351,76.5648366833291));
#98455=CARTESIAN_POINT('Ctrl Pts',(1.23978245630647,604.09111275409,76.5410897674937));
#98456=CARTESIAN_POINT('Ctrl Pts',(1.55239421536116,604.063622646471,76.5052488949338));
#98457=CARTESIAN_POINT('Ctrl Pts',(1.8624376689848,604.027528506644,76.4576945787578));
#98458=CARTESIAN_POINT('Ctrl Pts',(1.97909517691912,604.013947660624,76.4398017061562));
#98459=CARTESIAN_POINT('Ctrl Pts',(2.09538918047889,603.999149011819,76.4202509684407));
#98460=CARTESIAN_POINT('Ctrl Pts',(2.21131621964626,603.983163694485,76.3990641890932));
#98461=CARTESIAN_POINT('Ctrl Pts',(2.28847278600611,603.972524483767,76.3849630858612));
#98462=CARTESIAN_POINT('Ctrl Pts',(2.36554368200416,603.961344248248,76.3701075120779));
#98463=CARTESIAN_POINT('Ctrl Pts',(2.44247543406213,603.949645260512,76.354512897056));
#98464=CARTESIAN_POINT('Ctrl Pts',(2.64351074550446,603.919073882892,76.3137616051136));
#98465=CARTESIAN_POINT('Ctrl Pts',(2.84402605786525,603.884881770879,76.2678728545117));
#98466=CARTESIAN_POINT('Ctrl Pts',(3.04288942631138,603.847462527482,76.2171146986224));
#98467=CARTESIAN_POINT('Ctrl Pts',(3.16477478015113,603.824527897753,76.18600451559));
#98468=CARTESIAN_POINT('Ctrl Pts',(3.28603954227911,603.800381622635,76.153065981003));
#98469=CARTESIAN_POINT('Ctrl Pts',(3.40642527297712,603.775119573837,76.1183685737292));
#98470=CARTESIAN_POINT('Ctrl Pts',(3.47943076865768,603.759799914409,76.0973270316614));
#98471=CARTESIAN_POINT('Ctrl Pts',(3.55205443377298,603.744089700583,76.0756654689925));
#98472=CARTESIAN_POINT('Ctrl Pts',(3.62429267927299,603.728007283723,76.0533936492377));
#98473=CARTESIAN_POINT('Ctrl Pts',(3.94018000276088,603.657681217773,75.9560022261365));
#98474=CARTESIAN_POINT('Ctrl Pts',(4.24915881614502,603.580147082534,75.8468009339012));
#98475=CARTESIAN_POINT('Ctrl Pts',(4.55177540581521,603.496671628223,75.7262558160285));
#98476=CARTESIAN_POINT('Ctrl Pts',(4.61866590223142,603.478220179201,75.6996104732076));
#98477=CARTESIAN_POINT('Ctrl Pts',(4.68524538832333,603.459478235103,75.6724106564061));
#98478=CARTESIAN_POINT('Ctrl Pts',(4.75151758316339,603.440457788941,75.6446572600295));
#98479=CARTESIAN_POINT('Ctrl Pts',(5.00694798018935,603.367148007569,75.5376884011832));
#98480=CARTESIAN_POINT('Ctrl Pts',(5.25788462122224,603.289684311589,75.4224616809191));
#98481=CARTESIAN_POINT('Ctrl Pts',(5.50437127899814,603.208814644317,75.2991083225829));
#98482=CARTESIAN_POINT('Ctrl Pts',(5.54958725705096,603.193979759811,75.2764801495467));
#98483=CARTESIAN_POINT('Ctrl Pts',(5.59465355084976,603.179030309245,75.2535786253423));
#98484=CARTESIAN_POINT('Ctrl Pts',(5.63957051211805,603.163970968637,75.2304047182994));
#98485=CARTESIAN_POINT('Ctrl Pts',(5.70073378556493,603.143464715732,75.1988488878676));
#98486=CARTESIAN_POINT('Ctrl Pts',(5.76165357779712,603.122739917901,75.1667619524567));
#98487=CARTESIAN_POINT('Ctrl Pts',(5.82229488838826,603.101821536855,75.1341674982548));
#98488=CARTESIAN_POINT('Ctrl Pts',(6.03771053820998,603.027513336684,75.0183824754042));
#98489=CARTESIAN_POINT('Ctrl Pts',(6.24993868384465,602.950644480758,74.8960130814168));
#98490=CARTESIAN_POINT('Ctrl Pts',(6.45731962017304,602.872343202487,74.768123123783));
#98491=CARTESIAN_POINT('Ctrl Pts',(6.5289039751283,602.845314939444,74.7239776961243));
#98492=CARTESIAN_POINT('Ctrl Pts',(6.5999109723249,602.818116157948,74.6791748810223));
#98493=CARTESIAN_POINT('Ctrl Pts',(6.67027315473924,602.790793615782,74.6337595519187));
#98494=CARTESIAN_POINT('Ctrl Pts',(6.72531600416887,602.769419768029,74.598232099019));
#98495=CARTESIAN_POINT('Ctrl Pts',(6.78000298293603,602.747961435351,74.5623194192597));
#98496=CARTESIAN_POINT('Ctrl Pts',(6.83433353593322,602.726427989239,74.526023120994));
#98497=CARTESIAN_POINT('Ctrl Pts',(7.10822454753838,602.617873648939,74.3430463371938));
#98498=CARTESIAN_POINT('Ctrl Pts',(7.37336538639597,602.507313778295,74.1501101955184));
#98499=CARTESIAN_POINT('Ctrl Pts',(7.6299541645097,602.395819428982,73.9471842046893));
#98500=CARTESIAN_POINT('Ctrl Pts',(7.88844352073621,602.283499230146,73.7427551212483));
#98501=CARTESIAN_POINT('Ctrl Pts',(8.1382537825677,602.170231334259,73.5281875575888));
#98502=CARTESIAN_POINT('Ctrl Pts',(8.37962080004122,602.057113267395,73.3034909566141));
#98503=CARTESIAN_POINT('Ctrl Pts',(8.42385440908689,602.036382927359,73.2623124157122));
#98504=CARTESIAN_POINT('Ctrl Pts',(8.46780453567475,602.015657609979,73.2207937995259));
#98505=CARTESIAN_POINT('Ctrl Pts',(8.51147274583541,601.994944051262,73.1789353160944));
#98506=CARTESIAN_POINT('Ctrl Pts',(8.55430052500405,601.974629142196,73.1378824339602));
#98507=CARTESIAN_POINT('Ctrl Pts',(8.59688191547822,601.954309987454,73.0964662008015));
#98508=CARTESIAN_POINT('Ctrl Pts',(8.63920055811426,601.934000270583,73.0547024182158));
#98509=CARTESIAN_POINT('Ctrl Pts',(8.79391013170848,601.8597514894,72.9020213161517));
#98510=CARTESIAN_POINT('Ctrl Pts',(8.94539579189053,601.785495853092,72.744405309215));
#98511=CARTESIAN_POINT('Ctrl Pts',(9.09269306746393,601.711972387154,72.582736303401));
#98512=CARTESIAN_POINT('Ctrl Pts',(9.17109278887552,601.672839149798,72.4966871557344));
#98513=CARTESIAN_POINT('Ctrl Pts',(9.24830637545171,601.633913409097,72.4094906238459));
#98514=CARTESIAN_POINT('Ctrl Pts',(9.32419224683953,601.595306269131,72.3212842918984));
#98515=CARTESIAN_POINT('Ctrl Pts',(9.36129694465004,601.576429154912,72.2781554560291));
#98516=CARTESIAN_POINT('Ctrl Pts',(9.39807441423151,601.557634424496,72.2348034790566));
#98517=CARTESIAN_POINT('Ctrl Pts',(9.43452337359977,601.538927353083,72.1912312995811));
#98518=CARTESIAN_POINT('Ctrl Pts',(9.65091478739477,601.427866579296,71.9325505119194));
#98519=CARTESIAN_POINT('Ctrl Pts',(9.85597586740214,601.319771443215,71.665812843898));
#98520=CARTESIAN_POINT('Ctrl Pts',(10.0499594594973,601.215476303349,71.3908995346974));
#98521=CARTESIAN_POINT('Ctrl Pts',(10.0810275633506,601.198772559482,71.3468698559567));
#98522=CARTESIAN_POINT('Ctrl Pts',(10.1118142187007,601.18216568156,71.3026323420182));
#98523=CARTESIAN_POINT('Ctrl Pts',(10.1423182570292,601.165659189488,71.2581851032761));
#98524=CARTESIAN_POINT('Ctrl Pts',(10.3686972363495,601.043159906367,70.9283297434156));
#98525=CARTESIAN_POINT('Ctrl Pts',(10.579559455429,600.926156659991,70.5868461102067));
#98526=CARTESIAN_POINT('Ctrl Pts',(10.7743498376453,600.81612193495,70.2330686262663));
#98527=CARTESIAN_POINT('Ctrl Pts',(10.9361257815845,600.724736665785,69.9392518281387));
#98528=CARTESIAN_POINT('Ctrl Pts',(11.0868167655327,600.638157980438,69.6369556978456));
#98529=CARTESIAN_POINT('Ctrl Pts',(11.2261259025389,600.557220983097,69.325814430765));
#98530=CARTESIAN_POINT('Ctrl Pts',(11.2465333475455,600.545364493582,69.2802352359348));
#98531=CARTESIAN_POINT('Ctrl Pts',(11.2666986076393,600.533626714025,69.2344396511952));
#98532=CARTESIAN_POINT('Ctrl Pts',(11.2866125566538,600.522014665127,69.1884489145415));
#98533=CARTESIAN_POINT('Ctrl Pts',(11.3880924823089,600.462840572735,68.9540837199202));
#98534=CARTESIAN_POINT('Ctrl Pts',(11.4831444008088,600.406895471585,68.7144140723634));
#98535=CARTESIAN_POINT('Ctrl Pts',(11.5704748159017,600.355136620185,68.4723906692956));
#98536=CARTESIAN_POINT('Ctrl Pts',(11.6043465274097,600.335061588128,68.3785202018511));
#98537=CARTESIAN_POINT('Ctrl Pts',(11.6370570637982,600.315616134507,68.2842960263233));
#98538=CARTESIAN_POINT('Ctrl Pts',(11.6685326694549,600.296855283816,68.1898912049256));
#98539=CARTESIAN_POINT('Ctrl Pts',(11.683669793509,600.287832889541,68.1444904107873));
#98540=CARTESIAN_POINT('Ctrl Pts',(11.698537234685,600.278959648324,68.0990176527924));
#98541=CARTESIAN_POINT('Ctrl Pts',(11.7131347554859,600.270236634273,68.0534740137289));
#98542=CARTESIAN_POINT('Ctrl Pts',(11.8224706417622,600.204900986847,67.7123507360731));
#98543=CARTESIAN_POINT('Ctrl Pts',(11.9167276342155,600.147980114719,67.3670528841897));
#98544=CARTESIAN_POINT('Ctrl Pts',(11.9959228357299,600.099911956208,67.0175313575219));
#98545=CARTESIAN_POINT('Ctrl Pts',(12.0059728443566,600.093812023403,66.973176468702));
#98546=CARTESIAN_POINT('Ctrl Pts',(12.0157803206307,600.087854604843,66.9287535733242));
#98547=CARTESIAN_POINT('Ctrl Pts',(12.0253444381024,600.082040781623,66.8842623710702));
#98548=CARTESIAN_POINT('Ctrl Pts',(12.0802141521759,600.048686651592,66.6290146125931));
#98549=CARTESIAN_POINT('Ctrl Pts',(12.1270883150595,600.020048631873,66.3714346350682));
#98550=CARTESIAN_POINT('Ctrl Pts',(12.1657799000495,599.996347167062,66.111637861221));
#98551=CARTESIAN_POINT('Ctrl Pts',(12.1805677414246,599.987288517692,66.0123440875899));
#98552=CARTESIAN_POINT('Ctrl Pts',(12.1941607596469,599.978950710257,65.9127266173918));
#98553=CARTESIAN_POINT('Ctrl Pts',(12.2065502013075,599.971345031511,65.8127923574291));
#98554=CARTESIAN_POINT('Ctrl Pts',(12.2119202405116,599.968048450909,65.769477177574));
#98555=CARTESIAN_POINT('Ctrl Pts',(12.2170645586533,599.964889174657,65.7260864061383));
#98556=CARTESIAN_POINT('Ctrl Pts',(12.2219815693876,599.961868387845,65.6826258242829));
#98557=CARTESIAN_POINT('Ctrl Pts',(12.2489552484082,599.945296991469,65.4442102811103));
#98558=CARTESIAN_POINT('Ctrl Pts',(12.2691246111535,599.932876901693,65.2033421763265));
#98559=CARTESIAN_POINT('Ctrl Pts',(12.28218480039,599.92482856721,64.9610218376272));
#98560=CARTESIAN_POINT('Ctrl Pts',(12.2891074986876,599.920562458166,64.8325772518866));
#98561=CARTESIAN_POINT('Ctrl Pts',(12.2940334684439,599.917524237441,64.7037249406715));
#98562=CARTESIAN_POINT('Ctrl Pts',(12.2969222724657,599.915743706266,64.5746151917459));
#98563=CARTESIAN_POINT('Ctrl Pts',(12.297866127023,599.915161956016,64.5324313592704));
#98564=CARTESIAN_POINT('Ctrl Pts',(12.2985942535798,599.914714020858,64.490284702133));
#98565=CARTESIAN_POINT('Ctrl Pts',(12.2991072457852,599.914399324768,64.4481760965921));
#98566=CARTESIAN_POINT('Ctrl Pts',(12.3039230418204,599.911445065093,64.0528748551926));
#98567=CARTESIAN_POINT('Ctrl Pts',(12.2897795816084,599.92023327766,63.6605870250526));
#98568=CARTESIAN_POINT('Ctrl Pts',(12.2571208090154,599.94032743659,63.2713649049953));
#98569=CARTESIAN_POINT('Ctrl Pts',(12.2244620364223,599.96042159552,62.8821427849379));
#98570=CARTESIAN_POINT('Ctrl Pts',(12.1732881572924,599.991821500362,62.4959863338011));
#98571=CARTESIAN_POINT('Ctrl Pts',(12.1040930127778,600.034060437411,62.1129397664499));
#98572=CARTESIAN_POINT('Ctrl Pts',(12.097501651259,600.038084016033,62.076451680159));
#98573=CARTESIAN_POINT('Ctrl Pts',(12.0907423182806,600.042208174621,62.0399811711845));
#98574=CARTESIAN_POINT('Ctrl Pts',(12.083815675173,600.046432094228,62.0035314922614));
#98575=CARTESIAN_POINT('Ctrl Pts',(12.036394081548,600.075350142405,61.7539875451004));
#98576=CARTESIAN_POINT('Ctrl Pts',(11.9810777244824,600.108982138256,61.5051624948093));
#98577=CARTESIAN_POINT('Ctrl Pts',(11.9180804827827,600.14705872784,61.2582463139844));
#98578=CARTESIAN_POINT('Ctrl Pts',(11.8885070001017,600.164933436831,61.1423337565412));
#98579=CARTESIAN_POINT('Ctrl Pts',(11.857241490088,600.18378723064,61.0268418090815));
#98580=CARTESIAN_POINT('Ctrl Pts',(11.824309419125,600.203590273384,60.9118928329591));
#98581=CARTESIAN_POINT('Ctrl Pts',(11.8147012792869,600.209367936263,60.8783557426836));
#98582=CARTESIAN_POINT('Ctrl Pts',(11.8049614391109,600.215220265117,60.8448961507762));
#98583=CARTESIAN_POINT('Ctrl Pts',(11.7950906598908,600.2211463396,60.8115140280204));
#98584=CARTESIAN_POINT('Ctrl Pts',(11.6884979670894,600.285140906071,60.4510267476747));
#98585=CARTESIAN_POINT('Ctrl Pts',(11.5665815949929,600.357772992541,60.0993881528898));
#98586=CARTESIAN_POINT('Ctrl Pts',(11.4300925444937,600.438028106791,59.7560189685528));
#98587=CARTESIAN_POINT('Ctrl Pts',(11.4183382568568,600.444939589388,59.7264483902274));
#98588=CARTESIAN_POINT('Ctrl Pts',(11.4064758513312,600.451907658307,59.6969391717302));
#98589=CARTESIAN_POINT('Ctrl Pts',(11.3945054923629,600.458931745061,59.6674910998064));
#98590=CARTESIAN_POINT('Ctrl Pts',(11.2921850121051,600.518972378091,59.4157742657605));
#98591=CARTESIAN_POINT('Ctrl Pts',(11.1819396276912,600.583126551534,59.1684441712597));
#98592=CARTESIAN_POINT('Ctrl Pts',(11.0639479787222,600.650992808033,58.9255372139082));
#98593=CARTESIAN_POINT('Ctrl Pts',(11.0205465320782,600.675956385847,58.8361875570378));
#98594=CARTESIAN_POINT('Ctrl Pts',(10.9760974098984,600.701422015914,58.7474361314692));
#98595=CARTESIAN_POINT('Ctrl Pts',(10.9306109324387,600.727369061768,58.6592839633751));
#98596=CARTESIAN_POINT('Ctrl Pts',(10.9173036742458,600.734959977966,58.6334946799086));
#98597=CARTESIAN_POINT('Ctrl Pts',(10.9039026380964,600.742594854799,58.6077492085215));
#98598=CARTESIAN_POINT('Ctrl Pts',(10.8904091198926,600.75027250686,58.5820495569516));
#98599=CARTESIAN_POINT('Ctrl Pts',(10.7698070167273,600.81889367533,58.3523517136518));
#98600=CARTESIAN_POINT('Ctrl Pts',(10.6416424932073,600.891037826986,58.1259903442765));
#98601=CARTESIAN_POINT('Ctrl Pts',(10.5068163412964,600.965864459736,57.9044450450971));
#98602=CARTESIAN_POINT('Ctrl Pts',(10.4485076621509,600.998224962937,57.808632670547));
#98603=CARTESIAN_POINT('Ctrl Pts',(10.388953607307,601.031086906189,57.713720804032));
#98604=CARTESIAN_POINT('Ctrl Pts',(10.3282293807528,601.064381304421,57.6198275512506));
#98605=CARTESIAN_POINT('Ctrl Pts',(10.3139692496735,601.072199971037,57.5977781952009));
#98606=CARTESIAN_POINT('Ctrl Pts',(10.2996497960813,601.08004000547,57.5757900176145));
#98607=CARTESIAN_POINT('Ctrl Pts',(10.2852711775002,601.087900914242,57.5538629682177));
#98608=CARTESIAN_POINT('Ctrl Pts',(10.0352430737208,601.224593330348,57.1725760906757));
#98609=CARTESIAN_POINT('Ctrl Pts',(9.7670951332938,601.367730358321,56.8094299412247));
#98610=CARTESIAN_POINT('Ctrl Pts',(9.48107593711002,601.51505087391,56.4634525360561));
#98611=CARTESIAN_POINT('Ctrl Pts',(9.28311236320542,601.617016392884,56.2239898547702));
#98612=CARTESIAN_POINT('Ctrl Pts',(9.07658839347743,601.720985696932,55.9927510172806));
#98613=CARTESIAN_POINT('Ctrl Pts',(8.86159725045973,601.826207998157,55.7694040901285));
#98614=CARTESIAN_POINT('Ctrl Pts',(8.84757081570353,601.833072903019,55.75483250798));
#98615=CARTESIAN_POINT('Ctrl Pts',(8.83350480090613,601.839944523442,55.7402928849304));
#98616=CARTESIAN_POINT('Ctrl Pts',(8.81939960411073,601.846822423391,55.7257855526291));
#98617=CARTESIAN_POINT('Ctrl Pts',(8.49324152367174,602.005861866595,55.3903287898257));
#98618=CARTESIAN_POINT('Ctrl Pts',(8.14587360451403,602.168394192616,55.071876469928));
#98619=CARTESIAN_POINT('Ctrl Pts',(7.78212530167639,602.329037592453,54.7745772655493));
#98620=CARTESIAN_POINT('Ctrl Pts',(7.55195563853653,602.430688203432,54.5864547171009));
#98621=CARTESIAN_POINT('Ctrl Pts',(7.31522835413509,602.53158201021,54.406801468053));
#98622=CARTESIAN_POINT('Ctrl Pts',(7.07317494872266,602.630354405577,54.2366615516199));
#98623=CARTESIAN_POINT('Ctrl Pts',(7.06129788050289,602.635200966095,54.2283131320183));
#98624=CARTESIAN_POINT('Ctrl Pts',(7.04940682153739,602.640043182324,54.219985871321));
#98625=CARTESIAN_POINT('Ctrl Pts',(7.03750173377691,602.644880949622,54.2116797798133));
#98626=CARTESIAN_POINT('Ctrl Pts',(6.64028634981823,602.806293921402,53.9345455499968));
#98627=CARTESIAN_POINT('Ctrl Pts',(6.22730832302605,602.962823386694,53.6808812320354));
#98628=CARTESIAN_POINT('Ctrl Pts',(5.79712163891057,603.110586537824,53.451089758777));
#98629=CARTESIAN_POINT('Ctrl Pts',(5.54446643552948,603.197370091056,53.3161297203678));
#98630=CARTESIAN_POINT('Ctrl Pts',(5.28587575785619,603.281129805348,53.1894035722773));
#98631=CARTESIAN_POINT('Ctrl Pts',(5.02106131531314,603.361080841205,53.0709860658359));
#98632=CARTESIAN_POINT('Ctrl Pts',(5.01259930724037,603.363635635061,53.0672020958763));
#98633=CARTESIAN_POINT('Ctrl Pts',(5.00412957485699,603.366186781108,53.0634263089924));
#98634=CARTESIAN_POINT('Ctrl Pts',(4.99565222801652,603.36873421786,53.0596587598676));
#98635=CARTESIAN_POINT('Ctrl Pts',(4.72092237011719,603.451290346567,52.9375618048699));
#98636=CARTESIAN_POINT('Ctrl Pts',(4.43801237496684,603.530001065124,52.8240393805438));
#98637=CARTESIAN_POINT('Ctrl Pts',(4.15077506050142,603.602727805415,52.7210258524162));
#98638=CARTESIAN_POINT('Ctrl Pts',(4.06518506620748,603.624398671187,52.6903302330081));
#98639=CARTESIAN_POINT('Ctrl Pts',(3.9792111112585,603.645538308539,52.6605674732759));
#98640=CARTESIAN_POINT('Ctrl Pts',(3.89295563852526,603.666090453821,52.631788096699));
#98641=CARTESIAN_POINT('Ctrl Pts',(3.88647932075825,603.667633570094,52.6296272553988));
#98642=CARTESIAN_POINT('Ctrl Pts',(3.88000131269559,603.66917345026,52.6274718253079));
#98643=CARTESIAN_POINT('Ctrl Pts',(3.87352161455216,603.670710085412,52.6253218076544));
#98644=CARTESIAN_POINT('Ctrl Pts',(3.49528738953934,603.760406857197,52.4998205508172));
#98645=CARTESIAN_POINT('Ctrl Pts',(3.11117130680275,603.839071965887,52.3927215905075));
#98646=CARTESIAN_POINT('Ctrl Pts',(2.72090801980655,603.904991991953,52.3041975366685));
#98647=CARTESIAN_POINT('Ctrl Pts',(2.71660777482109,603.905718353543,52.3032221051296));
#98648=CARTESIAN_POINT('Ctrl Pts',(2.71230668873312,603.906443162019,52.3022489124891));
#98649=CARTESIAN_POINT('Ctrl Pts',(2.70800476328749,603.907166415128,52.3012779602549));
#98650=CARTESIAN_POINT('Ctrl Pts',(2.51064590304966,603.9403470016,52.2567337140315));
#98651=CARTESIAN_POINT('Ctrl Pts',(2.31170028173491,603.970224507093,52.2169417014671));
#98652=CARTESIAN_POINT('Ctrl Pts',(2.11111770838935,603.996621239467,52.1819925296957));
#98653=CARTESIAN_POINT('Ctrl Pts',(1.91053513504379,604.023017971842,52.1470433579242));
#98654=CARTESIAN_POINT('Ctrl Pts',(1.70831537286292,604.045934249502,52.116936815071));
#98655=CARTESIAN_POINT('Ctrl Pts',(1.50439479076097,604.0651612546,52.0918063490636));
#98656=CARTESIAN_POINT('Ctrl Pts',(1.36067001764632,604.07871259364,52.0740942059933));
#98657=CARTESIAN_POINT('Ctrl Pts',(1.21594950307107,604.09044149521,52.0588407343315));
#98658=CARTESIAN_POINT('Ctrl Pts',(1.07058065254979,604.10023689204,52.0461417320882));
#98659=CARTESIAN_POINT('Ctrl Pts',(0.927490453078763,604.109878746408,52.0336417862087));
#98660=CARTESIAN_POINT('Ctrl Pts',(0.783772258610783,604.117647119529,52.0236168794799));
#98661=CARTESIAN_POINT('Ctrl Pts',(0.639767420115063,604.12346573865,52.0161192211438));
#98662=CARTESIAN_POINT('Ctrl Pts',(0.514927066399052,604.128510002973,52.0096193678855));
#98663=CARTESIAN_POINT('Ctrl Pts',(0.389871499267707,604.132089331343,52.0050182899915));
#98664=CARTESIAN_POINT('Ctrl Pts',(0.264827872760508,604.134173512545,52.0023253862613));
#98665=CARTESIAN_POINT('',(0.270210553101167,603.934992543017,51.6012974652903));
#98666=CARTESIAN_POINT('Origin',(0.270210553101161,604.134173512545,51.7523833394738));
#98667=CARTESIAN_POINT('',(-0.252645464510396,603.935273498433,76.9980210944396));
#98668=CARTESIAN_POINT('Ctrl Pts',(0.270210553101167,603.934992543017,51.6012974652903));
#98669=CARTESIAN_POINT('Ctrl Pts',(0.416188845712395,603.932579184183,51.6044790675076));
#98670=CARTESIAN_POINT('Ctrl Pts',(0.562179672062878,603.928184368032,51.6102408737133));
#98671=CARTESIAN_POINT('Ctrl Pts',(0.707836668903442,603.921856159795,51.6185654510171));
#98672=CARTESIAN_POINT('Ctrl Pts',(0.855734314323341,603.915430604426,51.6270180856934));
#98673=CARTESIAN_POINT('Ctrl Pts',(1.00328760572363,603.907011809844,51.6381129450356));
#98674=CARTESIAN_POINT('Ctrl Pts',(1.15014230608927,603.896682910039,51.651789297983));
#98675=CARTESIAN_POINT('Ctrl Pts',(1.28385901362533,603.887278059729,51.6642421298138));
#98676=CARTESIAN_POINT('Ctrl Pts',(1.41699655037471,603.876290085905,51.678834639128));
#98677=CARTESIAN_POINT('Ctrl Pts',(1.54929519817638,603.863803587702,51.6954914009046));
#98678=CARTESIAN_POINT('Ctrl Pts',(1.75719362309163,603.844181895777,51.7216663814889));
#98679=CARTESIAN_POINT('Ctrl Pts',(1.96334804814265,603.82083589846,51.7529703760962));
#98680=CARTESIAN_POINT('Ctrl Pts',(2.16781670603911,603.793978432753,51.7892635905837));
#98681=CARTESIAN_POINT('Ctrl Pts',(2.37228536393557,603.767120967045,51.8255568050712));
#98682=CARTESIAN_POINT('Ctrl Pts',(2.57506848853287,603.736751721069,51.8668394514028));
#98683=CARTESIAN_POINT('Ctrl Pts',(2.77621117828721,603.703052922097,51.913014617884));
#98684=CARTESIAN_POINT('Ctrl Pts',(2.78094727797299,603.702259451197,51.9141018569566));
#98685=CARTESIAN_POINT('Ctrl Pts',(2.78568258013029,603.701464139836,51.9151918299073));
#98686=CARTESIAN_POINT('Ctrl Pts',(2.79041708794954,603.700666990254,51.9162845374166));
#98687=CARTESIAN_POINT('Ctrl Pts',(3.19062783311622,603.633283464828,52.0086517492297));
#98688=CARTESIAN_POINT('Ctrl Pts',(3.58441626783843,603.552886400077,52.120393363137));
#98689=CARTESIAN_POINT('Ctrl Pts',(3.97207884850313,603.461270401369,52.2512917195333));
#98690=CARTESIAN_POINT('Ctrl Pts',(3.97854352352209,603.459742609708,52.2534745851923));
#98691=CARTESIAN_POINT('Ctrl Pts',(3.98500659612942,603.458211624714,52.2556629087787));
#98692=CARTESIAN_POINT('Ctrl Pts',(3.99146802647606,603.456677468783,52.2578566698448));
#98693=CARTESIAN_POINT('Ctrl Pts',(4.32723754948626,603.376954748337,52.3718559033388));
#98694=CARTESIAN_POINT('Ctrl Pts',(4.65860664857762,603.288651568303,52.5005649822081));
#98695=CARTESIAN_POINT('Ctrl Pts',(4.97989942382872,603.194923456042,52.6410924029741));
#98696=CARTESIAN_POINT('Ctrl Pts',(5.02786800045472,603.180929975698,52.6620729567566));
#98697=CARTESIAN_POINT('Ctrl Pts',(5.0756120622286,603.166815578228,52.6833169044434));
#98698=CARTESIAN_POINT('Ctrl Pts',(5.12311282356784,603.15259076398,52.7048145891233));
#98699=CARTESIAN_POINT('Ctrl Pts',(5.13072165517588,603.150312185422,52.708258160512));
#98700=CARTESIAN_POINT('Ctrl Pts',(5.1383253293963,603.148030584285,52.7117084833211));
#98701=CARTESIAN_POINT('Ctrl Pts',(5.14592385222659,603.145745978856,52.7151655548058));
#98702=CARTESIAN_POINT('Ctrl Pts',(5.65405453740944,602.992969163174,52.9463478703011));
#98703=CARTESIAN_POINT('Ctrl Pts',(6.13932327105491,602.826720053408,53.2077731233885));
#98704=CARTESIAN_POINT('Ctrl Pts',(6.60384272748034,602.652322803614,53.4988133236704));
#98705=CARTESIAN_POINT('Ctrl Pts',(6.81232117442907,602.574052523895,53.6294334906302));
#98706=CARTESIAN_POINT('Ctrl Pts',(7.01662033266161,602.494140574613,53.7660183722793));
#98707=CARTESIAN_POINT('Ctrl Pts',(7.21693171141822,602.413065746167,53.9085088387218));
#98708=CARTESIAN_POINT('Ctrl Pts',(7.22513947055266,602.409743704913,53.9143473858616));
#98709=CARTESIAN_POINT('Ctrl Pts',(7.2333410811538,602.40641935671,53.9201966743798));
#98710=CARTESIAN_POINT('Ctrl Pts',(7.24153649808195,602.403092752226,53.92605666394));
#98711=CARTESIAN_POINT('Ctrl Pts',(7.6043313178296,602.255830583023,54.1854667555637));
#98712=CARTESIAN_POINT('Ctrl Pts',(7.95512168434254,602.104087311807,54.4659556720524));
#98713=CARTESIAN_POINT('Ctrl Pts',(8.28995998189607,601.952249122013,54.7640522820103));
#98714=CARTESIAN_POINT('Ctrl Pts',(8.55084003074742,601.833948573179,54.996306055657));
#98715=CARTESIAN_POINT('Ctrl Pts',(8.80203719276935,601.715590317356,55.23924784128));
#98716=CARTESIAN_POINT('Ctrl Pts',(9.04170368382727,601.599237814998,55.4912341838177));
#98717=CARTESIAN_POINT('Ctrl Pts',(9.04882604992429,601.595780072055,55.4987226690669));
#98718=CARTESIAN_POINT('Ctrl Pts',(9.05593912941172,601.592323753148,55.5062195590408));
#98719=CARTESIAN_POINT('Ctrl Pts',(9.06304292057171,601.588868883909,55.51372486464));
#98720=CARTESIAN_POINT('Ctrl Pts',(9.41782794432331,601.416322163805,55.8885627456103));
#98721=CARTESIAN_POINT('Ctrl Pts',(9.74946630680735,601.247393456694,56.2843874741021));
#98722=CARTESIAN_POINT('Ctrl Pts',(10.0578808158284,601.085182977549,56.7027531625713));
#98723=CARTESIAN_POINT('Ctrl Pts',(10.2247778709415,600.997403542776,56.9291497792141));
#98724=CARTESIAN_POINT('Ctrl Pts',(10.3848733586417,600.911591214942,57.1621477031375));
#98725=CARTESIAN_POINT('Ctrl Pts',(10.5381498361278,600.828236438483,57.4019967994255));
#98726=CARTESIAN_POINT('Ctrl Pts',(10.5430825010644,600.825553957845,57.4097154999511));
#98727=CARTESIAN_POINT('Ctrl Pts',(10.5480074933753,600.822874310698,57.4174407015241));
#98728=CARTESIAN_POINT('Ctrl Pts',(10.5529247796569,600.820197529248,57.4251723494432));
#98729=CARTESIAN_POINT('Ctrl Pts',(10.7311538823448,600.723176463412,57.7054091695081));
#98730=CARTESIAN_POINT('Ctrl Pts',(10.8991800315513,600.629963227712,57.9939850694789));
#98731=CARTESIAN_POINT('Ctrl Pts',(11.0554949410961,600.542048163169,58.2883985366065));
#98732=CARTESIAN_POINT('Ctrl Pts',(11.0884477683713,600.523514742747,58.3504639925379));
#98733=CARTESIAN_POINT('Ctrl Pts',(11.1208800201954,600.505216810882,58.412789017351));
#98734=CARTESIAN_POINT('Ctrl Pts',(11.1527773651985,600.487168396746,58.4753503757855));
#98735=CARTESIAN_POINT('Ctrl Pts',(11.1563744083562,600.485133088649,58.4824053800899));
#98736=CARTESIAN_POINT('Ctrl Pts',(11.1599650069621,600.483100757688,58.4894639315986));
#98737=CARTESIAN_POINT('Ctrl Pts',(11.1635491598044,600.481071411546,58.4965260351482));
#98738=CARTESIAN_POINT('Ctrl Pts',(11.3468191789593,600.377303987905,58.8576355943088));
#98739=CARTESIAN_POINT('Ctrl Pts',(11.5131975113051,600.281365293344,59.2279486399778));
#98740=CARTESIAN_POINT('Ctrl Pts',(11.6624107054815,600.194340509752,59.6078507224401));
#98741=CARTESIAN_POINT('Ctrl Pts',(11.6647417380394,600.192980994563,59.613785613975));
#98742=CARTESIAN_POINT('Ctrl Pts',(11.6670685829227,600.191623652892,59.6197228445413));
#98743=CARTESIAN_POINT('Ctrl Pts',(11.6693912367388,600.19026848945,59.6256624167821));
#98744=CARTESIAN_POINT('Ctrl Pts',(11.7914614847136,600.119046021278,59.9378247593849));
#98745=CARTESIAN_POINT('Ctrl Pts',(11.9019377577438,600.053852316669,60.2563928913557));
#98746=CARTESIAN_POINT('Ctrl Pts',(12.0003794520661,599.995341549017,60.5818958373324));
#98747=CARTESIAN_POINT('Ctrl Pts',(12.022403961461,599.982250846336,60.6547211045231));
#98748=CARTESIAN_POINT('Ctrl Pts',(12.0438259072257,599.969494746759,60.7278935918928));
#98749=CARTESIAN_POINT('Ctrl Pts',(12.0646400666275,599.957080728915,60.80141938881));
#98750=CARTESIAN_POINT('Ctrl Pts',(12.0658734024639,599.956345140569,60.8057761345467));
#98751=CARTESIAN_POINT('Ctrl Pts',(12.0671044404052,599.955610851485,60.8101336095226));
#98752=CARTESIAN_POINT('Ctrl Pts',(12.0683331795544,599.954877862898,60.8144918087508));
#98753=CARTESIAN_POINT('Ctrl Pts',(12.1541174147216,599.903704377145,61.1187588191434));
#98754=CARTESIAN_POINT('Ctrl Pts',(12.2286492071889,599.858897740509,61.4263757001235));
#98755=CARTESIAN_POINT('Ctrl Pts',(12.2916497337276,599.820862373119,61.7356739632439));
#98756=CARTESIAN_POINT('Ctrl Pts',(12.3123901833266,599.808340721893,61.8374982715437));
#98757=CARTESIAN_POINT('Ctrl Pts',(12.3318805284037,599.796553133965,61.9395049355604));
#98758=CARTESIAN_POINT('Ctrl Pts',(12.3501097718202,599.785514639999,62.0416346902988));
#98759=CARTESIAN_POINT('Ctrl Pts',(12.3505132822593,599.785270299219,62.0438953667977));
#98760=CARTESIAN_POINT('Ctrl Pts',(12.3509161912353,599.785026317299,62.0461561431484));
#98761=CARTESIAN_POINT('Ctrl Pts',(12.3513184986724,599.784782694315,62.048417019426));
#98762=CARTESIAN_POINT('Ctrl Pts',(12.4988878701167,599.695419964955,62.8777233171341));
#98763=CARTESIAN_POINT('Ctrl Pts',(12.5654436335101,599.654404252705,63.719998294979));
#98764=CARTESIAN_POINT('Ctrl Pts',(12.547023784357,599.665671383483,64.5759864683422));
#98765=CARTESIAN_POINT('Ctrl Pts',(12.5469692630458,599.665704733307,64.5785201263098));
#98766=CARTESIAN_POINT('Ctrl Pts',(12.5469139970635,599.665738541241,64.5810539094377));
#98767=CARTESIAN_POINT('Ctrl Pts',(12.5468579862992,599.665772807391,64.5835878177418));
#98768=CARTESIAN_POINT('Ctrl Pts',(12.5374524690111,599.67152689537,65.0090902838063));
#98769=CARTESIAN_POINT('Ctrl Pts',(12.5068775203495,599.690243814354,65.4317526596763));
#98770=CARTESIAN_POINT('Ctrl Pts',(12.4564407748525,599.720951539445,65.8474537330173));
#98771=CARTESIAN_POINT('Ctrl Pts',(12.4558465628446,599.721313317328,65.8523512450805));
#98772=CARTESIAN_POINT('Ctrl Pts',(12.4552495926927,599.721676760513,65.8572478053186));
#98773=CARTESIAN_POINT('Ctrl Pts',(12.4546498665094,599.722041867425,65.8621434068506));
#98774=CARTESIAN_POINT('Ctrl Pts',(12.4040416607679,599.752851604014,66.2752612870232));
#98775=CARTESIAN_POINT('Ctrl Pts',(12.3337717584624,599.795530575477,66.6829679693347));
#98776=CARTESIAN_POINT('Ctrl Pts',(12.2443814590765,599.849359697038,67.0853656096814));
#98777=CARTESIAN_POINT('Ctrl Pts',(12.2428405235091,599.850287618843,67.0923022553853));
#98778=CARTESIAN_POINT('Ctrl Pts',(12.2412939039662,599.851218854629,67.0992373326653));
#98779=CARTESIAN_POINT('Ctrl Pts',(12.2397416031979,599.852153400742,67.1061708425376));
#98780=CARTESIAN_POINT('Ctrl Pts',(12.150177183183,599.90607470408,67.5062194691017));
#98781=CARTESIAN_POINT('Ctrl Pts',(12.0416978792334,599.971020248024,67.9010490570525));
#98782=CARTESIAN_POINT('Ctrl Pts',(11.914246482633,600.046412925267,68.2907180385381));
#98783=CARTESIAN_POINT('Ctrl Pts',(11.9114061210395,600.048093114505,68.2994021396051));
#98784=CARTESIAN_POINT('Ctrl Pts',(11.9085563276577,600.049778496453,68.3080836988315));
#98785=CARTESIAN_POINT('Ctrl Pts',(11.9056971018176,600.051469064628,68.3167627159898));
#98786=CARTESIAN_POINT('Ctrl Pts',(11.7780348473212,600.12695164511,68.7042742170754));
#98787=CARTESIAN_POINT('Ctrl Pts',(11.63045559295,600.213409708628,69.0888496165626));
#98788=CARTESIAN_POINT('Ctrl Pts',(11.4674585767456,600.30739636449,69.4598550915683));
#98789=CARTESIAN_POINT('Ctrl Pts',(11.4630803893133,600.309920896565,69.4698204979655));
#98790=CARTESIAN_POINT('Ctrl Pts',(11.458691033693,600.312450893269,69.4797762480409));
#98791=CARTESIAN_POINT('Ctrl Pts',(11.4542905965529,600.314986288131,69.4897221352274));
#98792=CARTESIAN_POINT('Ctrl Pts',(11.2649214349098,600.424094902628,69.9177351390182));
#98793=CARTESIAN_POINT('Ctrl Pts',(11.0548558466121,600.543398885326,70.3297521124981));
#98794=CARTESIAN_POINT('Ctrl Pts',(10.8247037222242,600.670946153262,70.726699225892));
#98795=CARTESIAN_POINT('Ctrl Pts',(10.6530709448023,600.766062771919,71.0227170694926));
#98796=CARTESIAN_POINT('Ctrl Pts',(10.4702683526939,600.86576296356,71.3103549097454));
#98797=CARTESIAN_POINT('Ctrl Pts',(10.2765612833766,600.969227847842,71.5900073533418));
#98798=CARTESIAN_POINT('Ctrl Pts',(10.26913038327,600.973196919402,71.6007352497487));
#98799=CARTESIAN_POINT('Ctrl Pts',(10.2616833989456,600.97717153958,71.6114514209664));
#98800=CARTESIAN_POINT('Ctrl Pts',(10.2542203448061,600.981151662732,71.6221558912206));
#98801=CARTESIAN_POINT('Ctrl Pts',(10.0309413485718,601.100228636524,71.9424112891989));
#98802=CARTESIAN_POINT('Ctrl Pts',(9.79314227964304,601.224262012816,72.252096789745));
#98803=CARTESIAN_POINT('Ctrl Pts',(9.54042013959494,601.352059769454,72.5513581119672));
#98804=CARTESIAN_POINT('Ctrl Pts',(9.53153439293212,601.356553156893,72.561880182945));
#98805=CARTESIAN_POINT('Ctrl Pts',(9.52263008694161,601.36105124802,72.5723894853929));
#98806=CARTESIAN_POINT('Ctrl Pts',(9.51370721162863,601.365553986183,72.5828860130588));
#98807=CARTESIAN_POINT('Ctrl Pts',(9.31151806381215,601.467584414717,72.8207335576388));
#98808=CARTESIAN_POINT('Ctrl Pts',(9.10007725190372,601.571822437062,73.0514824786637));
#98809=CARTESIAN_POINT('Ctrl Pts',(8.88162082266105,601.676422980297,73.27297063567));
#98810=CARTESIAN_POINT('Ctrl Pts',(8.82635703934914,601.702884191695,73.3290013670949));
#98811=CARTESIAN_POINT('Ctrl Pts',(8.77064449620276,601.729368546238,73.3844395960069));
#98812=CARTESIAN_POINT('Ctrl Pts',(8.71451977111148,601.7558461,73.4392506659581));
#98813=CARTESIAN_POINT('Ctrl Pts',(8.70451527424168,601.760565848797,73.4490209976055));
#98814=CARTESIAN_POINT('Ctrl Pts',(8.69449736220669,601.765285535632,73.4587717209558));
#98815=CARTESIAN_POINT('Ctrl Pts',(8.68446623164617,601.770004995063,73.4685026450421));
#98816=CARTESIAN_POINT('Ctrl Pts',(8.35856609473877,601.923334917907,73.784649411633));
#98817=CARTESIAN_POINT('Ctrl Pts',(8.0173051312327,602.077302264897,74.0819867967456));
#98818=CARTESIAN_POINT('Ctrl Pts',(7.65987184783966,602.229304213188,74.3606572775429));
#98819=CARTESIAN_POINT('Ctrl Pts',(7.39538696002535,602.341778960531,74.566861160268));
#98820=CARTESIAN_POINT('Ctrl Pts',(7.12204759188462,602.453176967428,74.7628452062661));
#98821=CARTESIAN_POINT('Ctrl Pts',(6.83953361923856,602.562438676942,74.9486824712655));
#98822=CARTESIAN_POINT('Ctrl Pts',(6.8283183754523,602.566776149872,74.9560598417085));
#98823=CARTESIAN_POINT('Ctrl Pts',(6.81708850557562,602.571110306088,74.963421308603));
#98824=CARTESIAN_POINT('Ctrl Pts',(6.80584399584163,602.575441076129,74.9707668709572));
#98825=CARTESIAN_POINT('Ctrl Pts',(6.53600531050979,602.679368176726,75.1470410648162));
#98826=CARTESIAN_POINT('Ctrl Pts',(6.25682003402361,602.781549749761,75.3144018558047));
#98827=CARTESIAN_POINT('Ctrl Pts',(5.97168962523098,602.879560274357,75.4705491677736));
#98828=CARTESIAN_POINT('Ctrl Pts',(5.91058146394901,602.900565550398,75.5040141186497));
#98829=CARTESIAN_POINT('Ctrl Pts',(5.84920038486591,602.921379256117,75.5369641331808));
#98830=CARTESIAN_POINT('Ctrl Pts',(5.78758008341291,602.94197756147,75.5693767842874));
#98831=CARTESIAN_POINT('Ctrl Pts',(5.77645936187983,602.94569497298,75.5752263510472));
#98832=CARTESIAN_POINT('Ctrl Pts',(5.76533057667263,602.949405471281,75.5810585770746));
#98833=CARTESIAN_POINT('Ctrl Pts',(5.75419392195764,602.953108915887,75.5868733289663));
#98834=CARTESIAN_POINT('Ctrl Pts',(5.43563539121675,603.059044127368,75.7532014469371));
#98835=CARTESIAN_POINT('Ctrl Pts',(5.10974723271856,603.159597121675,75.9059290152303));
#98836=CARTESIAN_POINT('Ctrl Pts',(4.77620299473305,603.25324969582,76.0448419303691));
#98837=CARTESIAN_POINT('Ctrl Pts',(4.74275640446179,603.262640831743,76.0587716069364));
#98838=CARTESIAN_POINT('Ctrl Pts',(4.70923285127606,603.271962590153,76.0725624092105));
#98839=CARTESIAN_POINT('Ctrl Pts',(4.67563202082693,603.281213446915,76.0862141459992));
#98840=CARTESIAN_POINT('Ctrl Pts',(4.66519251392581,603.284087613468,76.0904556304658));
#98841=CARTESIAN_POINT('Ctrl Pts',(4.65474549323412,603.286954951213,76.0946837135968));
#98842=CARTESIAN_POINT('Ctrl Pts',(4.64429094472362,603.28981541585,76.0988983916672));
#98843=CARTESIAN_POINT('Ctrl Pts',(4.27379986217436,603.391185325689,76.248259278874));
#98844=CARTESIAN_POINT('Ctrl Pts',(3.89386018446255,603.483930593988,76.3807926409729));
#98845=CARTESIAN_POINT('Ctrl Pts',(3.50348924748349,603.565802211847,76.4956462456033));
#98846=CARTESIAN_POINT('Ctrl Pts',(3.49421925398875,603.567746386715,76.4983736314481));
#98847=CARTESIAN_POINT('Ctrl Pts',(3.48494331671118,603.569684439582,76.5010910617607));
#98848=CARTESIAN_POINT('Ctrl Pts',(3.47566142285345,603.571616339724,76.5037985243144));
#98849=CARTESIAN_POINT('Ctrl Pts',(3.11357967530811,603.646978737772,76.6094151999532));
#98850=CARTESIAN_POINT('Ctrl Pts',(2.7438424302204,603.712508108099,76.6992121831753));
#98851=CARTESIAN_POINT('Ctrl Pts',(2.37198166188092,603.765955496843,76.7716691688606));
#98852=CARTESIAN_POINT('Ctrl Pts',(2.34061880025861,603.770463267493,76.7777802152766));
#98853=CARTESIAN_POINT('Ctrl Pts',(2.30924086295087,603.774885088492,76.7837679159742));
#98854=CARTESIAN_POINT('Ctrl Pts',(2.27785118480887,603.779219606907,76.7896313582786));
#98855=CARTESIAN_POINT('Ctrl Pts',(2.27065610270344,603.780213156944,76.7909753653311));
#98856=CARTESIAN_POINT('Ctrl Pts',(2.26346025582309,603.781202142936,76.7923128747317));
#98857=CARTESIAN_POINT('Ctrl Pts',(2.2562636865822,603.7821865477,76.7936438742462));
#98858=CARTESIAN_POINT('Ctrl Pts',(1.9692581637581,603.821445477121,76.8467253077395));
#98859=CARTESIAN_POINT('Ctrl Pts',(1.68006019104971,603.853622624926,76.8898579427872));
#98860=CARTESIAN_POINT('Ctrl Pts',(1.38876410941509,603.878279106643,76.9227278834569));
#98861=CARTESIAN_POINT('Ctrl Pts',(1.10512361179407,603.902287588681,76.9547339656398));
#98862=CARTESIAN_POINT('Ctrl Pts',(0.819493826352742,603.919165365058,76.9770097040741));
#98863=CARTESIAN_POINT('Ctrl Pts',(0.531969592127929,603.928534477404,76.9893049833241));
#98864=CARTESIAN_POINT('Ctrl Pts',(0.271955131239933,603.937007170853,77.0004238735779));
#98865=CARTESIAN_POINT('Ctrl Pts',(0.0103914694479063,603.939339493112,
77.0033811689881));
#98866=CARTESIAN_POINT('Ctrl Pts',(-0.252645464510395,603.935273498433,
76.9980210944396));
#98867=CARTESIAN_POINT('',(-0.247612686332903,604.134451125088,76.5969814761947));
#98868=CARTESIAN_POINT('Origin',(-0.252645464510396,604.134451125088,76.8469308133488));
#98869=CARTESIAN_POINT('Origin',(0.00102225664455322,598.119834463972,68.9078455093001));
#98870=CARTESIAN_POINT('Origin',(0.,1218.57245358804,64.2994740882088));
#98871=CARTESIAN_POINT('',(5.49793566439933E-15,605.608439769695,76.5994740882088));
#98872=CARTESIAN_POINT('',(1.50631556295125E-15,605.608439769695,51.9994740882088));
#98873=CARTESIAN_POINT('Ctrl Pts',(-5.41233724504764E-15,605.608439769695,
76.5994740882088));
#98874=CARTESIAN_POINT('Ctrl Pts',(0.803517342471626,605.608439769695,76.5994740882088));
#98875=CARTESIAN_POINT('Ctrl Pts',(1.62216512710203,605.542186255804,76.5196085118227));
#98876=CARTESIAN_POINT('Ctrl Pts',(3.23077935439455,605.286420618322,76.195909276783));
#98877=CARTESIAN_POINT('Ctrl Pts',(4.02089381669516,605.097608851242,75.952258243854));
#98878=CARTESIAN_POINT('Ctrl Pts',(6.27564182199435,604.41675711289,75.0030400468755));
#98879=CARTESIAN_POINT('Ctrl Pts',(7.62604171070065,603.813936675359,74.0682591946972));
#98880=CARTESIAN_POINT('Ctrl Pts',(9.75980156458901,602.747193352477,71.9344993408089));
#98881=CARTESIAN_POINT('Ctrl Pts',(10.7006947361121,602.202165792572,70.5818572288996));
#98882=CARTESIAN_POINT('Ctrl Pts',(11.654095320228,601.628958177762,68.317292844778));
#98883=CARTESIAN_POINT('Ctrl Pts',(11.8983125166469,601.477289438537,67.5235508793709));
#98884=CARTESIAN_POINT('Ctrl Pts',(12.2213288811781,601.275438695951,65.9130515674887));
#98885=CARTESIAN_POINT('Ctrl Pts',(12.3,601.225373764374,65.0962538701053));
#98886=CARTESIAN_POINT('Ctrl Pts',(12.3,601.225373764374,63.5026943063123));
#98887=CARTESIAN_POINT('Ctrl Pts',(12.2213288811781,601.275438695951,62.6858966089289));
#98888=CARTESIAN_POINT('Ctrl Pts',(11.8983125166469,601.477289438537,61.0753972970467));
#98889=CARTESIAN_POINT('Ctrl Pts',(11.654095320228,601.628958177762,60.2816553316396));
#98890=CARTESIAN_POINT('Ctrl Pts',(10.7006947361121,602.202165792572,58.017090947518));
#98891=CARTESIAN_POINT('Ctrl Pts',(9.75980156458901,602.747193352477,56.6644488356087));
#98892=CARTESIAN_POINT('Ctrl Pts',(7.62604171070065,603.813936675359,54.5306889817204));
#98893=CARTESIAN_POINT('Ctrl Pts',(6.27564182199435,604.41675711289,53.5959081295421));
#98894=CARTESIAN_POINT('Ctrl Pts',(4.02089381669516,605.097608851242,52.6466899325635));
#98895=CARTESIAN_POINT('Ctrl Pts',(3.23077935439454,605.286420618322,52.4030388996346));
#98896=CARTESIAN_POINT('Ctrl Pts',(1.62216512710202,605.542186255804,52.0793396645949));
#98897=CARTESIAN_POINT('Ctrl Pts',(0.803517342471629,605.608439769695,51.9994740882088));
#98898=CARTESIAN_POINT('Ctrl Pts',(-1.66533453693773E-15,605.608439769695,
51.9994740882088));
#98899=CARTESIAN_POINT('',(2.22564887778133E-9,604.13637726519,51.9994620213434));
#98900=CARTESIAN_POINT('',(1.50631556295125E-15,1218.57245358804,51.9994740882088));
#98901=CARTESIAN_POINT('Origin',(-0.00103899058863242,598.122522219325,
59.6908665380107));
#98902=CARTESIAN_POINT('Ctrl Pts',(-1.17513814323332E-13,604.136380686556,
51.9994740882088));
#98903=CARTESIAN_POINT('Ctrl Pts',(-0.830412355315779,604.136380686556,
51.9994740882088));
#98904=CARTESIAN_POINT('Ctrl Pts',(-1.64231938507752,604.071082960544,52.0826407378975));
#98905=CARTESIAN_POINT('Ctrl Pts',(-2.83515367981027,603.890097069807,52.323812890186));
#98906=CARTESIAN_POINT('Ctrl Pts',(-3.22987045740506,603.81567035152,52.424181909713));
#98907=CARTESIAN_POINT('Ctrl Pts',(-4.00546366491676,603.643294902985,52.6628556650889));
#98908=CARTESIAN_POINT('Ctrl Pts',(-4.38197303754884,603.546457604273,52.7996457417166));
#98909=CARTESIAN_POINT('Ctrl Pts',(-5.11472586370269,603.336277713785,53.1062922778494));
#98910=CARTESIAN_POINT('Ctrl Pts',(-5.47096314710355,603.222927458667,53.2761570602037));
#98911=CARTESIAN_POINT('Ctrl Pts',(-6.16461781176576,602.983839522965,53.6485378245871));
#98912=CARTESIAN_POINT('Ctrl Pts',(-6.50301550231245,602.857701739012,53.851722530015));
#98913=CARTESIAN_POINT('Ctrl Pts',(-7.48440400049397,602.468880926984,54.5069979081194));
#98914=CARTESIAN_POINT('Ctrl Pts',(-8.08540127789581,602.199757460366,54.9978561404269));
#98915=CARTESIAN_POINT('Ctrl Pts',(-8.91512989826463,601.801595070901,55.8164668699611));
#98916=CARTESIAN_POINT('Ctrl Pts',(-9.17960981988056,601.669736473115,56.1031778705516));
#98917=CARTESIAN_POINT('Ctrl Pts',(-9.68420831858871,601.410800771055,56.7060152337074));
#98918=CARTESIAN_POINT('Ctrl Pts',(-9.92291043224852,601.284425051111,57.020747596285));
#98919=CARTESIAN_POINT('Ctrl Pts',(-10.5886307482388,600.924068655943,57.9917849677706));
#98920=CARTESIAN_POINT('Ctrl Pts',(-10.9702548417479,600.706496345919,58.6797638067076));
#98921=CARTESIAN_POINT('Ctrl Pts',(-11.4461458407884,600.429020734492,59.778948219836));
#98922=CARTESIAN_POINT('Ctrl Pts',(-11.5888532985442,600.344508512903,60.1575729830521));
#98923=CARTESIAN_POINT('Ctrl Pts',(-11.8381254652903,600.195540415103,60.9355996838764));
#98924=CARTESIAN_POINT('Ctrl Pts',(-11.942724253673,600.132274080171,61.3285943265156));
#98925=CARTESIAN_POINT('Ctrl Pts',(-12.1975694083951,599.977328667355,62.5194580326036));
#98926=CARTESIAN_POINT('Ctrl Pts',(-12.289485607334,599.920336544294,63.3290997708905));
#98927=CARTESIAN_POINT('Ctrl Pts',(-12.3039937693074,599.911388735899,64.5687472338976));
#98928=CARTESIAN_POINT('Ctrl Pts',(-12.2877001556324,599.921457064597,64.9861606719559));
#98929=CARTESIAN_POINT('Ctrl Pts',(-12.2143945388426,599.966555320586,65.8053557663365));
#98930=CARTESIAN_POINT('Ctrl Pts',(-12.157513719035,600.001503621978,66.2102226898584));
#98931=CARTESIAN_POINT('Ctrl Pts',(-12.0043633846711,600.094884079366,67.0108131994228));
#98932=CARTESIAN_POINT('Ctrl Pts',(-11.9080923355525,600.153319701732,67.4065361653133));
#98933=CARTESIAN_POINT('Ctrl Pts',(-11.6759895729646,600.292636128654,68.1889168908538));
#98934=CARTESIAN_POINT('Ctrl Pts',(-11.5401719162743,600.373491958218,68.574557701102));
#98935=CARTESIAN_POINT('Ctrl Pts',(-11.0840493285825,600.641030827664,69.6921989559469));
#98936=CARTESIAN_POINT('Ctrl Pts',(-10.7131207478732,600.854147781253,70.3944487585354));
#98937=CARTESIAN_POINT('Ctrl Pts',(-10.0591458219388,601.211445845161,71.3889736072566));
#98938=CARTESIAN_POINT('Ctrl Pts',(-9.82548367484483,601.336394134174,71.709149064036));
#98939=CARTESIAN_POINT('Ctrl Pts',(-9.33415010121997,601.59145909223,72.3192655181611));
#98940=CARTESIAN_POINT('Ctrl Pts',(-9.07556749241062,601.722084359554,72.6106271901342));
#98941=CARTESIAN_POINT('Ctrl Pts',(-8.53249912601977,601.986550095139,73.1672612900657));
#98942=CARTESIAN_POINT('Ctrl Pts',(-8.24801593828978,602.120399261203,73.4325321421858));
#98943=CARTESIAN_POINT('Ctrl Pts',(-7.65202535438249,602.388174013953,73.9373693102728));
#98944=CARTESIAN_POINT('Ctrl Pts',(-7.33917816046283,602.522602244775,74.1777117225767));
#98945=CARTESIAN_POINT('Ctrl Pts',(-6.37510403592012,602.913420537684,74.8474837516201));
#98946=CARTESIAN_POINT('Ctrl Pts',(-5.69483978904818,603.159546862301,75.230310456561));
#98947=CARTESIAN_POINT('Ctrl Pts',(-4.61072722039349,603.483928244513,75.7094386141298));
#98948=CARTESIAN_POINT('Ctrl Pts',(-4.2386453508364,603.58453418778,75.8531520209646));
#98949=CARTESIAN_POINT('Ctrl Pts',(-3.47047139790995,603.76585931445,76.1066505694978));
#98950=CARTESIAN_POINT('Ctrl Pts',(-3.07637753452551,603.845878534603,76.215460838861));
#98951=CARTESIAN_POINT('Ctrl Pts',(-1.88763310249759,604.04373748117,76.4808614138366));
#98952=CARTESIAN_POINT('Ctrl Pts',(-1.07745358387034,604.121518543566,76.5802724694517));
#98953=CARTESIAN_POINT('Ctrl Pts',(-0.247612686332903,604.134451125088,
76.5969814761947));
#98954=CARTESIAN_POINT('Ctrl Pts',(1.87350135405495E-15,605.608439769695,
51.9994740882088));
#98955=CARTESIAN_POINT('Ctrl Pts',(-0.803517342471629,605.608439769695,
51.9994740882088));
#98956=CARTESIAN_POINT('Ctrl Pts',(-1.62216512710202,605.542186255804,52.0793396645949));
#98957=CARTESIAN_POINT('Ctrl Pts',(-3.23077935439454,605.286420618322,52.4030388996346));
#98958=CARTESIAN_POINT('Ctrl Pts',(-4.02089381669516,605.097608851242,52.6466899325635));
#98959=CARTESIAN_POINT('Ctrl Pts',(-6.27564182199435,604.41675711289,53.5959081295421));
#98960=CARTESIAN_POINT('Ctrl Pts',(-7.62604171070064,603.813936675359,54.5306889817204));
#98961=CARTESIAN_POINT('Ctrl Pts',(-9.75980156458901,602.747193352477,56.6644488356087));
#98962=CARTESIAN_POINT('Ctrl Pts',(-10.7006947361121,602.202165792572,58.017090947518));
#98963=CARTESIAN_POINT('Ctrl Pts',(-11.654095320228,601.628958177762,60.2816553316396));
#98964=CARTESIAN_POINT('Ctrl Pts',(-11.8983125166469,601.477289438537,61.0753972970467));
#98965=CARTESIAN_POINT('Ctrl Pts',(-12.2213288811781,601.275438695951,62.6858966089289));
#98966=CARTESIAN_POINT('Ctrl Pts',(-12.3,601.225373764374,63.5026943063123));
#98967=CARTESIAN_POINT('Ctrl Pts',(-12.3,601.225373764374,65.0962538701053));
#98968=CARTESIAN_POINT('Ctrl Pts',(-12.2213288811781,601.275438695951,65.9130515674887));
#98969=CARTESIAN_POINT('Ctrl Pts',(-11.8983125166469,601.477289438537,67.5235508793709));
#98970=CARTESIAN_POINT('Ctrl Pts',(-11.654095320228,601.628958177762,68.317292844778));
#98971=CARTESIAN_POINT('Ctrl Pts',(-10.7006947361121,602.202165792572,70.5818572288996));
#98972=CARTESIAN_POINT('Ctrl Pts',(-9.75980156458901,602.747193352477,71.9344993408089));
#98973=CARTESIAN_POINT('Ctrl Pts',(-7.62604171070064,603.813936675359,74.0682591946972));
#98974=CARTESIAN_POINT('Ctrl Pts',(-6.27564182199435,604.41675711289,75.0030400468755));
#98975=CARTESIAN_POINT('Ctrl Pts',(-4.02089381669516,605.097608851242,75.952258243854));
#98976=CARTESIAN_POINT('Ctrl Pts',(-3.23077935439458,605.286420618322,76.195909276783));
#98977=CARTESIAN_POINT('Ctrl Pts',(-1.62216512710205,605.542186255804,76.5196085118227));
#98978=CARTESIAN_POINT('Ctrl Pts',(-0.803517342471629,605.608439769695,
76.5994740882088));
#98979=CARTESIAN_POINT('Ctrl Pts',(2.63677968348475E-15,605.608439769695,
76.5994740882088));
#98980=CARTESIAN_POINT('Origin',(0.,1218.57245358804,64.2994740882088));
#98981=CARTESIAN_POINT('',(-1.09932974876048E-8,606.827140852494,48.5811983853019));
#98982=CARTESIAN_POINT('Ctrl Pts',(-6.34270402866122E-9,606.827140852493,
48.5811983853026));
#98983=CARTESIAN_POINT('Ctrl Pts',(0.131183067920692,606.827109872663,48.5812192224713));
#98984=CARTESIAN_POINT('Ctrl Pts',(0.262263850660884,606.825270297635,48.5828845405628));
#98985=CARTESIAN_POINT('Ctrl Pts',(0.393087042492152,606.82166339004,48.5861654542112));
#98986=CARTESIAN_POINT('Ctrl Pts',(0.625956739931848,606.815242972769,48.5920055912538));
#98987=CARTESIAN_POINT('Ctrl Pts',(0.858266994442126,606.803210550177,48.6029757350671));
#98988=CARTESIAN_POINT('Ctrl Pts',(1.08860828168967,606.78577822036,48.618932133042));
#98989=CARTESIAN_POINT('Ctrl Pts',(1.16869635359817,606.779717119892,48.62448006222));
#98990=CARTESIAN_POINT('Ctrl Pts',(1.24854641186113,606.773003566343,48.6306304686977));
#98991=CARTESIAN_POINT('Ctrl Pts',(1.32809942293837,606.765647546756,48.637376328015));
#98992=CARTESIAN_POINT('Ctrl Pts',(1.40535872090964,606.758503619687,48.6439276872661));
#98993=CARTESIAN_POINT('Ctrl Pts',(1.48241468364269,606.750760481874,48.6510297053401));
#98994=CARTESIAN_POINT('Ctrl Pts',(1.55926269747948,606.742431721439,48.6586783314213));
#98995=CARTESIAN_POINT('Ctrl Pts',(2.07067858640153,606.687004649108,48.7095791772737));
#98996=CARTESIAN_POINT('Ctrl Pts',(2.57353940461455,606.60556357932,48.7847527919497));
#98997=CARTESIAN_POINT('Ctrl Pts',(3.06861266584221,606.501763789166,48.8833382201712));
#98998=CARTESIAN_POINT('Ctrl Pts',(3.5280360180697,606.405438555533,48.9748245747402));
#98999=CARTESIAN_POINT('Ctrl Pts',(3.98077413585813,606.2898469916,49.0864791016381));
#99000=CARTESIAN_POINT('Ctrl Pts',(4.42735940791135,606.157954728535,49.2175762302821));
#99001=CARTESIAN_POINT('Ctrl Pts',(4.46201311942236,606.147720274511,49.2277489842));
#99002=CARTESIAN_POINT('Ctrl Pts',(4.49663613259049,606.137384633688,49.2380436267645));
#99003=CARTESIAN_POINT('Ctrl Pts',(4.53121896438333,606.12695270202,49.2484565026335));
#99004=CARTESIAN_POINT('Ctrl Pts',(4.74601947947585,606.062157999576,49.3131328459027));
#99005=CARTESIAN_POINT('Ctrl Pts',(4.95932213084444,605.993629202336,49.3823865525655));
#99006=CARTESIAN_POINT('Ctrl Pts',(5.16884411272973,605.92253759955,49.4553437713038));
#99007=CARTESIAN_POINT('Ctrl Pts',(5.41200740793915,605.840031371614,49.5400151626208));
#99008=CARTESIAN_POINT('Ctrl Pts',(5.65093526308688,605.753840160942,49.6299024007825));
#99009=CARTESIAN_POINT('Ctrl Pts',(5.8859656787125,605.664587255718,49.7248192945151));
#99010=CARTESIAN_POINT('Ctrl Pts',(5.9012058732883,605.658799785026,49.7309740380412));
#99011=CARTESIAN_POINT('Ctrl Pts',(5.91642974293557,605.652999506951,49.7371498648016));
#99012=CARTESIAN_POINT('Ctrl Pts',(5.93163735194618,605.647186561106,49.7433467521698));
#99013=CARTESIAN_POINT('Ctrl Pts',(6.38532277407425,605.47377016229,49.9282171982447));
#99014=CARTESIAN_POINT('Ctrl Pts',(6.82458941528544,605.289065018589,50.1318546390623));
#99015=CARTESIAN_POINT('Ctrl Pts',(7.25129724309775,605.096716462177,50.3537276895692));
#99016=CARTESIAN_POINT('Ctrl Pts',(7.67449000072657,604.905952406051,50.5737730273099));
#99017=CARTESIAN_POINT('Ctrl Pts',(8.08531522162717,604.707648175585,50.8117642540156));
#99018=CARTESIAN_POINT('Ctrl Pts',(8.48485213004562,604.504622243655,51.0679794092165));
#99019=CARTESIAN_POINT('Ctrl Pts',(8.50152150271616,604.496151649701,51.0786691498034));
#99020=CARTESIAN_POINT('Ctrl Pts',(8.51817133864071,604.487672771725,51.0893906828856));
#99021=CARTESIAN_POINT('Ctrl Pts',(8.53480170293739,604.479185821683,51.1001440211828));
#99022=CARTESIAN_POINT('Ctrl Pts',(8.88265589538547,604.301665888822,51.3250695695815));
#99023=CARTESIAN_POINT('Ctrl Pts',(9.22310591837765,604.119945955855,51.564885383951));
#99024=CARTESIAN_POINT('Ctrl Pts',(9.55213627055251,603.938098784817,51.8166263297717));
#99025=CARTESIAN_POINT('Ctrl Pts',(9.58597325041618,603.919397898944,51.8425149849012));
#99026=CARTESIAN_POINT('Ctrl Pts',(9.61968948708153,603.900695672363,51.8685297222792));
#99027=CARTESIAN_POINT('Ctrl Pts',(9.65328063531735,603.881996535394,51.8946672948334));
#99028=CARTESIAN_POINT('Ctrl Pts',(9.68287665471879,603.865521361142,51.917696221948));
#99029=CARTESIAN_POINT('Ctrl Pts',(9.71237647083121,603.849047630201,51.940821203202));
#99030=CARTESIAN_POINT('Ctrl Pts',(9.74177715342261,603.832578395773,51.9640400780151));
#99031=CARTESIAN_POINT('Ctrl Pts',(10.085743018819,603.63990074433,52.2356834435658));
#99032=CARTESIAN_POINT('Ctrl Pts',(10.4168996980707,603.447637351623,52.5202505899506));
#99033=CARTESIAN_POINT('Ctrl Pts',(10.7356021263374,603.25742169904,52.8182111751762));
#99034=CARTESIAN_POINT('Ctrl Pts',(11.1345671134278,603.019301814638,53.191210658376));
#99035=CARTESIAN_POINT('Ctrl Pts',(11.5140262355694,602.784321821904,53.5852075140256));
#99036=CARTESIAN_POINT('Ctrl Pts',(11.8747642121883,602.555396734084,54.0011669855163));
#99037=CARTESIAN_POINT('Ctrl Pts',(12.1396201387599,602.387318599316,54.3065668557228));
#99038=CARTESIAN_POINT('Ctrl Pts',(12.3942600538462,602.222458556566,54.6238994674662));
#99039=CARTESIAN_POINT('Ctrl Pts',(12.6384027128533,602.061913537245,54.9540941874028));
#99040=CARTESIAN_POINT('Ctrl Pts',(12.6934199989364,602.025734889511,55.0285032130265));
#99041=CARTESIAN_POINT('Ctrl Pts',(12.7479128130092,601.989770157807,55.1035770627712));
#99042=CARTESIAN_POINT('Ctrl Pts',(12.8018733060317,601.954035169909,55.1793208996343));
#99043=CARTESIAN_POINT('Ctrl Pts',(12.9672617185302,601.844507762207,55.4114750597183));
#99044=CARTESIAN_POINT('Ctrl Pts',(13.1265971638445,601.737833525833,55.6485181832555));
#99045=CARTESIAN_POINT('Ctrl Pts',(13.2794577936644,601.634588593285,55.8898965896893));
#99046=CARTESIAN_POINT('Ctrl Pts',(13.338098902136,601.594981290242,55.9824953008883));
#99047=CARTESIAN_POINT('Ctrl Pts',(13.3957875297173,601.555878461061,56.0757317394338));
#99048=CARTESIAN_POINT('Ctrl Pts',(13.4525014240595,601.517311758678,56.1695736395204));
#99049=CARTESIAN_POINT('Ctrl Pts',(13.5103276838369,601.477988623198,56.265256120072));
#99050=CARTESIAN_POINT('Ctrl Pts',(13.5671707966639,601.439201248967,56.3616179364094));
#99051=CARTESIAN_POINT('Ctrl Pts',(13.6230077720489,601.400982219844,56.4586314313638));
#99052=CARTESIAN_POINT('Ctrl Pts',(13.7869220361003,601.288786958761,56.7434229251517));
#99053=CARTESIAN_POINT('Ctrl Pts',(13.9424991854398,601.181288965271,57.034114638469));
#99054=CARTESIAN_POINT('Ctrl Pts',(14.0893519141326,601.079054705159,57.3308706561203));
#99055=CARTESIAN_POINT('Ctrl Pts',(14.1111562362249,601.063875220541,57.3749322397849));
#99056=CARTESIAN_POINT('Ctrl Pts',(14.132768292625,601.048811737215,57.4191274655816));
#99057=CARTESIAN_POINT('Ctrl Pts',(14.1541868887825,601.033866065188,57.4634568184053));
#99058=CARTESIAN_POINT('Ctrl Pts',(14.3690003859214,600.883971457167,57.9080491360308));
#99059=CARTESIAN_POINT('Ctrl Pts',(14.5644206321617,600.74588107374,58.3662732287448));
#99060=CARTESIAN_POINT('Ctrl Pts',(14.7394736989775,600.62123961036,58.8391490276349));
#99061=CARTESIAN_POINT('Ctrl Pts',(14.7930222736766,600.583111899524,58.9838013065173));
#99062=CARTESIAN_POINT('Ctrl Pts',(14.844665954123,600.546245890809,59.129826700604));
#99063=CARTESIAN_POINT('Ctrl Pts',(14.8943779224113,600.510686681454,59.2772573842497));
#99064=CARTESIAN_POINT('Ctrl Pts',(14.9788181415358,600.450286187705,59.5276815710471));
#99065=CARTESIAN_POINT('Ctrl Pts',(15.0576110594056,600.393686811632,59.7824113765591));
#99066=CARTESIAN_POINT('Ctrl Pts',(15.1295263785222,600.341868479667,60.0377155440763));
#99067=CARTESIAN_POINT('Ctrl Pts',(15.1536787692919,600.324465558871,60.1234581382101));
#99068=CARTESIAN_POINT('Ctrl Pts',(15.1770912859024,600.307576293993,60.2093651695768));
#99069=CARTESIAN_POINT('Ctrl Pts',(15.1997652434983,600.291202752349,60.2954371488871));
#99070=CARTESIAN_POINT('Ctrl Pts',(15.2446133607517,600.258816588073,60.4656838384653));
#99071=CARTESIAN_POINT('Ctrl Pts',(15.2865717155591,600.22845079911,60.636574808298));
#99072=CARTESIAN_POINT('Ctrl Pts',(15.325649598072,600.200124194892,60.8081106404716));
#99073=CARTESIAN_POINT('Ctrl Pts',(15.4433396652835,600.114813534744,61.3247216316376));
#99074=CARTESIAN_POINT('Ctrl Pts',(15.5349555636936,600.047977681829,61.8471715921895));
#99075=CARTESIAN_POINT('Ctrl Pts',(15.600123128367,600.000357873918,62.3755944903987));
#99076=CARTESIAN_POINT('Ctrl Pts',(15.6386979344604,599.972170157137,62.6883852312509));
#99077=CARTESIAN_POINT('Ctrl Pts',(15.6680084809615,599.950712943742,63.00326810169));
#99078=CARTESIAN_POINT('Ctrl Pts',(15.6877925284557,599.936218732362,63.3203069204358));
#99079=CARTESIAN_POINT('Ctrl Pts',(15.7005815679487,599.926849211701,63.5252509277185));
#99080=CARTESIAN_POINT('Ctrl Pts',(15.7093924335227,599.920387366526,63.731194673896));
#99081=CARTESIAN_POINT('Ctrl Pts',(15.7141470311175,599.916898340084,63.9378910949099));
#99082=CARTESIAN_POINT('Ctrl Pts',(15.7144659003351,599.916664346962,63.9517532829757));
#99083=CARTESIAN_POINT('Ctrl Pts',(15.7147665408604,599.916443713548,63.9656188529851));
#99084=CARTESIAN_POINT('Ctrl Pts',(15.7150489358492,599.916236454561,63.9794877289295));
#99085=CARTESIAN_POINT('Ctrl Pts',(15.7158488065306,599.915649403114,64.0187706754704));
#99086=CARTESIAN_POINT('Ctrl Pts',(15.7165007988266,599.915170663659,64.0581033421356));
#99087=CARTESIAN_POINT('Ctrl Pts',(15.7170049051664,599.914800215272,64.0974701301083));
#99088=CARTESIAN_POINT('Ctrl Pts',(15.7194694294047,599.912989131069,64.2899303224863));
#99089=CARTESIAN_POINT('Ctrl Pts',(15.7184018336157,599.913777206096,64.4836683248951));
#99090=CARTESIAN_POINT('Ctrl Pts',(15.7137735335997,599.917173057418,64.6767950132617));
#99091=CARTESIAN_POINT('Ctrl Pts',(15.712833394712,599.917862851051,64.716024516398));
#99092=CARTESIAN_POINT('Ctrl Pts',(15.7117464743577,599.918660143879,64.7552287682158));
#99093=CARTESIAN_POINT('Ctrl Pts',(15.7105127430939,599.919564854116,64.7943919360785));
#99094=CARTESIAN_POINT('Ctrl Pts',(15.7095991882977,599.92023477503,64.8233915252814));
#99095=CARTESIAN_POINT('Ctrl Pts',(15.708605979292,599.92096297442,64.8523701843884));
#99096=CARTESIAN_POINT('Ctrl Pts',(15.7075334205578,599.921749165278,64.8813270198615));
#99097=CARTESIAN_POINT('Ctrl Pts',(15.6985693797753,599.928319851522,65.1233373134135));
#99098=CARTESIAN_POINT('Ctrl Pts',(15.6840546075089,599.938957018774,65.3640472137197));
#99099=CARTESIAN_POINT('Ctrl Pts',(15.6641212610662,599.953549632281,65.6034907467274));
#99100=CARTESIAN_POINT('Ctrl Pts',(15.6411292069346,599.970381435241,65.8796761172172));
#99101=CARTESIAN_POINT('Ctrl Pts',(15.6110000935115,599.992447069947,66.1541909485691));
#99102=CARTESIAN_POINT('Ctrl Pts',(15.5737798644399,600.019643054132,66.4270558219922));
#99103=CARTESIAN_POINT('Ctrl Pts',(15.5042909343416,600.070417052335,66.9364854678731));
#99104=CARTESIAN_POINT('Ctrl Pts',(15.4100832406381,600.13907485609,67.4401695893287));
#99105=CARTESIAN_POINT('Ctrl Pts',(15.2914680739337,600.224933399288,67.9381923855767));
#99106=CARTESIAN_POINT('Ctrl Pts',(15.2270223963164,600.271581835144,68.2087768096833));
#99107=CARTESIAN_POINT('Ctrl Pts',(15.1553484481903,600.323324701704,68.4777850319379));
#99108=CARTESIAN_POINT('Ctrl Pts',(15.0765013223764,600.380048388059,68.7451756305374));
#99109=CARTESIAN_POINT('Ctrl Pts',(15.0102267686864,600.42772719636,68.969929448767));
#99110=CARTESIAN_POINT('Ctrl Pts',(14.9393986310139,600.478551665265,69.1917973879912));
#99111=CARTESIAN_POINT('Ctrl Pts',(14.8641408406389,600.532348321835,69.4108007082289));
#99112=CARTESIAN_POINT('Ctrl Pts',(14.6384917767306,600.693649432805,70.0674489297383));
#99113=CARTESIAN_POINT('Ctrl Pts',(14.3730295175932,600.881663250137,70.6983179949));
#99114=CARTESIAN_POINT('Ctrl Pts',(14.0709202551345,601.091836979959,71.3048669688541));
#99115=CARTESIAN_POINT('Ctrl Pts',(14.0153823306542,601.130474036763,71.4163712333539));
#99116=CARTESIAN_POINT('Ctrl Pts',(13.9586060318343,601.169859933587,71.5270536792301));
#99117=CARTESIAN_POINT('Ctrl Pts',(13.9006111685527,601.209966324507,71.6369234719541));
#99118=CARTESIAN_POINT('Ctrl Pts',(13.8132963508808,601.270348951737,71.8023391721821));
#99119=CARTESIAN_POINT('Ctrl Pts',(13.722999297798,601.332505688626,71.9661929969353));
#99120=CARTESIAN_POINT('Ctrl Pts',(13.6299592468021,601.396203040114,72.1281591912608));
#99121=CARTESIAN_POINT('Ctrl Pts',(13.5153701108117,601.474653389117,72.3276385130017));
#99122=CARTESIAN_POINT('Ctrl Pts',(13.3964238457257,601.555586127919,72.524588512448));
#99123=CARTESIAN_POINT('Ctrl Pts',(13.2736785048461,601.638477345278,72.7181535822209));
#99124=CARTESIAN_POINT('Ctrl Pts',(13.2230467223124,601.67266951959,72.7979981160226));
#99125=CARTESIAN_POINT('Ctrl Pts',(13.1717690142467,601.707194642083,72.877266958708));
#99126=CARTESIAN_POINT('Ctrl Pts',(13.119886458028,601.742014888341,72.9559013911626));
#99127=CARTESIAN_POINT('Ctrl Pts',(13.028077430013,601.803631223334,73.0950493310163));
#99128=CARTESIAN_POINT('Ctrl Pts',(12.9344479627768,601.866125360828,73.232156163104));
#99129=CARTESIAN_POINT('Ctrl Pts',(12.8390792114001,601.929383398044,73.367197238578));
#99130=CARTESIAN_POINT('Ctrl Pts',(12.6440223006845,602.058764533259,73.643395622445));
#99131=CARTESIAN_POINT('Ctrl Pts',(12.4414058536515,602.191546620317,73.9113615973352));
#99132=CARTESIAN_POINT('Ctrl Pts',(12.2313971791557,602.327125324242,74.1715598542876));
#99133=CARTESIAN_POINT('Ctrl Pts',(12.1400319511015,602.386109455412,74.2847602882354));
#99134=CARTESIAN_POINT('Ctrl Pts',(12.0472674516941,602.445624173488,74.3964896998921));
#99135=CARTESIAN_POINT('Ctrl Pts',(11.9530990206169,602.50562051508,74.506770281284));
#99136=CARTESIAN_POINT('Ctrl Pts',(11.7624766227194,602.627069352749,74.7300080333202));
#99137=CARTESIAN_POINT('Ctrl Pts',(11.5660389794749,602.750532246518,74.9473754835045));
#99138=CARTESIAN_POINT('Ctrl Pts',(11.3639002900369,602.875504933021,75.158894069929));
#99139=CARTESIAN_POINT('Ctrl Pts',(11.3241855659211,602.900058647999,75.2004516872687));
#99140=CARTESIAN_POINT('Ctrl Pts',(11.2842508843427,602.924670611825,75.2417836420512));
#99141=CARTESIAN_POINT('Ctrl Pts',(11.244097275529,602.949336959137,75.2828902591882));
#99142=CARTESIAN_POINT('Ctrl Pts',(11.1555970541534,603.003702612987,75.373490950486));
#99143=CARTESIAN_POINT('Ctrl Pts',(11.0659447322039,603.058384308477,75.463070243372));
#99144=CARTESIAN_POINT('Ctrl Pts',(10.9752166475744,603.113292912197,75.5515588294562));
#99145=CARTESIAN_POINT('Ctrl Pts',(10.7995114119639,603.21962965669,75.7229270218991));
#99146=CARTESIAN_POINT('Ctrl Pts',(10.6193973010466,603.327051486015,75.8905643475695));
#99147=CARTESIAN_POINT('Ctrl Pts',(10.4355011010676,603.434846331506,76.0538402392495));
#99148=CARTESIAN_POINT('Ctrl Pts',(10.3437034279004,603.488655578226,76.1353446256493));
#99149=CARTESIAN_POINT('Ctrl Pts',(10.2509639608671,603.54255759095,76.215762720377));
#99150=CARTESIAN_POINT('Ctrl Pts',(10.1573640686073,603.596463254928,76.2950194899588));
#99151=CARTESIAN_POINT('Ctrl Pts',(10.0741297969101,603.644399193455,76.3654990528508));
#99152=CARTESIAN_POINT('Ctrl Pts',(9.99030988510561,603.692296630999,76.4350092280443));
#99153=CARTESIAN_POINT('Ctrl Pts',(9.90591360420889,603.740115162276,76.5035433110902));
#99154=CARTESIAN_POINT('Ctrl Pts',(9.4063955163693,604.023139734598,76.9091774664249));
#99155=CARTESIAN_POINT('Ctrl Pts',(8.88565058296727,604.304165011645,77.281463795644));
#99156=CARTESIAN_POINT('Ctrl Pts',(8.34163289819202,604.577037261729,77.621886832962));
#99157=CARTESIAN_POINT('Ctrl Pts',(8.14290238271327,604.676717923657,77.746243903661));
#99158=CARTESIAN_POINT('Ctrl Pts',(7.94106647154317,604.775310977399,77.866349108996));
#99159=CARTESIAN_POINT('Ctrl Pts',(7.73602658782701,604.87251780605,77.982275225029));
#99160=CARTESIAN_POINT('Ctrl Pts',(7.67213350385386,604.902808713132,78.0183993045599));
#99161=CARTESIAN_POINT('Ctrl Pts',(7.607925744799,604.932962822967,78.0541135135407));
#99162=CARTESIAN_POINT('Ctrl Pts',(7.54339610210028,604.962967574738,78.0894159789354));
#99163=CARTESIAN_POINT('Ctrl Pts',(7.29105366481601,605.080300816876,78.2274658702299));
#99164=CARTESIAN_POINT('Ctrl Pts',(7.03370074023305,605.195402283494,78.3592633252969));
#99165=CARTESIAN_POINT('Ctrl Pts',(6.77108651639008,605.307447272327,78.4846057105468));
#99166=CARTESIAN_POINT('Ctrl Pts',(6.64811138532239,605.359914907116,78.543300156068));
#99167=CARTESIAN_POINT('Ctrl Pts',(6.52398298359675,605.411712539362,78.6005796581665));
#99168=CARTESIAN_POINT('Ctrl Pts',(6.39867799322463,605.462756977176,78.6564262110446));
#99169=CARTESIAN_POINT('Ctrl Pts',(6.34699373997078,605.483811155812,78.6794611067318));
#99170=CARTESIAN_POINT('Ctrl Pts',(6.29507802198154,605.504745800373,78.7022602318609));
#99171=CARTESIAN_POINT('Ctrl Pts',(6.24294708348502,605.525547606992,78.7248152334023));
#99172=CARTESIAN_POINT('Ctrl Pts',(5.9934113591915,605.625119838586,78.8327795019997));
#99173=CARTESIAN_POINT('Ctrl Pts',(5.73853110389339,605.721805612182,78.9353252138375));
#99174=CARTESIAN_POINT('Ctrl Pts',(5.48010053992522,605.814107611896,79.0314825681166));
#99175=CARTESIAN_POINT('Ctrl Pts',(5.31038406680991,605.874724164414,79.0946310083854));
#99176=CARTESIAN_POINT('Ctrl Pts',(5.13913733644966,605.933450239989,79.1550248358518));
#99177=CARTESIAN_POINT('Ctrl Pts',(4.96687438959262,605.989867757648,79.2123984530303));
#99178=CARTESIAN_POINT('Ctrl Pts',(4.93007196624935,606.001920850938,79.2246558083506));
#99179=CARTESIAN_POINT('Ctrl Pts',(4.89321390536558,606.013874408525,79.2367829629027));
#99180=CARTESIAN_POINT('Ctrl Pts',(4.85630009928057,606.02572615544,79.2487791179175));
#99181=CARTESIAN_POINT('Ctrl Pts',(4.25499476199429,606.218784510348,79.4441898003244));
#99182=CARTESIAN_POINT('Ctrl Pts',(3.63825269281664,606.385103343078,79.6050498204426));
#99183=CARTESIAN_POINT('Ctrl Pts',(3.00303825816605,606.515495744393,79.7285331847965));
#99184=CARTESIAN_POINT('Ctrl Pts',(2.6393277264934,606.590155712778,79.7992371827726));
#99185=CARTESIAN_POINT('Ctrl Pts',(2.26956149135921,606.6530382001,79.8576872889477));
#99186=CARTESIAN_POINT('Ctrl Pts',(1.89317385967764,606.70242510632,79.9033533194805));
#99187=CARTESIAN_POINT('',(-7.31873414160669E-15,608.476132031997,48.5811677441054));
#99188=CARTESIAN_POINT('',(1.92493735523237E-15,1218.57245358804,48.5811677441054));
#99189=CARTESIAN_POINT('Ctrl Pts',(3.93978362444746,607.874843764614,49.082928510463));
#99190=CARTESIAN_POINT('Ctrl Pts',(3.62591964374305,607.968397240746,49.0016645885587));
#99191=CARTESIAN_POINT('Ctrl Pts',(3.30579924060091,608.053570299406,48.9292260493855));
#99192=CARTESIAN_POINT('Ctrl Pts',(2.66144129984969,608.201953140762,48.8046503202028));
#99193=CARTESIAN_POINT('Ctrl Pts',(2.3359974548026,608.265536826742,48.7521822712622));
#99194=CARTESIAN_POINT('Ctrl Pts',(1.67806442767431,608.369017250152,48.6674791187011));
#99195=CARTESIAN_POINT('Ctrl Pts',(1.34557472886657,608.408910004209,48.6352427984729));
#99196=CARTESIAN_POINT('Ctrl Pts',(0.672995467599795,608.462621079598,48.5919666363597));
#99197=CARTESIAN_POINT('Ctrl Pts',(0.334567964264235,608.476132031997,48.5811677441054));
#99198=CARTESIAN_POINT('Ctrl Pts',(-7.31873414160669E-15,608.476132031997,
48.5811677441054));
#99199=CARTESIAN_POINT('Ctrl Pts',(-7.31873414160669E-15,608.476132031997,
48.5811677441054));
#99200=CARTESIAN_POINT('Ctrl Pts',(-1.00038541833525,608.476132031997,48.5811677441054));
#99201=CARTESIAN_POINT('Ctrl Pts',(-1.98186107540155,608.355804039834,48.6756960232106));
#99202=CARTESIAN_POINT('Ctrl Pts',(-3.18805636841628,608.0812830782,48.9059115645402));
#99203=CARTESIAN_POINT('Ctrl Pts',(-3.42854858272458,608.0201047022,48.9577280742447));
#99204=CARTESIAN_POINT('Ctrl Pts',(-3.9008061116148,607.88835111953,49.0709538770827));
#99205=CARTESIAN_POINT('Ctrl Pts',(-4.13345843873349,607.817596758595,49.1325121211066));
#99206=CARTESIAN_POINT('Ctrl Pts',(-4.82191402968074,607.59267130225,49.3314235132617));
#99207=CARTESIAN_POINT('Ctrl Pts',(-5.26825798195031,607.4259010746,49.4829579943547));
#99208=CARTESIAN_POINT('Ctrl Pts',(-6.13948585279377,607.067521867576,49.8222366173663));
#99209=CARTESIAN_POINT('Ctrl Pts',(-6.56545659234339,606.875360414686,50.0105449985554));
#99210=CARTESIAN_POINT('Ctrl Pts',(-7.39359379433368,606.47552949295,50.4209480281591));
#99211=CARTESIAN_POINT('Ctrl Pts',(-7.79284032142572,606.269378077533,50.6414529752954));
#99212=CARTESIAN_POINT('Ctrl Pts',(-8.95204291419482,605.641124055901,51.3478306146848));
#99213=CARTESIAN_POINT('Ctrl Pts',(-9.6739937385886,605.209537903166,51.8780902826517));
#99214=CARTESIAN_POINT('Ctrl Pts',(-10.6909797044834,604.568043191503,52.7681666459264));
#99215=CARTESIAN_POINT('Ctrl Pts',(-11.018834746685,604.355085789127,53.0807607042935));
#99216=CARTESIAN_POINT('Ctrl Pts',(-11.6523858512663,603.934348995513,53.7403002029845));
#99217=CARTESIAN_POINT('Ctrl Pts',(-11.9552766171641,603.728415571992,54.0845026139995));
#99218=CARTESIAN_POINT('Ctrl Pts',(-12.8157642528714,603.133398024851,55.1530076404017));
#99219=CARTESIAN_POINT('Ctrl Pts',(-13.3290592983858,602.764738088077,55.9162808887406));
#99220=CARTESIAN_POINT('Ctrl Pts',(-14.004746121757,602.270400060673,57.1474541420456));
#99221=CARTESIAN_POINT('Ctrl Pts',(-14.2141395881851,602.115412268844,57.5723098240839));
#99222=CARTESIAN_POINT('Ctrl Pts',(-14.5988681163382,601.828423328471,58.4540012253265));
#99223=CARTESIAN_POINT('Ctrl Pts',(-14.774314469106,601.696323764207,58.9121779826557));
#99224=CARTESIAN_POINT('Ctrl Pts',(-15.2329469259702,601.34910589721,60.3025784912361));
#99225=CARTESIAN_POINT('Ctrl Pts',(-15.4543798168271,601.178811145537,61.2611681259982));
#99226=CARTESIAN_POINT('Ctrl Pts',(-15.6499076381601,601.02822212081,62.7513958204655));
#99227=CARTESIAN_POINT('Ctrl Pts',(-15.6916676668363,600.995953718117,63.2567226635694));
#99228=CARTESIAN_POINT('Ctrl Pts',(-15.7262198238666,600.969261205682,64.2573462892223));
#99229=CARTESIAN_POINT('Ctrl Pts',(-15.7195678789232,600.974407590695,64.7561248933746));
#99230=CARTESIAN_POINT('Ctrl Pts',(-15.6590995589811,601.021098663315,65.7506616225585));
#99231=CARTESIAN_POINT('Ctrl Pts',(-15.6052831790191,601.062644377796,66.2464197156399));
#99232=CARTESIAN_POINT('Ctrl Pts',(-15.4498800061554,601.182160079324,67.2348902714699));
#99233=CARTESIAN_POINT('Ctrl Pts',(-15.3482435235833,601.260162049379,67.7257307925787));
#99234=CARTESIAN_POINT('Ctrl Pts',(-14.9812478047689,601.540233943488,69.1572522104259));
#99235=CARTESIAN_POINT('Ctrl Pts',(-14.6526793160863,601.789458207514,70.0696014607015));
#99236=CARTESIAN_POINT('Ctrl Pts',(-13.8372960983329,602.394765535271,71.8177596455625));
#99237=CARTESIAN_POINT('Ctrl Pts',(-13.3616578586644,602.742527172046,72.6296038086577));
#99238=CARTESIAN_POINT('Ctrl Pts',(-12.2895634342419,603.50114039407,74.1428267938299));
#99239=CARTESIAN_POINT('Ctrl Pts',(-11.6877930740782,603.915615183279,74.8486713035806));
#99240=CARTESIAN_POINT('Ctrl Pts',(-10.3949373649157,604.761836407664,76.1246737064291));
#99241=CARTESIAN_POINT('Ctrl Pts',(-9.70188800092167,605.195554364056,76.6994753988773));
#99242=CARTESIAN_POINT('Ctrl Pts',(-8.58467388731213,605.839463452404,77.4742190882292));
#99243=CARTESIAN_POINT('Ctrl Pts',(-8.19773601749983,606.05368580674,77.7185803584321));
#99244=CARTESIAN_POINT('Ctrl Pts',(-7.40176600282271,606.47083721012,78.1735199632814));
#99245=CARTESIAN_POINT('Ctrl Pts',(-6.99390219741844,606.673234514064,78.3836222033658));
#99246=CARTESIAN_POINT('Ctrl Pts',(-5.73705816174997,607.252779638758,78.9624303035971));
#99247=CARTESIAN_POINT('Ctrl Pts',(-4.8557807881079,607.603554702388,79.2806298462149));
#99248=CARTESIAN_POINT('Ctrl Pts',(-3.91253447320281,607.88294039512,79.5230488432747));
#99249=CARTESIAN_POINT('Ctrl Pts',(-1.91941230150446,606.698958856847,48.698800681464));
#99250=CARTESIAN_POINT('Ctrl Pts',(-1.77856148952992,606.717691793978,48.6814712512444));
#99251=CARTESIAN_POINT('Ctrl Pts',(-1.63703421267371,606.734446862159,48.6660258498612));
#99252=CARTESIAN_POINT('Ctrl Pts',(-1.49482298761707,606.749197548788,48.6524629893762));
#99253=CARTESIAN_POINT('Ctrl Pts',(-1.47848330594896,606.750892362428,48.6509046537192));
#99254=CARTESIAN_POINT('Ctrl Pts',(-1.4621345691852,606.752560679373,48.6493712049886));
#99255=CARTESIAN_POINT('Ctrl Pts',(-1.44577674730114,606.754202430862,48.647862668289));
#99256=CARTESIAN_POINT('Ctrl Pts',(-1.30269956743955,606.76856236061,48.6346679301252));
#99257=CARTESIAN_POINT('Ctrl Pts',(-1.15892868452667,606.780892900214,48.6233762927986));
#99258=CARTESIAN_POINT('Ctrl Pts',(-1.01444129745525,606.791127273198,48.6140239791455));
#99259=CARTESIAN_POINT('Ctrl Pts',(-0.998637300191364,606.792246706568,
48.6130010252228));
#99260=CARTESIAN_POINT('Ctrl Pts',(-0.98282472172319,606.79334102437,48.6120013076366));
#99261=CARTESIAN_POINT('Ctrl Pts',(-0.967003526926913,606.79441011141,48.6110248994056));
#99262=CARTESIAN_POINT('Ctrl Pts',(-0.806537717335273,606.805253282208,
48.6011217195697));
#99263=CARTESIAN_POINT('Ctrl Pts',(-0.645476066513777,606.813481813266,
48.5936338603989));
#99264=CARTESIAN_POINT('Ctrl Pts',(-0.484183920938916,606.818964448633,
48.588641220104));
#99265=CARTESIAN_POINT('Ctrl Pts',(-0.422615490343729,606.82105727996,48.586735429674));
#99266=CARTESIAN_POINT('Ctrl Pts',(-0.361005641426017,606.822749448665,
48.58519312428));
#99267=CARTESIAN_POINT('Ctrl Pts',(-0.29939725843297,606.824040854733,48.5840194145379));
#99268=CARTESIAN_POINT('Ctrl Pts',(-0.280307236559404,606.82444101083,48.5836557279167));
#99269=CARTESIAN_POINT('Ctrl Pts',(-0.261214851172684,606.824802746722,
48.5833273536881));
#99270=CARTESIAN_POINT('Ctrl Pts',(-0.242121350637935,606.825126404318,
48.5830342121591));
#99271=CARTESIAN_POINT('Ctrl Pts',(-0.161408243682281,606.826494587699,
48.5817950279905));
#99272=CARTESIAN_POINT('Ctrl Pts',(-0.0806852921308739,606.827159906852,
48.5811855692694));
#99273=CARTESIAN_POINT('Ctrl Pts',(-1.56438910714485E-8,606.827140852495,
48.5811983853012));
#99274=CARTESIAN_POINT('Ctrl Pts',(-19.6604693917099,639.614613618721,62.5660159449655));
#99275=CARTESIAN_POINT('Ctrl Pts',(-19.6043473940929,640.042864396936,62.5045768852686));
#99276=CARTESIAN_POINT('Ctrl Pts',(-19.1902534503917,640.029230307342,62.3679625261942));
#99277=CARTESIAN_POINT('Ctrl Pts',(-19.5362970273361,639.656420566866,62.9361067570152));
#99278=CARTESIAN_POINT('Ctrl Pts',(-19.4739947450425,640.077793049794,62.8838115245112));
#99279=CARTESIAN_POINT('Ctrl Pts',(-19.0563824034601,640.070385553537,62.780340451598));
#99280=CARTESIAN_POINT('Ctrl Pts',(-19.4529721346903,639.685402500002,63.3126278577785));
#99281=CARTESIAN_POINT('Ctrl Pts',(-19.3848517001577,640.102600286318,63.2753840449119));
#99282=CARTESIAN_POINT('Ctrl Pts',(-18.9665644890546,640.098956603779,63.199877359281));
#99283=CARTESIAN_POINT('Ctrl Pts',(-19.3883804561941,639.707874785332,63.8868784008059));
#99284=CARTESIAN_POINT('Ctrl Pts',(-19.3163013556422,640.121692201212,63.8713399627084));
#99285=CARTESIAN_POINT('Ctrl Pts',(-18.8969388964883,640.121110791056,63.8397379568555));
#99286=CARTESIAN_POINT('Ctrl Pts',(-19.3769841736612,639.711863719473,64.0798899164937));
#99287=CARTESIAN_POINT('Ctrl Pts',(-19.3041878248497,640.12508992708,64.0717390566854));
#99288=CARTESIAN_POINT('Ctrl Pts',(-18.8846548024122,640.125044298213,64.0548016868818));
#99289=CARTESIAN_POINT('Ctrl Pts',(-19.375186673142,639.71249178762,64.4692203034188));
#99290=CARTESIAN_POINT('Ctrl Pts',(-19.3022819370354,640.125623427249,64.4755024746936));
#99291=CARTESIAN_POINT('Ctrl Pts',(-18.8827172550505,640.125663592786,64.4886143790017));
#99292=CARTESIAN_POINT('Ctrl Pts',(-19.3849840685433,639.709061256727,64.6658272951823));
#99293=CARTESIAN_POINT('Ctrl Pts',(-19.3126965606472,640.12270098294,64.6796458141313));
#99294=CARTESIAN_POINT('Ctrl Pts',(-18.8932778841669,640.122280676192,64.707684380311));
#99295=CARTESIAN_POINT('Ctrl Pts',(-19.4452767686435,639.688071722563,65.2450126378428));
#99296=CARTESIAN_POINT('Ctrl Pts',(-19.3766820633375,640.104867502093,65.2807205567288));
#99297=CARTESIAN_POINT('Ctrl Pts',(-18.9582692702832,640.101587693298,65.3530435950167));
#99298=CARTESIAN_POINT('Ctrl Pts',(-19.526131319747,639.65992314981,65.6222918010434));
#99299=CARTESIAN_POINT('Ctrl Pts',(-19.4631745914249,640.080771137981,65.6731048965284));
#99300=CARTESIAN_POINT('Ctrl Pts',(-19.0454249069794,640.073836781612,65.7734281706718));
#99301=CARTESIAN_POINT('Ctrl Pts',(-19.7068251736695,639.59897289078,66.1753917003921));
#99302=CARTESIAN_POINT('Ctrl Pts',(-19.6535908638706,640.029636059382,66.2421063751751));
#99303=CARTESIAN_POINT('Ctrl Pts',(-19.2402290736399,640.013832011843,66.3897215922081));
#99304=CARTESIAN_POINT('Ctrl Pts',(-19.7773500518966,639.575429358817,66.3580430271829));
#99305=CARTESIAN_POINT('Ctrl Pts',(-19.7282627805238,640.009830550918,66.4305066259489));
#99306=CARTESIAN_POINT('Ctrl Pts',(-19.3162648045463,639.990664629944,66.5932414468988));
#99307=CARTESIAN_POINT('Ctrl Pts',(-19.9349482970738,639.523774305166,66.7110781169987));
#99308=CARTESIAN_POINT('Ctrl Pts',(-19.8945480523043,639.966662205344,66.7935682190135));
#99309=CARTESIAN_POINT('Ctrl Pts',(-19.4861918640954,639.939877906828,66.9866119824641));
#99310=CARTESIAN_POINT('Ctrl Pts',(-20.0222946068357,639.495568525969,66.8824893749696));
#99311=CARTESIAN_POINT('Ctrl Pts',(-19.9867696521186,639.943145147396,66.969541097156));
#99312=CARTESIAN_POINT('Ctrl Pts',(-19.5803774190672,639.912165675139,67.1776075526048));
#99313=CARTESIAN_POINT('Ctrl Pts',(-20.2134165147897,639.435245715633,67.2155869499658));
#99314=CARTESIAN_POINT('Ctrl Pts',(-20.1878269004917,639.893224462444,67.3103559506421));
#99315=CARTESIAN_POINT('Ctrl Pts',(-19.7864846440742,639.852963266996,67.5487626450847));
#99316=CARTESIAN_POINT('Ctrl Pts',(-20.3171936898167,639.403126937874,67.3772721460263));
#99317=CARTESIAN_POINT('Ctrl Pts',(-20.2970154844049,639.866746775558,67.47535656416));
#99318=CARTESIAN_POINT('Ctrl Pts',(-19.8984079972179,639.821471319271,67.7289209182822));
#99319=CARTESIAN_POINT('Ctrl Pts',(-20.5410431146462,639.33577623417,67.6911018289748));
#99320=CARTESIAN_POINT('Ctrl Pts',(-20.5315995437245,639.811706987032,67.7943468231785));
#99321=CARTESIAN_POINT('Ctrl Pts',(-20.1398571470931,639.755528739292,68.078606697025));
#99322=CARTESIAN_POINT('Ctrl Pts',(-20.66161879079,639.300409001074,67.8437149881379));
#99323=CARTESIAN_POINT('Ctrl Pts',(-20.6578743308502,639.782976975004,67.9488690872092));
#99324=CARTESIAN_POINT('Ctrl Pts',(-20.2699261878463,639.720946438105,68.2486564224931));
#99325=CARTESIAN_POINT('Ctrl Pts',(-21.0408663871178,639.192912656625,68.2791535667018));
#99326=CARTESIAN_POINT('Ctrl Pts',(-21.0562413302891,639.695892337362,68.3909401809132));
#99327=CARTESIAN_POINT('Ctrl Pts',(-20.6790881543741,639.616027662147,68.7338453225555));
#99328=CARTESIAN_POINT('Ctrl Pts',(-21.3184472555098,639.118885613595,68.5424636157139));
#99329=CARTESIAN_POINT('Ctrl Pts',(-21.345483233491,639.637322639742,68.6531058695304));
#99330=CARTESIAN_POINT('Ctrl Pts',(-20.9786322139011,639.544022285944,69.0272394297093));
#99331=CARTESIAN_POINT('Ctrl Pts',(-21.921761724668,638.973297071061,69.0180659887194));
#99332=CARTESIAN_POINT('Ctrl Pts',(-21.9667100270014,639.525213923758,69.1216530518533));
#99333=CARTESIAN_POINT('Ctrl Pts',(-21.6299071797506,639.403272217871,69.5571809714726));
#99334=CARTESIAN_POINT('Ctrl Pts',(-22.2494126434192,638.901508308394,69.2305907102972));
#99335=CARTESIAN_POINT('Ctrl Pts',(-22.3020685690074,639.471693284507,69.3264745684198));
#99336=CARTESIAN_POINT('Ctrl Pts',(-21.9837112677507,639.334322479089,69.7939873572225));
#99337=CARTESIAN_POINT('Ctrl Pts',(-22.9292469963058,638.772850945573,69.5887280397824));
#99338=CARTESIAN_POINT('Ctrl Pts',(-22.9897008093125,639.379125595584,69.667121205382));
#99339=CARTESIAN_POINT('Ctrl Pts',(-22.7181072739011,639.212144997237,70.1930430801067));
#99340=CARTESIAN_POINT('Ctrl Pts',(-23.2840893761466,638.715229200386,69.7368588847111));
#99341=CARTESIAN_POINT('Ctrl Pts',(-23.3447311905104,639.340004169329,69.8029639541895));
#99342=CARTESIAN_POINT('Ctrl Pts',(-23.1015678781488,639.158182199808,70.3580983729776));
#99343=CARTESIAN_POINT('Ctrl Pts',(-23.8400397081407,638.643801346691,69.9110832725672));
#99344=CARTESIAN_POINT('Ctrl Pts',(-23.8907379099241,639.294626550114,69.958336958928));
#99345=CARTESIAN_POINT('Ctrl Pts',(-23.7026318796329,639.093034350673,70.5522284812034));
#99346=CARTESIAN_POINT('Ctrl Pts',(-24.0301388274256,638.622452400188,69.9611880307775));
#99347=CARTESIAN_POINT('Ctrl Pts',(-24.0776195734464,639.281653485817,70.002165703523));
#99348=CARTESIAN_POINT('Ctrl Pts',(-23.9082019757128,639.073922036048,70.6080578768363));
#99349=CARTESIAN_POINT('Ctrl Pts',(-24.410372221457,638.58639745276,70.0426866143446));
#99350=CARTESIAN_POINT('Ctrl Pts',(-24.4496351039123,639.2609913659,70.0718111149744));
#99351=CARTESIAN_POINT('Ctrl Pts',(-24.3194774954357,639.042533755913,70.6988679476676));
#99352=CARTESIAN_POINT('Ctrl Pts',(-24.601335407632,638.571560050251,70.074414171567));
#99353=CARTESIAN_POINT('Ctrl Pts',(-24.6352021221028,639.253302178315,70.0976274626793));
#99354=CARTESIAN_POINT('Ctrl Pts',(-24.526078729531,639.030135030137,70.7342204849604));
#99355=CARTESIAN_POINT('Ctrl Pts',(-25.1767601479727,638.537133522905,70.1426665970483));
#99356=CARTESIAN_POINT('Ctrl Pts',(-25.1955539595057,639.23785273376,70.1500812974023));
#99357=CARTESIAN_POINT('Ctrl Pts',(-25.1487757592767,639.003355461779,70.8102709790819));
#99358=CARTESIAN_POINT('Ctrl Pts',(-25.563731151051,638.527630622351,70.1525518511399));
#99359=CARTESIAN_POINT('Ctrl Pts',(-25.5643966079534,639.238200260492,70.1503052553348));
#99360=CARTESIAN_POINT('Ctrl Pts',(-25.5677370210007,638.999391403185,70.8212856580984));
#99361=CARTESIAN_POINT('Ctrl Pts',(-26.3449430775709,638.538201511733,70.0952068196612));
#99362=CARTESIAN_POINT('Ctrl Pts',(-26.3101215344426,639.259956556377,70.0813790172625));
#99363=CARTESIAN_POINT('Ctrl Pts',(-26.4139660749482,639.022007969339,70.7573887616778));
#99364=CARTESIAN_POINT('Ctrl Pts',(-26.7282279181265,638.55827679445,70.0283683140306));
#99365=CARTESIAN_POINT('Ctrl Pts',(-26.6721307562498,639.281238556969,70.0125473081986));
#99366=CARTESIAN_POINT('Ctrl Pts',(-26.8293681462139,639.048425499655,70.6829137334035));
#99367=CARTESIAN_POINT('Ctrl Pts',(-27.2841361653692,638.607369964634,69.8731681263508));
#99368=CARTESIAN_POINT('Ctrl Pts',(-27.2028933885728,639.326706258709,69.8587349175253));
#99369=CARTESIAN_POINT('Ctrl Pts',(-27.4321510026923,639.107297343891,70.5099814025619));
#99370=CARTESIAN_POINT('Ctrl Pts',(-27.4667215187653,638.626901856262,69.8121804983067));
#99371=CARTESIAN_POINT('Ctrl Pts',(-27.3772534188525,639.344086126414,69.7991077552769));
#99372=CARTESIAN_POINT('Ctrl Pts',(-27.63018197883,639.130139927938,70.4420257333318));
#99373=CARTESIAN_POINT('Ctrl Pts',(-27.8263762321758,638.671746207838,69.6711847249545));
#99374=CARTESIAN_POINT('Ctrl Pts',(-27.7224215060154,639.383169440062,69.6618289971831));
#99375=CARTESIAN_POINT('Ctrl Pts',(-28.0203545837303,639.181690618376,70.2849207185056));
#99376=CARTESIAN_POINT('Ctrl Pts',(-28.0042122567427,638.697208341129,69.5906848480275));
#99377=CARTESIAN_POINT('Ctrl Pts',(-27.8935367666387,639.404934118318,69.5839425890701));
#99378=CARTESIAN_POINT('Ctrl Pts',(-28.2133287232379,639.210564262153,70.1952234599579));
#99379=CARTESIAN_POINT('Ctrl Pts',(-28.517678386789,638.779374195469,69.3254946573024));
#99380=CARTESIAN_POINT('Ctrl Pts',(-28.3889976863558,639.474465198322,69.3278776694702));
#99381=CARTESIAN_POINT('Ctrl Pts',(-28.7706297699789,639.302831299308,69.8997343998282));
#99382=CARTESIAN_POINT('Ctrl Pts',(-28.8368019609363,638.842144825035,69.1164244028433));
#99383=CARTESIAN_POINT('Ctrl Pts',(-28.7004074914826,639.526813318195,69.1267051815092));
#99384=CARTESIAN_POINT('Ctrl Pts',(-29.1171684630673,639.372219716366,69.6667771654812));
#99385=CARTESIAN_POINT('Ctrl Pts',(-29.2821652331234,638.942012522508,68.754787226998));
#99386=CARTESIAN_POINT('Ctrl Pts',(-29.1426111606792,639.611228165578,68.7725889580942));
#99387=CARTESIAN_POINT('Ctrl Pts',(-29.6009713712576,639.481679229375,69.2638217267234));
#99388=CARTESIAN_POINT('Ctrl Pts',(-29.4257458324037,638.976445684631,68.6254237801236));
#99389=CARTESIAN_POINT('Ctrl Pts',(-29.2853375079637,639.640235865451,68.6462428574156));
#99390=CARTESIAN_POINT('Ctrl Pts',(-29.7569772664138,639.519269640047,69.1196780709533));
#99391=CARTESIAN_POINT('Ctrl Pts',(-29.6975535013539,639.045172134778,68.3539257857801));
#99392=CARTESIAN_POINT('Ctrl Pts',(-29.5569080178443,639.698370750662,68.3797876371925));
#99393=CARTESIAN_POINT('Ctrl Pts',(-30.0523587091175,639.594075821366,68.8171605190338));
#99394=CARTESIAN_POINT('Ctrl Pts',(-29.8255815043549,639.079383885521,68.2121761101742));
#99395=CARTESIAN_POINT('Ctrl Pts',(-29.6856009206759,639.727412866963,68.2402497616682));
#99396=CARTESIAN_POINT('Ctrl Pts',(-30.1915174672224,639.631204693504,68.6592154660613));
#99397=CARTESIAN_POINT('Ctrl Pts',(-30.1870135856361,639.180024049103,67.7693531242958));
#99398=CARTESIAN_POINT('Ctrl Pts',(-30.0486031852443,639.812777163191,67.804557648681));
#99399=CARTESIAN_POINT('Ctrl Pts',(-30.5844318653539,639.740197922646,68.1657984662501));
#99400=CARTESIAN_POINT('Ctrl Pts',(-30.3980015252607,639.244468011042,67.4508867391265));
#99401=CARTESIAN_POINT('Ctrl Pts',(-30.2645436408508,639.868308369816,67.4876764108793));
#99402=CARTESIAN_POINT('Ctrl Pts',(-30.8138811498187,639.809683374485,67.8109462262171));
#99403=CARTESIAN_POINT('Ctrl Pts',(-30.7593869387953,639.360204041504,66.7653665317526));
#99404=CARTESIAN_POINT('Ctrl Pts',(-30.6352574879512,639.968523506671,66.8008921937396));
#99405=CARTESIAN_POINT('Ctrl Pts',(-31.206966008069,639.934210074654,67.047103030666));
#99406=CARTESIAN_POINT('Ctrl Pts',(-30.9041015064952,639.409625712735,66.4088790927884));
#99407=CARTESIAN_POINT('Ctrl Pts',(-30.7858111889449,640.01191089884,66.4409608338525));
#99408=CARTESIAN_POINT('Ctrl Pts',(-31.3644198481214,639.987241357622,66.6498843590981));
#99409=CARTESIAN_POINT('Ctrl Pts',(-31.0141476947143,639.44800149248,66.0405185693756));
#99410=CARTESIAN_POINT('Ctrl Pts',(-30.9005396207576,640.045728745606,66.0664164809275));
#99411=CARTESIAN_POINT('Ctrl Pts',(-31.484164369445,640.02838482468,66.2394387527513));
#99412=CARTESIAN_POINT('',(-31.0141476947143,639.44800149248,66.0405185693756));
#99413=CARTESIAN_POINT('',(-19.3760282912166,639.712197922296,64.2994740881845));
#99414=CARTESIAN_POINT('Ctrl Pts',(-31.0141476947143,639.44800149248,66.0405185693756));
#99415=CARTESIAN_POINT('Ctrl Pts',(-30.964172162317,639.430573810473,66.2078029936897));
#99416=CARTESIAN_POINT('Ctrl Pts',(-30.9070963674012,639.410889044142,66.3724853570777));
#99417=CARTESIAN_POINT('Ctrl Pts',(-30.8427717435498,639.389175714363,66.5345397812563));
#99418=CARTESIAN_POINT('Ctrl Pts',(-30.7784471196983,639.367462384584,66.6965942054349));
#99419=CARTESIAN_POINT('Ctrl Pts',(-30.7068738047457,639.343720218765,66.8560208760923));
#99420=CARTESIAN_POINT('Ctrl Pts',(-30.6278540796739,639.318163608302,67.0127761790815));
#99421=CARTESIAN_POINT('Ctrl Pts',(-30.6117724312023,639.312962471178,67.0446781336433));
#99422=CARTESIAN_POINT('Ctrl Pts',(-30.5953858009309,639.307687752954,67.0764620783354));
#99423=CARTESIAN_POINT('Ctrl Pts',(-30.5786931148851,639.302341438801,67.1081269277583));
#99424=CARTESIAN_POINT('Ctrl Pts',(-30.4687474822263,639.267128178916,67.3166860472013));
#99425=CARTESIAN_POINT('Ctrl Pts',(-30.3476320077173,639.229502304161,67.5161693060764));
#99426=CARTESIAN_POINT('Ctrl Pts',(-30.2153800827863,639.190321630889,67.7069108282264));
#99427=CARTESIAN_POINT('Ctrl Pts',(-30.1703849865028,639.17699147961,67.771805408467));
#99428=CARTESIAN_POINT('Ctrl Pts',(-30.1241004869899,639.163481279123,67.8356878427701));
#99429=CARTESIAN_POINT('Ctrl Pts',(-30.0765268382153,639.149824622943,67.8985704517844));
#99430=CARTESIAN_POINT('Ctrl Pts',(-30.0340673542078,639.137636056591,67.9546931836028));
#99431=CARTESIAN_POINT('Ctrl Pts',(-29.9905766274731,639.125330676828,68.0100248730267));
#99432=CARTESIAN_POINT('Ctrl Pts',(-29.9460581899746,639.112933745349,68.0645685899863));
#99433=CARTESIAN_POINT('Ctrl Pts',(-29.825600346812,639.079390168538,68.2121528016568));
#99434=CARTESIAN_POINT('Ctrl Pts',(-29.6975577157899,639.045173518059,68.3539215227992));
#99435=CARTESIAN_POINT('Ctrl Pts',(-29.5616496471025,639.010809002831,68.4896747861607));
#99436=CARTESIAN_POINT('Ctrl Pts',(-29.5009767263279,638.995467783358,68.550278597784));
#99437=CARTESIAN_POINT('Ctrl Pts',(-29.4387762621089,638.980113378838,68.6096070566503));
#99438=CARTESIAN_POINT('Ctrl Pts',(-29.3753030064446,638.964854823256,68.6674399705206));
#99439=CARTESIAN_POINT('Ctrl Pts',(-29.2965613930307,638.945925854318,68.7391844698206));
#99440=CARTESIAN_POINT('Ctrl Pts',(-29.2158764789106,638.927149530007,68.8086138167981));
#99441=CARTESIAN_POINT('Ctrl Pts',(-29.1337101377013,638.908726592018,68.875333021914));
#99442=CARTESIAN_POINT('Ctrl Pts',(-28.9858011108829,638.875563148338,68.9954353966035));
#99443=CARTESIAN_POINT('Ctrl Pts',(-28.8324181716989,638.84335373522,69.1075648843374));
#99444=CARTESIAN_POINT('Ctrl Pts',(-28.6733382516838,638.812589007746,69.2117599847112));
#99445=CARTESIAN_POINT('Ctrl Pts',(-28.6310104190001,638.804403158539,69.2394841171767));
#99446=CARTESIAN_POINT('Ctrl Pts',(-28.5882790861707,638.796319628859,69.2666462816184));
#99447=CARTESIAN_POINT('Ctrl Pts',(-28.5451396868815,638.788347763513,69.2932467040797));
#99448=CARTESIAN_POINT('Ctrl Pts',(-28.4250134433244,638.766149256951,69.3673184083678));
#99449=CARTESIAN_POINT('Ctrl Pts',(-28.3017294042537,638.744824138075,69.4370253915424));
#99450=CARTESIAN_POINT('Ctrl Pts',(-28.1753668997168,638.72460142226,69.5022880910652));
#99451=CARTESIAN_POINT('Ctrl Pts',(-28.1463954434268,638.719964908213,69.5172510379736));
#99452=CARTESIAN_POINT('Ctrl Pts',(-28.1172369493377,638.715384248088,69.5319854519995));
#99453=CARTESIAN_POINT('Ctrl Pts',(-28.0879158996004,638.710864993133,69.54648058979));
#99454=CARTESIAN_POINT('Ctrl Pts',(-27.9760916405646,638.693629514143,69.6017619681025));
#99455=CARTESIAN_POINT('Ctrl Pts',(-27.861674530411,638.677255876872,69.6536712213467));
#99456=CARTESIAN_POINT('Ctrl Pts',(-27.7460960223066,638.662070518278,69.7015521321279));
#99457=CARTESIAN_POINT('Ctrl Pts',(-27.7129974149808,638.657721835902,69.7152639500977));
#99458=CARTESIAN_POINT('Ctrl Pts',(-27.6798037327096,638.653470532345,69.7286456758798));
#99459=CARTESIAN_POINT('Ctrl Pts',(-27.6465488703812,638.649324069762,69.7416826110321));
#99460=CARTESIAN_POINT('Ctrl Pts',(-27.6326745277465,638.647594113943,69.7471217827063));
#99461=CARTESIAN_POINT('Ctrl Pts',(-27.6187849721134,638.645881515037,69.7525038695469));
#99462=CARTESIAN_POINT('Ctrl Pts',(-27.6048805343477,638.644186425559,69.7578289051375));
#99463=CARTESIAN_POINT('Ctrl Pts',(-27.4384561734201,638.623897638069,69.8215650777181));
#99464=CARTESIAN_POINT('Ctrl Pts',(-27.2697521412095,638.606099695926,69.8771839024021));
#99465=CARTESIAN_POINT('Ctrl Pts',(-27.0988334158908,638.591005578511,69.9249015221625));
#99466=CARTESIAN_POINT('Ctrl Pts',(-26.9337006291902,638.576422426976,69.971003805637));
#99467=CARTESIAN_POINT('Ctrl Pts',(-26.7661415228627,638.564359870537,70.0098078169358));
#99468=CARTESIAN_POINT('Ctrl Pts',(-26.5966620479512,638.554998549506,70.041199579679));
#99469=CARTESIAN_POINT('Ctrl Pts',(-26.461079942878,638.547509574145,70.0663127166939));
#99470=CARTESIAN_POINT('Ctrl Pts',(-26.3239827419714,638.541734850019,70.0867314754902));
#99471=CARTESIAN_POINT('Ctrl Pts',(-26.1857776575908,638.537787923926,70.1023345303239));
#99472=CARTESIAN_POINT('Ctrl Pts',(-26.1089490305539,638.535593815699,70.1110083159942));
#99473=CARTESIAN_POINT('Ctrl Pts',(-26.0317783136576,638.533964259481,70.1181947427061));
#99474=CARTESIAN_POINT('Ctrl Pts',(-25.9543371050814,638.532916410857,70.1238793316371));
#99475=CARTESIAN_POINT('Ctrl Pts',(-25.8167125789174,638.531054228265,70.133981690219));
#99476=CARTESIAN_POINT('Ctrl Pts',(-25.6795944555712,638.531029990121,70.1392897137754));
#99477=CARTESIAN_POINT('Ctrl Pts',(-25.5431350324273,638.532774282377,70.139953710851));
#99478=CARTESIAN_POINT('Ctrl Pts',(-25.2914954588901,638.535990864635,70.1411781623186));
#99479=CARTESIAN_POINT('Ctrl Pts',(-25.0415283182023,638.54522420148,70.1266264453647));
#99480=CARTESIAN_POINT('Ctrl Pts',(-24.7931436546858,638.560084548181,70.0971649802425));
#99481=CARTESIAN_POINT('Ctrl Pts',(-24.6947005333332,638.565974198906,70.0854884195998));
#99482=CARTESIAN_POINT('Ctrl Pts',(-24.5965076945556,638.57274775555,70.0714505616851));
#99483=CARTESIAN_POINT('Ctrl Pts',(-24.4985645019917,638.580380570782,70.0550492251778));
#99484=CARTESIAN_POINT('Ctrl Pts',(-24.4055700369588,638.587627726511,70.0394765909354));
#99485=CARTESIAN_POINT('Ctrl Pts',(-24.3128009675369,638.595649471429,70.0217733564026));
#99486=CARTESIAN_POINT('Ctrl Pts',(-24.2202555268896,638.604424965257,70.0019373245855));
#99487=CARTESIAN_POINT('Ctrl Pts',(-24.0300461694498,638.622461305359,69.961168175509));
#99488=CARTESIAN_POINT('Ctrl Pts',(-23.8399539788754,638.643812726827,69.9110564175541));
#99489=CARTESIAN_POINT('Ctrl Pts',(-23.6547230176572,638.667611720096,69.8530085660251));
#99490=CARTESIAN_POINT('Ctrl Pts',(-23.5956647900816,638.675199686769,69.83450084354));
#99491=CARTESIAN_POINT('Ctrl Pts',(-23.5370157634051,638.683040624755,69.815183697452));
#99492=CARTESIAN_POINT('Ctrl Pts',(-23.4787716692218,638.691121070468,69.7950618652513));
#99493=CARTESIAN_POINT('Ctrl Pts',(-23.2954816375586,638.716549659775,69.7317398870677));
#99494=CARTESIAN_POINT('Ctrl Pts',(-23.1161090862269,638.744363790947,69.6604122975168));
#99495=CARTESIAN_POINT('Ctrl Pts',(-22.9406726614924,638.77412321845,69.5812766910076));
#99496=CARTESIAN_POINT('Ctrl Pts',(-22.8217503042241,638.794296117407,69.5276333675976));
#99497=CARTESIAN_POINT('Ctrl Pts',(-22.7046361153286,638.81536258406,69.4704032346877));
#99498=CARTESIAN_POINT('Ctrl Pts',(-22.5893301219767,638.837183127349,69.4096598760731));
#99499=CARTESIAN_POINT('Ctrl Pts',(-22.5686659162834,638.841093628284,69.398773943604));
#99500=CARTESIAN_POINT('Ctrl Pts',(-22.5480499464903,638.845031127836,69.3877658954824));
#99501=CARTESIAN_POINT('Ctrl Pts',(-22.5274854821768,638.848994107946,69.3766377974433));
#99502=CARTESIAN_POINT('Ctrl Pts',(-22.367532149233,638.879818731788,69.2900818656407));
#99503=CARTESIAN_POINT('Ctrl Pts',(-22.210359426731,638.912253152739,69.1960767963424));
#99504=CARTESIAN_POINT('Ctrl Pts',(-22.0575602488078,638.945591200531,69.0955440329588));
#99505=CARTESIAN_POINT('Ctrl Pts',(-21.9193885106254,638.975737802585,69.0046352541957));
#99506=CARTESIAN_POINT('Ctrl Pts',(-21.7847938371326,639.006622687079,68.9083899705106));
#99507=CARTESIAN_POINT('Ctrl Pts',(-21.6549354488148,639.037718739692,68.8075207260076));
#99508=CARTESIAN_POINT('Ctrl Pts',(-21.643287802225,639.040507899759,68.7984732603261));
#99509=CARTESIAN_POINT('Ctrl Pts',(-21.6316772250658,639.043298999767,68.7893878199803));
#99510=CARTESIAN_POINT('Ctrl Pts',(-21.6201045092409,639.046091673901,68.7802648661229));
#99511=CARTESIAN_POINT('Ctrl Pts',(-21.3855062639945,639.102703834884,68.5953273805063));
#99512=CARTESIAN_POINT('Ctrl Pts',(-21.1653101456083,639.160101323533,68.3948305812084));
#99513=CARTESIAN_POINT('Ctrl Pts',(-20.9599503527233,639.216574790309,68.1780943251773));
#99514=CARTESIAN_POINT('Ctrl Pts',(-20.9375987588717,639.222721426781,68.1545045041142));
#99515=CARTESIAN_POINT('Ctrl Pts',(-20.9154228865181,639.228857107169,68.1307223393094));
#99516=CARTESIAN_POINT('Ctrl Pts',(-20.8934232692971,639.234979621408,68.1067469800065));
#99517=CARTESIAN_POINT('Ctrl Pts',(-20.8578334961279,639.244884288876,68.0679609597466));
#99518=CARTESIAN_POINT('Ctrl Pts',(-20.8227033851914,639.254754601208,68.0286675090153));
#99519=CARTESIAN_POINT('Ctrl Pts',(-20.7880346630825,639.264581421708,67.9888621558238));
#99520=CARTESIAN_POINT('Ctrl Pts',(-20.6616762743501,639.300397602092,67.8437820955777));
#99521=CARTESIAN_POINT('Ctrl Pts',(-20.5410984570128,639.335762387801,67.6911801290186));
#99522=CARTESIAN_POINT('Ctrl Pts',(-20.4291183567793,639.369452958869,67.534187278599));
#99523=CARTESIAN_POINT('Ctrl Pts',(-20.3697325502214,639.387319898906,67.4509301014172));
#99524=CARTESIAN_POINT('Ctrl Pts',(-20.3126235691871,639.40475389604,67.366306414107));
#99525=CARTESIAN_POINT('Ctrl Pts',(-20.2578038594729,639.421695203221,67.2802970661521));
#99526=CARTESIAN_POINT('Ctrl Pts',(-20.2093649909189,639.436664595726,67.2042989347917));
#99527=CARTESIAN_POINT('Ctrl Pts',(-20.1627111642279,639.451249581901,67.1272149272915));
#99528=CARTESIAN_POINT('Ctrl Pts',(-20.1178555439554,639.465407366224,67.0490382112228));
#99529=CARTESIAN_POINT('Ctrl Pts',(-20.0223407470047,639.495554712012,66.8825700380885));
#99530=CARTESIAN_POINT('Ctrl Pts',(-19.9349790005985,639.523766588609,66.7111477600417));
#99531=CARTESIAN_POINT('Ctrl Pts',(-19.8561484137327,639.549609228609,66.5345618643413));
#99532=CARTESIAN_POINT('Ctrl Pts',(-19.8294237927332,639.558370228458,66.4746968890304));
#99533=CARTESIAN_POINT('Ctrl Pts',(-19.8036481144562,639.566869796379,66.414120338036));
#99534=CARTESIAN_POINT('Ctrl Pts',(-19.7789014749039,639.575070818021,66.3530062062367));
#99535=CARTESIAN_POINT('Ctrl Pts',(-19.7307143056419,639.591040017278,66.2340035025727));
#99536=CARTESIAN_POINT('Ctrl Pts',(-19.6864044881282,639.605878387103,66.1128942179124));
#99537=CARTESIAN_POINT('Ctrl Pts',(-19.646591826502,639.619305133542,65.9910272445652));
#99538=CARTESIAN_POINT('Ctrl Pts',(-19.5982725234243,639.635600729064,65.8431213528264));
#99539=CARTESIAN_POINT('Ctrl Pts',(-19.5563270690099,639.64988432506,65.6938288756537));
#99540=CARTESIAN_POINT('Ctrl Pts',(-19.5208462578372,639.662045684834,65.5432736384627));
#99541=CARTESIAN_POINT('Ctrl Pts',(-19.505465144989,639.667317696405,65.4780071742364));
#99542=CARTESIAN_POINT('Ctrl Pts',(-19.4912982950981,639.672191081517,65.4125035254526));
#99543=CARTESIAN_POINT('Ctrl Pts',(-19.4783502595523,639.676657814842,65.3467733418589));
#99544=CARTESIAN_POINT('Ctrl Pts',(-19.460100437904,639.682953525589,65.2541288535699));
#99545=CARTESIAN_POINT('Ctrl Pts',(-19.4443099666198,639.688427265665,65.1612494229568));
#99546=CARTESIAN_POINT('Ctrl Pts',(-19.4309280055641,639.693076648407,65.0679022967298));
#99547=CARTESIAN_POINT('Ctrl Pts',(-19.420981995495,639.696532256099,64.9985229693267));
#99548=CARTESIAN_POINT('Ctrl Pts',(-19.4123674445347,639.699532175518,64.9288850734574));
#99549=CARTESIAN_POINT('Ctrl Pts',(-19.4050808070072,639.702069575624,64.8588893165577));
#99550=CARTESIAN_POINT('Ctrl Pts',(-19.3955152473809,639.70540055674,64.767002134893));
#99551=CARTESIAN_POINT('Ctrl Pts',(-19.3882670280903,639.707928940124,64.6741951541139));
#99552=CARTESIAN_POINT('Ctrl Pts',(-19.3833968487432,639.709628527129,64.5808344913998));
#99553=CARTESIAN_POINT('Ctrl Pts',(-19.3787769857904,639.711240759139,64.4922723592536));
#99554=CARTESIAN_POINT('Ctrl Pts',(-19.3762971925334,639.71210714373,64.4032105488006));
#99555=CARTESIAN_POINT('Ctrl Pts',(-19.3760492768828,639.712191230638,64.3139797755864));
#99556=CARTESIAN_POINT('Ctrl Pts',(-19.3760358441571,639.712195786689,64.3091450162767));
#99557=CARTESIAN_POINT('Ctrl Pts',(-19.3760289735364,639.712198042607,64.3043097686405));
#99558=CARTESIAN_POINT('Ctrl Pts',(-19.3760286830353,639.712197991384,64.2994740881603));
#99559=CARTESIAN_POINT('',(-31.4841643694399,640.028384824678,66.2394387527688));
#99560=CARTESIAN_POINT('Origin',(-31.4841643694399,639.530878113616,66.1895681958392));
#99561=CARTESIAN_POINT('',(-19.1902534503917,640.029230307342,62.3679625261942));
#99562=CARTESIAN_POINT('Ctrl Pts',(-19.1902534503917,640.029230307342,62.3679625261942));
#99563=CARTESIAN_POINT('Ctrl Pts',(-19.0661541944461,640.067381465102,62.7502393133262));
#99564=CARTESIAN_POINT('Ctrl Pts',(-18.9797925330106,640.094758237498,63.1390436335595));
#99565=CARTESIAN_POINT('Ctrl Pts',(-18.9308583517509,640.110319951076,63.5343769526662));
#99566=CARTESIAN_POINT('Ctrl Pts',(-18.9275335472574,640.111377282656,63.5612376451706));
#99567=CARTESIAN_POINT('Ctrl Pts',(-18.9243815405164,640.112380060573,63.5881284854448));
#99568=CARTESIAN_POINT('Ctrl Pts',(-18.9214022412361,640.113327953849,63.615049477024));
#99569=CARTESIAN_POINT('Ctrl Pts',(-18.9209816912288,640.113461755957,63.6188495729999));
#99570=CARTESIAN_POINT('Ctrl Pts',(-18.920564586754,640.113594463482,63.6226502418285));
#99571=CARTESIAN_POINT('Ctrl Pts',(-18.9201509276431,640.113726075471,63.6264514814598));
#99572=CARTESIAN_POINT('Ctrl Pts',(-18.902553802402,640.119324870691,63.7881568279721));
#99573=CARTESIAN_POINT('Ctrl Pts',(-18.8912383129095,640.122939359055,63.9509059522893));
#99574=CARTESIAN_POINT('Ctrl Pts',(-18.8863728855358,640.12449505208,64.1145722906471));
#99575=CARTESIAN_POINT('Ctrl Pts',(-18.8848185279603,640.124992049168,64.1668587586874));
#99576=CARTESIAN_POINT('Ctrl Pts',(-18.8839220986039,640.125279042398,64.219238776882));
#99577=CARTESIAN_POINT('Ctrl Pts',(-18.8836880253474,640.125353945508,64.2717080420946));
#99578=CARTESIAN_POINT('Ctrl Pts',(-18.88301708418,640.125568645732,64.4221045058983));
#99579=CARTESIAN_POINT('Ctrl Pts',(-18.8878933700143,640.124007040391,64.5733859358451));
#99580=CARTESIAN_POINT('Ctrl Pts',(-18.8981256828954,640.120744141073,64.7234029230822));
#99581=CARTESIAN_POINT('Ctrl Pts',(-18.9021353453646,640.119465532308,64.7821889952511));
#99582=CARTESIAN_POINT('Ctrl Pts',(-18.906967113598,640.117925787138,64.8407812737556));
#99583=CARTESIAN_POINT('Ctrl Pts',(-18.9126081755515,640.116129824278,64.8990522739188));
#99584=CARTESIAN_POINT('Ctrl Pts',(-18.9133750559051,640.115885670138,64.9069739889396));
#99585=CARTESIAN_POINT('Ctrl Pts',(-18.9141569982845,640.115636744668,64.9148909499626));
#99586=CARTESIAN_POINT('Ctrl Pts',(-18.9149539843053,640.115383055814,64.9228028479913));
#99587=CARTESIAN_POINT('Ctrl Pts',(-18.9390529021059,640.107712122208,65.1620393907661));
#99588=CARTESIAN_POINT('Ctrl Pts',(-18.9767296895114,640.095716478747,65.3984843576705));
#99589=CARTESIAN_POINT('Ctrl Pts',(-19.0278441371165,640.0796734569,65.6320777987911));
#99590=CARTESIAN_POINT('Ctrl Pts',(-19.0657431118152,640.067778305773,65.8052764212864));
#99591=CARTESIAN_POINT('Ctrl Pts',(-19.1110284495377,640.053658493531,65.9769076528193));
#99592=CARTESIAN_POINT('Ctrl Pts',(-19.1636259297164,640.037432831445,66.1469510602767));
#99593=CARTESIAN_POINT('Ctrl Pts',(-19.1674780851709,640.036244489865,66.1594047678937));
#99594=CARTESIAN_POINT('Ctrl Pts',(-19.1713696911087,640.035044796896,66.1718505666322));
#99595=CARTESIAN_POINT('Ctrl Pts',(-19.1753007143207,640.033833800824,66.1842884067607));
#99596=CARTESIAN_POINT('Ctrl Pts',(-19.2285496458958,640.017429866411,66.3527691463099));
#99597=CARTESIAN_POINT('Ctrl Pts',(-19.289319827394,639.998881530564,66.5201053281933));
#99598=CARTESIAN_POINT('Ctrl Pts',(-19.3563790031072,639.978718302077,66.6834337378297));
#99599=CARTESIAN_POINT('Ctrl Pts',(-19.3652569531254,639.976048896544,66.7050567512635));
#99600=CARTESIAN_POINT('Ctrl Pts',(-19.3742450600393,639.97335120706,66.7266095305223));
#99601=CARTESIAN_POINT('Ctrl Pts',(-19.3833404036078,639.970626479297,66.7480854497941));
#99602=CARTESIAN_POINT('Ctrl Pts',(-19.389259711703,639.968853208943,66.7620621161881));
#99603=CARTESIAN_POINT('Ctrl Pts',(-19.3952253226528,639.967068178453,66.7760086572856));
#99604=CARTESIAN_POINT('Ctrl Pts',(-19.4012364653116,639.965271726116,66.7899231687001));
#99605=CARTESIAN_POINT('Ctrl Pts',(-19.4648946971272,639.94624722681,66.9372783794339));
#99606=CARTESIAN_POINT('Ctrl Pts',(-19.5338281275451,639.925888517147,67.0816821104859));
#99607=CARTESIAN_POINT('Ctrl Pts',(-19.6078620284061,639.904390307426,67.2230749934025));
#99608=CARTESIAN_POINT('Ctrl Pts',(-19.6247075204097,639.899498657578,67.2552471827756));
#99609=CARTESIAN_POINT('Ctrl Pts',(-19.6418168977857,639.894548065483,67.2872635875361));
#99610=CARTESIAN_POINT('Ctrl Pts',(-19.6591877821883,639.889540914653,67.3191236770128));
#99611=CARTESIAN_POINT('Ctrl Pts',(-19.6672132267431,639.887227583309,67.3338432143535));
#99612=CARTESIAN_POINT('Ctrl Pts',(-19.6752948262461,639.884902074872,67.3485300567643));
#99613=CARTESIAN_POINT('Ctrl Pts',(-19.6834324285052,639.882564594915,67.3631843223957));
#99614=CARTESIAN_POINT('Ctrl Pts',(-19.7776280083814,639.855507450449,67.5328125500803));
#99615=CARTESIAN_POINT('Ctrl Pts',(-19.8793287143073,639.826844553833,67.6980744824025));
#99616=CARTESIAN_POINT('Ctrl Pts',(-19.9885164512294,639.796882111454,67.8590274942721));
#99617=CARTESIAN_POINT('Ctrl Pts',(-19.998657149862,639.794099380472,67.8739758395112));
#99618=CARTESIAN_POINT('Ctrl Pts',(-20.0088629640138,639.791305313846,67.8888877085587));
#99619=CARTESIAN_POINT('Ctrl Pts',(-20.0191337952575,639.788500187125,67.9037629706155));
#99620=CARTESIAN_POINT('Ctrl Pts',(-20.1143609759211,639.762492135519,68.0416806555319));
#99621=CARTESIAN_POINT('Ctrl Pts',(-20.2155196510365,639.735450423221,68.1767756433179));
#99622=CARTESIAN_POINT('Ctrl Pts',(-20.3210516911105,639.707998172089,68.3071685062823));
#99623=CARTESIAN_POINT('Ctrl Pts',(-20.3372811768278,639.703776364974,68.3272212704061));
#99624=CARTESIAN_POINT('Ctrl Pts',(-20.3536140016895,639.69954486717,68.3471628573523));
#99625=CARTESIAN_POINT('Ctrl Pts',(-20.3700444059045,639.695305961865,68.3669864753928));
#99626=CARTESIAN_POINT('Ctrl Pts',(-20.3820839732001,639.692199855343,68.3815124590702));
#99627=CARTESIAN_POINT('Ctrl Pts',(-20.3941775547018,639.689089316829,68.3959772275318));
#99628=CARTESIAN_POINT('Ctrl Pts',(-20.4063230234607,639.685975213723,68.4103781892567));
#99629=CARTESIAN_POINT('Ctrl Pts',(-20.5574363591296,639.647229693296,68.5895542594672));
#99630=CARTESIAN_POINT('Ctrl Pts',(-20.717043795479,639.607778714808,68.7598361525156));
#99631=CARTESIAN_POINT('Ctrl Pts',(-20.8850330097057,639.568267584666,68.9213365607569));
#99632=CARTESIAN_POINT('Ctrl Pts',(-21.0058686124506,639.539847002738,69.0375047282385));
#99633=CARTESIAN_POINT('Ctrl Pts',(-21.1310402565699,639.511395652052,69.1491302172699));
#99634=CARTESIAN_POINT('Ctrl Pts',(-21.2604957797351,639.483157142327,69.2562674885842));
#99635=CARTESIAN_POINT('Ctrl Pts',(-21.2750353916501,639.479985574499,69.2683004579659));
#99636=CARTESIAN_POINT('Ctrl Pts',(-21.289629990286,639.476816511724,69.2802775120789));
#99637=CARTESIAN_POINT('Ctrl Pts',(-21.3042794741003,639.4736503114,69.2921986802951));
#99638=CARTESIAN_POINT('Ctrl Pts',(-21.4607808919954,639.43982558103,69.4195533197106));
#99639=CARTESIAN_POINT('Ctrl Pts',(-21.6240297334742,639.406279563647,69.5405878515707));
#99640=CARTESIAN_POINT('Ctrl Pts',(-21.7923110743027,639.373756834287,69.6541564729845));
#99641=CARTESIAN_POINT('Ctrl Pts',(-21.9591823739661,639.341506615159,69.766773494949));
#99642=CARTESIAN_POINT('Ctrl Pts',(-22.1310007280687,639.310263231699,69.8720483495535));
#99643=CARTESIAN_POINT('Ctrl Pts',(-22.3060525550972,639.280754274564,69.9688928418353));
#99644=CARTESIAN_POINT('Ctrl Pts',(-22.3209841823156,639.278237210018,69.9771535145827));
#99645=CARTESIAN_POINT('Ctrl Pts',(-22.3359409831016,639.275732443914,69.9853539171062));
#99646=CARTESIAN_POINT('Ctrl Pts',(-22.3509219295449,639.273240430825,69.9934933567789));
#99647=CARTESIAN_POINT('Ctrl Pts',(-22.5575543226994,639.238868061217,70.1057607562306));
#99648=CARTESIAN_POINT('Ctrl Pts',(-22.7696906147764,639.206689097186,70.207314951391));
#99649=CARTESIAN_POINT('Ctrl Pts',(-22.9874368158415,639.177355225063,70.2977872106618));
#99650=CARTESIAN_POINT('Ctrl Pts',(-23.1430911565897,639.156386112837,70.3624606690456));
#99651=CARTESIAN_POINT('Ctrl Pts',(-23.3016117153739,639.136870942413,70.4214721408255));
#99652=CARTESIAN_POINT('Ctrl Pts',(-23.4630294903487,639.119046867783,70.4747013867516));
#99653=CARTESIAN_POINT('Ctrl Pts',(-23.4760929938243,639.117604369514,70.4790092174058));
#99654=CARTESIAN_POINT('Ctrl Pts',(-23.4891763555709,639.11617285942,70.4832794429651));
#99655=CARTESIAN_POINT('Ctrl Pts',(-23.5022794848633,639.114752478456,70.4875119546639));
#99656=CARTESIAN_POINT('Ctrl Pts',(-23.6447432912411,639.099309382824,70.5335299488156));
#99657=CARTESIAN_POINT('Ctrl Pts',(-23.7900031744777,639.085168169529,70.5751004640745));
#99658=CARTESIAN_POINT('Ctrl Pts',(-23.9360313149344,639.072643530069,70.6116036338563));
#99659=CARTESIAN_POINT('Ctrl Pts',(-23.984047368707,639.068525256975,70.6236063763252));
#99660=CARTESIAN_POINT('Ctrl Pts',(-24.0321462796011,639.064581660107,70.6350616021584));
#99661=CARTESIAN_POINT('Ctrl Pts',(-24.0802556359924,639.060823572796,70.6459484087714));
#99662=CARTESIAN_POINT('Ctrl Pts',(-24.0914495259928,639.059949156277,70.6484815067969));
#99663=CARTESIAN_POINT('Ctrl Pts',(-24.1026450649215,639.059084673775,70.6509841478699));
#99664=CARTESIAN_POINT('Ctrl Pts',(-24.1138413856779,639.05823026425,70.6534560603949));
#99665=CARTESIAN_POINT('Ctrl Pts',(-24.2901636767411,639.044774822211,70.6923843198837));
#99666=CARTESIAN_POINT('Ctrl Pts',(-24.4673393093431,639.033728544892,70.7239610465782));
#99667=CARTESIAN_POINT('Ctrl Pts',(-24.6452243354155,639.025223969683,70.7481570845842));
#99668=CARTESIAN_POINT('Ctrl Pts',(-24.6658100213957,639.024239780521,70.7509571631032));
#99669=CARTESIAN_POINT('Ctrl Pts',(-24.6864051962316,639.0232896132,70.7536584516014));
#99670=CARTESIAN_POINT('Ctrl Pts',(-24.7070096277252,639.022373659332,70.7562609470984));
#99671=CARTESIAN_POINT('Ctrl Pts',(-24.7158860784374,639.021979063666,70.7573821099421));
#99672=CARTESIAN_POINT('Ctrl Pts',(-24.7247643877193,639.021590806335,70.7584849700153));
#99673=CARTESIAN_POINT('Ctrl Pts',(-24.7336445558265,639.021208901519,70.7595695302754));
#99674=CARTESIAN_POINT('Ctrl Pts',(-25.1448548055267,639.003524194108,70.8097918109785));
#99675=CARTESIAN_POINT('Ctrl Pts',(-25.5600221154403,638.999460434065,70.8210939230077));
#99676=CARTESIAN_POINT('Ctrl Pts',(-25.9794873808982,639.010400866811,70.7901814866191));
#99677=CARTESIAN_POINT('Ctrl Pts',(-25.9832750388911,639.010499655962,70.7899023556722));
#99678=CARTESIAN_POINT('Ctrl Pts',(-25.9870629997303,639.010599667727,70.7896197849193));
#99679=CARTESIAN_POINT('Ctrl Pts',(-25.9908512633906,639.010700903034,70.7893337721921));
#99680=CARTESIAN_POINT('Ctrl Pts',(-26.2663020200481,639.018061885379,70.7685373257971));
#99681=CARTESIAN_POINT('Ctrl Pts',(-26.5383229063629,639.03182351378,70.7297246005164));
#99682=CARTESIAN_POINT('Ctrl Pts',(-26.8052344292236,639.051326252545,70.6734607796385));
#99683=CARTESIAN_POINT('Ctrl Pts',(-26.9487943211451,639.061815912336,70.6431989611986));
#99684=CARTESIAN_POINT('Ctrl Pts',(-27.0908765464588,639.073966216304,70.6078894896557));
#99685=CARTESIAN_POINT('Ctrl Pts',(-27.2312233323724,639.087673452015,70.56762534775));
#99686=CARTESIAN_POINT('Ctrl Pts',(-27.2323605203673,639.087784517643,70.5672990994608));
#99687=CARTESIAN_POINT('Ctrl Pts',(-27.2334976101377,639.087895685839,70.5669725224296));
#99688=CARTESIAN_POINT('Ctrl Pts',(-27.2346346016704,639.08800695655,70.5666456166163));
#99689=CARTESIAN_POINT('Ctrl Pts',(-27.4345340242248,639.107569943678,70.5091708848989));
#99690=CARTESIAN_POINT('Ctrl Pts',(-27.6314474761934,639.130308814554,70.4415110705284));
#99691=CARTESIAN_POINT('Ctrl Pts',(-27.8252672673916,639.15591603875,70.3634708926868));
#99692=CARTESIAN_POINT('Ctrl Pts',(-27.8282445068165,639.156309387835,70.3622721281398));
#99693=CARTESIAN_POINT('Ctrl Pts',(-27.8312212104409,639.156703452167,70.3610707873401));
#99694=CARTESIAN_POINT('Ctrl Pts',(-27.834197359946,639.157098227311,70.3598668790042));
#99695=CARTESIAN_POINT('Ctrl Pts',(-27.9894491330569,639.177691796646,70.2970646227717));
#99696=CARTESIAN_POINT('Ctrl Pts',(-28.1432703577507,639.20023292809,70.2272339023149));
#99697=CARTESIAN_POINT('Ctrl Pts',(-28.2929815772957,639.224084541252,70.1516373994087));
#99698=CARTESIAN_POINT('Ctrl Pts',(-28.3285967893406,639.229758666832,70.1336535402895));
#99699=CARTESIAN_POINT('Ctrl Pts',(-28.3639795834936,639.235506933618,70.1153435164027));
#99700=CARTESIAN_POINT('Ctrl Pts',(-28.3990942913099,639.241320738419,70.096724553437));
#99701=CARTESIAN_POINT('Ctrl Pts',(-28.4034106922287,639.242035388033,70.0944358569377));
#99702=CARTESIAN_POINT('Ctrl Pts',(-28.4077235599911,639.242751075026,70.0921423887562));
#99703=CARTESIAN_POINT('Ctrl Pts',(-28.4120328939071,639.243467791937,70.0898441520015));
#99704=CARTESIAN_POINT('Ctrl Pts',(-28.658158288822,639.284402710433,69.9585815392916));
#99705=CARTESIAN_POINT('Ctrl Pts',(-28.8929149867157,639.328720256045,69.8116819089959));
#99706=CARTESIAN_POINT('Ctrl Pts',(-29.116618808618,639.375128618273,69.6494399515747));
#99707=CARTESIAN_POINT('Ctrl Pts',(-29.2269895260826,639.398025519149,69.5693932134762));
#99708=CARTESIAN_POINT('Ctrl Pts',(-29.334670118163,639.421431631444,69.4856124469673));
#99709=CARTESIAN_POINT('Ctrl Pts',(-29.4397007152155,639.44519366648,69.3981367404782));
#99710=CARTESIAN_POINT('Ctrl Pts',(-29.4448089218575,639.446349342908,69.3938823232185));
#99711=CARTESIAN_POINT('Ctrl Pts',(-29.4499116020077,639.447506069964,69.3896182581848));
#99712=CARTESIAN_POINT('Ctrl Pts',(-29.4550086592013,639.448663806067,69.3853446352532));
#99713=CARTESIAN_POINT('Ctrl Pts',(-29.5908506819648,639.47951871078,69.2714480157898));
#99714=CARTESIAN_POINT('Ctrl Pts',(-29.7228031442344,639.511116227394,69.1506637347806));
#99715=CARTESIAN_POINT('Ctrl Pts',(-29.8489633040033,639.54265629442,69.0247387156344));
#99716=CARTESIAN_POINT('Ctrl Pts',(-29.8676605002224,639.547330597488,69.0060763677411));
#99717=CARTESIAN_POINT('Ctrl Pts',(-29.8862305633637,639.55200365133,68.9873011389271));
#99718=CARTESIAN_POINT('Ctrl Pts',(-29.9046673995305,639.55667286808,68.9684187394493));
#99719=CARTESIAN_POINT('Ctrl Pts',(-29.9094138856866,639.557874938352,68.9635575448873));
#99720=CARTESIAN_POINT('Ctrl Pts',(-29.9141513180268,639.559076664587,68.9586896901739));
#99721=CARTESIAN_POINT('Ctrl Pts',(-29.9188797057288,639.560278028195,68.953815187973));
#99722=CARTESIAN_POINT('Ctrl Pts',(-30.0614635141599,639.596504964179,68.8068253191634));
#99723=CARTESIAN_POINT('Ctrl Pts',(-30.195875970295,639.632413788924,68.6537419339198));
#99724=CARTESIAN_POINT('Ctrl Pts',(-30.3224858870252,639.667536294259,68.4947407588566));
#99725=CARTESIAN_POINT('Ctrl Pts',(-30.3264285834488,639.668630026722,68.4897893823731));
#99726=CARTESIAN_POINT('Ctrl Pts',(-30.3303637706444,639.669723000392,68.4848323127038));
#99727=CARTESIAN_POINT('Ctrl Pts',(-30.3342914487826,639.670815201699,68.4798695468125));
#99728=CARTESIAN_POINT('Ctrl Pts',(-30.4782769420951,639.710854415335,68.2979385764189));
#99729=CARTESIAN_POINT('Ctrl Pts',(-30.6121413968524,639.749841074717,68.1084191608539));
#99730=CARTESIAN_POINT('Ctrl Pts',(-30.7359639883784,639.787131213705,67.9110767494707));
#99731=CARTESIAN_POINT('Ctrl Pts',(-30.8337001870814,639.816565232077,67.7553095595437));
#99732=CARTESIAN_POINT('Ctrl Pts',(-30.9251791288008,639.844942498338,67.5946678504991));
#99733=CARTESIAN_POINT('Ctrl Pts',(-31.0104208812647,639.871946950842,67.4290232404352));
#99734=CARTESIAN_POINT('Ctrl Pts',(-31.0122763604105,639.872534763704,67.4254176116124));
#99735=CARTESIAN_POINT('Ctrl Pts',(-31.0141283326744,639.87312174693,67.421810661113));
#99736=CARTESIAN_POINT('Ctrl Pts',(-31.0159767997225,639.873707898436,67.4182023901961));
#99737=CARTESIAN_POINT('Ctrl Pts',(-31.1033885579826,639.901426290174,67.2475716475735));
#99738=CARTESIAN_POINT('Ctrl Pts',(-31.1828892592656,639.927259372726,67.0741503956703));
#99739=CARTESIAN_POINT('Ctrl Pts',(-31.2547101808772,639.95100397125,66.8980122231744));
#99740=CARTESIAN_POINT('Ctrl Pts',(-31.3273357480885,639.975014592351,66.7199006868974));
#99741=CARTESIAN_POINT('Ctrl Pts',(-31.3921084363252,639.996889925891,66.5390108510075));
#99742=CARTESIAN_POINT('Ctrl Pts',(-31.4492188957602,640.016409086981,66.3553999762133));
#99743=CARTESIAN_POINT('Ctrl Pts',(-31.4612045326073,640.020505527085,66.3168659968294));
#99744=CARTESIAN_POINT('Ctrl Pts',(-31.4728525242766,640.024498145574,66.2782121103769));
#99745=CARTESIAN_POINT('Ctrl Pts',(-31.4841643694399,640.028384824678,66.2394387527688));
#99746=CARTESIAN_POINT('',(-19.6604693917099,639.614613618721,62.5660159449655));
#99747=CARTESIAN_POINT('Origin',(-19.1902534503917,639.531701861507,62.4176157797164));
#99748=CARTESIAN_POINT('Ctrl Pts',(-19.376027899398,639.712197853207,64.2994740882088));
#99749=CARTESIAN_POINT('Ctrl Pts',(-19.376027899398,639.712197853207,64.0018698655157));
#99750=CARTESIAN_POINT('Ctrl Pts',(-19.4004974737455,639.703610742277,63.7087642394116));
#99751=CARTESIAN_POINT('Ctrl Pts',(-19.4956764044269,639.670658245073,63.1310286597025));
#99752=CARTESIAN_POINT('Ctrl Pts',(-19.5663951239896,639.646286994885,62.8464005726073));
#99753=CARTESIAN_POINT('Ctrl Pts',(-19.6604693917099,639.614613618721,62.5660159449655));
#99754=CARTESIAN_POINT('Ctrl Pts',(-2.24785136021961,606.490049520156,76.3728616211989));
#99755=CARTESIAN_POINT('Ctrl Pts',(-2.07645831249209,605.414627084222,76.4046723372956));
#99756=CARTESIAN_POINT('Ctrl Pts',(-2.33937824014887,606.115760787361,77.1959965376399));
#99757=CARTESIAN_POINT('Ctrl Pts',(-1.40572798238319,606.634621533619,76.5295902130151));
#99758=CARTESIAN_POINT('Ctrl Pts',(-1.2654170129743,605.520243681078,76.5426302087965));
#99759=CARTESIAN_POINT('Ctrl Pts',(-1.46297067363917,606.264147629094,77.3634086157539));
#99760=CARTESIAN_POINT('Ctrl Pts',(-0.558874392673838,606.700257805871,
76.5971497221964));
#99761=CARTESIAN_POINT('Ctrl Pts',(-0.514725151067144,605.560838546424,
76.5942633105063));
#99762=CARTESIAN_POINT('Ctrl Pts',(-0.581630402706062,606.331517016794,
77.4355745853251));
#99763=CARTESIAN_POINT('Ctrl Pts',(0.706100277663303,606.671595580696,76.5669850049637));
#99764=CARTESIAN_POINT('Ctrl Pts',(0.646113299414241,605.541339525764,76.5691293178837));
#99765=CARTESIAN_POINT('Ctrl Pts',(0.734851049714794,606.302098310751,77.4033535057652));
#99766=CARTESIAN_POINT('Ctrl Pts',(1.12182523736722,606.642185791387,76.5361105303261));
#99767=CARTESIAN_POINT('Ctrl Pts',(1.0251340776358,605.521722692831,76.543880399892));
#99768=CARTESIAN_POINT('Ctrl Pts',(1.16750341452896,606.271912301717,77.3703742754705));
#99769=CARTESIAN_POINT('Ctrl Pts',(1.95026027616442,606.544314852399,76.4316729163024));
#99770=CARTESIAN_POINT('Ctrl Pts',(1.79327421445325,605.453614337091,76.455582544209));
#99771=CARTESIAN_POINT('Ctrl Pts',(2.0296703980175,606.171458263482,77.2588170101284));
#99772=CARTESIAN_POINT('Ctrl Pts',(2.35571831397261,606.47689240761,76.3591800393728));
#99773=CARTESIAN_POINT('Ctrl Pts',(2.1710193365545,605.406592564273,76.3944710230157));
#99774=CARTESIAN_POINT('Ctrl Pts',(2.45163778157805,606.102256333507,77.1813821711447));
#99775=CARTESIAN_POINT('Ctrl Pts',(3.15092750039858,606.310847716552,76.1762401766097));
#99776=CARTESIAN_POINT('Ctrl Pts',(2.92564597397687,605.285471359352,76.234853866594));
#99777=CARTESIAN_POINT('Ctrl Pts',(3.27922604287808,605.931829263743,76.9859709699879));
#99778=CARTESIAN_POINT('Ctrl Pts',(3.54067700376135,606.212227570323,76.0657839944311));
#99779=CARTESIAN_POINT('Ctrl Pts',(3.29897216237761,605.212582988352,76.1380212205389));
#99780=CARTESIAN_POINT('Ctrl Pts',(3.68484527501558,605.830606250497,76.8679847444035));
#99781=CARTESIAN_POINT('Ctrl Pts',(4.30578941666232,605.989162728325,75.8078458454146));
#99782=CARTESIAN_POINT('Ctrl Pts',(4.04402710457102,605.040948311733,75.904820336075));
#99783=CARTESIAN_POINT('Ctrl Pts',(4.48111132932754,605.601654146907,76.5924623214939));
#99784=CARTESIAN_POINT('Ctrl Pts',(4.68185936719368,605.864313109311,75.6597967341437));
#99785=CARTESIAN_POINT('Ctrl Pts',(4.41428255177422,604.943151687818,75.7698350030808));
#99786=CARTESIAN_POINT('Ctrl Pts',(4.87249402091235,605.473509417797,76.4343202707809));
#99787=CARTESIAN_POINT('Ctrl Pts',(5.76664965320662,605.467770079489,75.1711954372518));
#99788=CARTESIAN_POINT('Ctrl Pts',(5.47578346481391,604.628428677137,75.3217454446971));
#99789=CARTESIAN_POINT('Ctrl Pts',(6.00145504788499,605.066500484564,75.9124092474764));
#99790=CARTESIAN_POINT('Ctrl Pts',(6.44125011399598,605.172267934022,74.784314430178));
#99791=CARTESIAN_POINT('Ctrl Pts',(6.16307079581374,604.382188597855,74.9571009510351));
#99792=CARTESIAN_POINT('Ctrl Pts',(6.70352384989602,604.763199285767,75.4991529048738));
#99793=CARTESIAN_POINT('Ctrl Pts',(7.39260369019905,604.71114788997,74.1137189387619));
#99794=CARTESIAN_POINT('Ctrl Pts',(7.15897786590069,603.974427505579,74.2892807227976));
#99795=CARTESIAN_POINT('Ctrl Pts',(7.69361438062187,604.289909408297,74.7828399123804));
#99796=CARTESIAN_POINT('Ctrl Pts',(7.69999421515557,604.554074189567,73.8745480813111));
#99797=CARTESIAN_POINT('Ctrl Pts',(7.47684208610668,603.836400663942,74.0542734601015));
#99798=CARTESIAN_POINT('Ctrl Pts',(8.01352130722828,604.128690167082,74.5273634858685));
#99799=CARTESIAN_POINT('Ctrl Pts',(8.29275501798807,604.238713379567,73.3660152009349));
#99800=CARTESIAN_POINT('Ctrl Pts',(8.09137141934386,603.556059847339,73.5499197260923));
#99801=CARTESIAN_POINT('Ctrl Pts',(8.63041836958312,603.805006249089,73.9841609752444));
#99802=CARTESIAN_POINT('Ctrl Pts',(8.57500490891436,604.082124761452,73.0994134185156));
#99803=CARTESIAN_POINT('Ctrl Pts',(8.38578298933409,603.415273016501,73.2841816609331));
#99804=CARTESIAN_POINT('Ctrl Pts',(8.92416103428722,603.644284895453,73.6993832924709));
#99805=CARTESIAN_POINT('Ctrl Pts',(9.38165373201386,603.620751618402,72.2621847580793));
#99806=CARTESIAN_POINT('Ctrl Pts',(9.21438704392936,603.003986413452,72.4577134501767));
#99807=CARTESIAN_POINT('Ctrl Pts',(9.76365581150127,603.170734829699,72.8050748647865));
#99808=CARTESIAN_POINT('Ctrl Pts',(9.86648097776603,603.324313826912,71.654602795079));
#99809=CARTESIAN_POINT('Ctrl Pts',(9.72827362326639,602.72931292187,71.8438171025923));
#99810=CARTESIAN_POINT('Ctrl Pts',(10.2682245291729,602.866473387679,72.1560695767886));
#99811=CARTESIAN_POINT('Ctrl Pts',(10.5131125646575,602.91509695399,70.659537110542));
#99812=CARTESIAN_POINT('Ctrl Pts',(10.4161108402933,602.345015132654,70.8199643162105));
#99813=CARTESIAN_POINT('Ctrl Pts',(10.941186104955,602.446456401338,71.0931626340489));
#99814=CARTESIAN_POINT('Ctrl Pts',(10.7157975268766,602.784113279091,70.3120817185628));
#99815=CARTESIAN_POINT('Ctrl Pts',(10.6299402839473,602.222643594815,70.4658892792959));
#99816=CARTESIAN_POINT('Ctrl Pts',(11.1521242095173,602.312015745438,70.7220183137493));
#99817=CARTESIAN_POINT('Ctrl Pts',(11.084674691934,602.542335927575,69.6013374038105));
#99818=CARTESIAN_POINT('Ctrl Pts',(11.0180928131922,601.996679307108,69.7407948866327));
#99819=CARTESIAN_POINT('Ctrl Pts',(11.536021775298,602.063857265052,69.962816417792));
#99820=CARTESIAN_POINT('Ctrl Pts',(11.2518487421506,602.430935708244,69.2368447373392));
#99821=CARTESIAN_POINT('Ctrl Pts',(11.1947990337114,601.891830607767,69.3678350652564));
#99822=CARTESIAN_POINT('Ctrl Pts',(11.7100030252517,601.949516913845,69.5734730530018));
#99823=CARTESIAN_POINT('Ctrl Pts',(11.551217309919,602.229419141143,68.4888783550685));
#99824=CARTESIAN_POINT('Ctrl Pts',(11.5101732026518,601.702409110986,68.6025385409749));
#99825=CARTESIAN_POINT('Ctrl Pts',(12.0215617073792,601.742681788853,68.7745109630704));
#99826=CARTESIAN_POINT('Ctrl Pts',(11.6834165707129,602.139294354524,68.1054086939741));
#99827=CARTESIAN_POINT('Ctrl Pts',(11.6500527589341,601.617151454847,68.2091225258212));
#99828=CARTESIAN_POINT('Ctrl Pts',(12.1591440413972,601.650178377243,68.3648966030017));
#99829=CARTESIAN_POINT('Ctrl Pts',(11.9111236037373,601.982987992257,67.3181651639017));
#99830=CARTESIAN_POINT('Ctrl Pts',(11.890105925035,601.469623640317,67.4020108101631));
#99831=CARTESIAN_POINT('Ctrl Pts',(12.3961232041752,601.489746664308,67.5239791695796));
#99832=CARTESIAN_POINT('Ctrl Pts',(12.0069667791483,601.916568786804,66.911668961761));
#99833=CARTESIAN_POINT('Ctrl Pts',(11.9916079185944,601.406550775875,66.9841120694481));
#99834=CARTESIAN_POINT('Ctrl Pts',(12.4958690656147,601.421574482202,67.089768199197));
#99835=CARTESIAN_POINT('Ctrl Pts',(12.2299344763514,601.761466322693,65.690004883469));
#99836=CARTESIAN_POINT('Ctrl Pts',(12.2258063111644,601.260358021303,65.7350813999208));
#99837=CARTESIAN_POINT('Ctrl Pts',(12.7279159619352,601.262378414473,65.7848111091887));
#99838=CARTESIAN_POINT('Ctrl Pts',(12.2958567378873,601.714886434859,64.8673118420714));
#99839=CARTESIAN_POINT('Ctrl Pts',(12.2966228016023,601.215349916125,64.8820610902705));
#99840=CARTESIAN_POINT('Ctrl Pts',(12.7965225255397,601.214569178336,64.906027061425));
#99841=CARTESIAN_POINT('Ctrl Pts',(12.2691242107389,601.733648040287,63.6206371830607));
#99842=CARTESIAN_POINT('Ctrl Pts',(12.2684356679878,601.233129138177,63.6017923894247));
#99843=CARTESIAN_POINT('Ctrl Pts',(12.7687014560782,601.233825955092,63.5743540715745));
#99844=CARTESIAN_POINT('Ctrl Pts',(12.2386272268548,601.755068763332,63.199960706747));
#99845=CARTESIAN_POINT('Ctrl Pts',(12.2361148149086,601.253534283818,63.1686064467318));
#99846=CARTESIAN_POINT('Ctrl Pts',(12.7369626473578,601.25581202788,63.1249959000212));
#99847=CARTESIAN_POINT('Ctrl Pts',(12.1360150250495,601.826793186119,62.3733211263854));
#99848=CARTESIAN_POINT('Ctrl Pts',(12.1278783154331,601.321481049692,62.3196016812068));
#99849=CARTESIAN_POINT('Ctrl Pts',(12.6301721078754,601.329429458576,62.2419960871396));
#99850=CARTESIAN_POINT('Ctrl Pts',(12.0642627442628,601.876841506454,61.966781870534));
#99851=CARTESIAN_POINT('Ctrl Pts',(12.0518668066587,601.369077315824,61.9013451715682));
#99852=CARTESIAN_POINT('Ctrl Pts',(12.5554981065861,601.380798685877,61.8077390713353));
#99853=CARTESIAN_POINT('Ctrl Pts',(11.8816140310333,602.003262763878,61.166562295788));
#99854=CARTESIAN_POINT('Ctrl Pts',(11.8592631718102,601.488601905001,61.0802544646279));
#99855=CARTESIAN_POINT('Ctrl Pts',(12.3654120067484,601.510556548268,60.9529607510218));
#99856=CARTESIAN_POINT('Ctrl Pts',(11.7707128919438,602.079641820668,60.772884098279));
#99857=CARTESIAN_POINT('Ctrl Pts',(11.7418361923576,601.561038683665,60.6757975217571));
#99858=CARTESIAN_POINT('Ctrl Pts',(12.24999503422,601.588951446709,60.5324417644507));
#99859=CARTESIAN_POINT('Ctrl Pts',(11.5101835598806,602.257123807651,59.9980565322959));
#99860=CARTESIAN_POINT('Ctrl Pts',(11.4672537822116,601.728288580003,59.8820278090674));
#99861=CARTESIAN_POINT('Ctrl Pts',(11.9788570767703,601.771117661675,59.7047869321897));
#99862=CARTESIAN_POINT('Ctrl Pts',(11.3599469816121,602.358621283629,59.6161284319979));
#99863=CARTESIAN_POINT('Ctrl Pts',(11.3083541540513,601.824109992935,59.4906070974741));
#99864=CARTESIAN_POINT('Ctrl Pts',(11.8225029661159,601.875293914858,59.2968193042848));
#99865=CARTESIAN_POINT('Ctrl Pts',(10.8623141995672,602.690011075352,58.5132634066806));
#99866=CARTESIAN_POINT('Ctrl Pts',(10.7793394197783,602.137864461831,58.3527219119798));
#99867=CARTESIAN_POINT('Ctrl Pts',(11.3046070446312,602.215429860194,58.1187624395528));
#99868=CARTESIAN_POINT('Ctrl Pts',(10.4661234341584,602.948411668527,57.826102858912));
#99869=CARTESIAN_POINT('Ctrl Pts',(10.356765890555,602.381898559536,57.6501409533267));
#99870=CARTESIAN_POINT('Ctrl Pts',(10.8922838620022,602.480650216832,57.38475245639));
#99871=CARTESIAN_POINT('Ctrl Pts',(9.77894881027317,603.375457962377,56.8598623147943));
#99872=CARTESIAN_POINT('Ctrl Pts',(9.64506765475245,602.77115804364,56.6833001238243));
#99873=CARTESIAN_POINT('Ctrl Pts',(10.1771279455515,602.918967477386,56.3526354312712));
#99874=CARTESIAN_POINT('Ctrl Pts',(9.53441356862628,603.524266415077,56.5491977096818));
#99875=CARTESIAN_POINT('Ctrl Pts',(9.3881532972667,602.908133560702,56.3693702079608));
#99876=CARTESIAN_POINT('Ctrl Pts',(9.92263552743373,603.071703338872,56.0207905222547));
#99877=CARTESIAN_POINT('Ctrl Pts',(9.02298980808865,603.826597991785,55.9593613574983));
#99878=CARTESIAN_POINT('Ctrl Pts',(8.85332952510663,603.18403735001,55.7753564682485));
#99879=CARTESIAN_POINT('Ctrl Pts',(9.39038724050548,603.382014172498,55.3907408801181));
#99880=CARTESIAN_POINT('Ctrl Pts',(8.75507913189959,603.980773157895,55.6786872175428));
#99881=CARTESIAN_POINT('Ctrl Pts',(8.57309886107225,603.323937574205,55.4940908270661));
#99882=CARTESIAN_POINT('Ctrl Pts',(9.11156762612114,603.540258381175,55.090931316096));
#99883=CARTESIAN_POINT('Ctrl Pts',(8.19463976841416,604.291810284563,55.1442976661868));
#99884=CARTESIAN_POINT('Ctrl Pts',(7.98991581692825,603.603406408195,54.9607215721971));
#99885=CARTESIAN_POINT('Ctrl Pts',(8.52830801024527,603.859504509158,54.5201090911092));
#99886=CARTESIAN_POINT('Ctrl Pts',(7.90211495074044,604.44868351391,54.8905842355243));
#99887=CARTESIAN_POINT('Ctrl Pts',(7.68581591431249,603.743146615829,54.7092695072828));
#99888=CARTESIAN_POINT('Ctrl Pts',(8.2238720660799,604.020517985683,54.249098530159));
#99889=CARTESIAN_POINT('Ctrl Pts',(7.29112855786425,604.761500763142,54.4095765831193));
#99890=CARTESIAN_POINT('Ctrl Pts',(7.05467644855106,604.018499588404,54.235046571121));
#99891=CARTESIAN_POINT('Ctrl Pts',(7.58800735659369,604.341591210503,53.7352979823133));
#99892=CARTESIAN_POINT('Ctrl Pts',(6.97101558534139,604.918182407445,54.1813147654603));
#99893=CARTESIAN_POINT('Ctrl Pts',(6.72505953251661,604.154601600561,54.0123480361725));
#99894=CARTESIAN_POINT('Ctrl Pts',(7.25485997662567,604.502408049335,53.4914744107168));
#99895=CARTESIAN_POINT('Ctrl Pts',(5.98483237209617,605.372809378709,53.5471616990657));
#99896=CARTESIAN_POINT('Ctrl Pts',(5.69764408550192,604.551590711133,53.3856625261571));
#99897=CARTESIAN_POINT('Ctrl Pts',(6.2285217108747,604.969033495642,52.8140885319357));
#99898=CARTESIAN_POINT('Ctrl Pts',(5.291763389905,605.656883943073,53.1889683039969));
#99899=CARTESIAN_POINT('Ctrl Pts',(4.99883657181497,604.782956995844,53.0534099549068));
#99900=CARTESIAN_POINT('Ctrl Pts',(5.50723239645897,605.260605545413,52.4314756793782));
#99901=CARTESIAN_POINT('Ctrl Pts',(4.18911713925861,606.025248782652,52.7483954928647));
#99902=CARTESIAN_POINT('Ctrl Pts',(3.92944127969241,605.069509242206,52.6545633889695));
#99903=CARTESIAN_POINT('Ctrl Pts',(4.35968842339054,605.638692597612,51.9608675862803));
#99904=CARTESIAN_POINT('Ctrl Pts',(3.81096175995496,606.138324284714,52.6178133054263));
#99905=CARTESIAN_POINT('Ctrl Pts',(3.56120429928033,605.155992497434,52.5373866738974));
#99906=CARTESIAN_POINT('Ctrl Pts',(3.9661354003342,605.754752469228,51.8213832724702));
#99907=CARTESIAN_POINT('Ctrl Pts',(3.00672598670703,606.344708975615,52.3845762519713));
#99908=CARTESIAN_POINT('Ctrl Pts',(2.78594596552362,605.311313687175,52.3295333561008));
#99909=CARTESIAN_POINT('Ctrl Pts',(3.12915300807807,605.966584199717,51.5722459548577));
#99910=CARTESIAN_POINT('Ctrl Pts',(2.57673878094782,606.43650711821,52.283993642024));
#99911=CARTESIAN_POINT('Ctrl Pts',(2.37958814121467,605.377182855783,52.2431427434406));
#99912=CARTESIAN_POINT('Ctrl Pts',(2.68165673811207,606.060805327666,51.464806254603));
#99913=CARTESIAN_POINT('Ctrl Pts',(2.14707264243295,606.506964973997,52.2077657609361));
#99914=CARTESIAN_POINT('Ctrl Pts',(1.98191615594632,605.426670682687,52.1785498499702));
#99915=CARTESIAN_POINT('Ctrl Pts',(2.23449661093605,606.133122595151,51.3833819921005));
#99916=CARTESIAN_POINT('',(2.22051577456844,606.494663641934,52.2210317180765));
#99917=CARTESIAN_POINT('',(4.22249409534898E-10,606.684224932409,76.580334695687));
#99918=CARTESIAN_POINT('Ctrl Pts',(2.22051577456844,606.494663641934,52.2210317180765));
#99919=CARTESIAN_POINT('Ctrl Pts',(2.60483303074393,606.429484540379,52.2916850774771));
#99920=CARTESIAN_POINT('Ctrl Pts',(2.98704755411254,606.347911981023,52.381202132682));
#99921=CARTESIAN_POINT('Ctrl Pts',(3.72765041168058,606.161164801006,52.5916868547165));
#99922=CARTESIAN_POINT('Ctrl Pts',(4.08671405697885,606.056144140749,52.7124754929602));
#99923=CARTESIAN_POINT('Ctrl Pts',(5.1345743018316,605.714430404768,53.1183811864826));
#99924=CARTESIAN_POINT('Ctrl Pts',(5.79438301248105,605.451397101099,53.4465291776656));
#99925=CARTESIAN_POINT('Ctrl Pts',(6.7355315478591,605.029219853622,54.0238946887425));
#99926=CARTESIAN_POINT('Ctrl Pts',(7.04239893277636,604.883107748655,54.2317409141202));
#99927=CARTESIAN_POINT('Ctrl Pts',(7.63205469932197,604.589122876331,54.6710591065219));
#99928=CARTESIAN_POINT('Ctrl Pts',(7.91508088583165,604.441230479337,54.9024484325785));
#99929=CARTESIAN_POINT('Ctrl Pts',(8.73098867449171,603.999577513356,55.6321883543658));
#99930=CARTESIAN_POINT('Ctrl Pts',(9.23111241966252,603.707850689127,56.1656879276833));
#99931=CARTESIAN_POINT('Ctrl Pts',(9.91630154576906,603.290954132867,57.0451969084296));
#99932=CARTESIAN_POINT('Ctrl Pts',(10.1324915118317,603.156183694246,57.3502753776917));
#99933=CARTESIAN_POINT('Ctrl Pts',(10.5357713613976,602.900401551024,57.9783769701487));
#99934=CARTESIAN_POINT('Ctrl Pts',(10.7236262872103,602.778919608739,58.3023594003029));
#99935=CARTESIAN_POINT('Ctrl Pts',(11.0712376013219,602.551117160149,58.9713183751389));
#99936=CARTESIAN_POINT('Ctrl Pts',(11.2309988089124,602.444788739996,59.3162894189298));
#99937=CARTESIAN_POINT('Ctrl Pts',(11.5208797326646,602.249914737681,60.0290181547742));
#99938=CARTESIAN_POINT('Ctrl Pts',(11.6501690769847,602.161922525909,60.3953019668914));
#99939=CARTESIAN_POINT('Ctrl Pts',(11.9839910541968,601.933170100156,61.5063440997196));
#99940=CARTESIAN_POINT('Ctrl Pts',(12.1379146213264,601.825487893945,62.2699324426638));
#99941=CARTESIAN_POINT('Ctrl Pts',(12.2580662787846,601.741388185839,63.4530645764399));
#99942=CARTESIAN_POINT('Ctrl Pts',(12.2789163285454,601.726736270966,63.8499267607108));
#99943=CARTESIAN_POINT('Ctrl Pts',(12.2825378585981,601.724194293723,64.6358410829958));
#99944=CARTESIAN_POINT('Ctrl Pts',(12.2655225913637,601.736153568246,65.0268582260156));
#99945=CARTESIAN_POINT('Ctrl Pts',(12.1944767448526,601.785908540228,65.8050866022495));
#99946=CARTESIAN_POINT('Ctrl Pts',(12.1404459138046,601.82370562741,66.1922977510875));
#99947=CARTESIAN_POINT('Ctrl Pts',(11.9949724860648,601.92483744177,66.9629011030374));
#99948=CARTESIAN_POINT('Ctrl Pts',(11.903019104308,601.988518090871,67.3470686022024));
#99949=CARTESIAN_POINT('Ctrl Pts',(11.5792106607343,602.210767543754,68.4638808611085));
#99950=CARTESIAN_POINT('Ctrl Pts',(11.2984041214378,602.401449237337,69.1715940183495));
#99951=CARTESIAN_POINT('Ctrl Pts',(10.7859893300428,602.73835379426,70.1837668701614));
#99952=CARTESIAN_POINT('Ctrl Pts',(10.5987639460202,602.859865399784,70.5144589620626));
#99953=CARTESIAN_POINT('Ctrl Pts',(10.2001915144139,603.113663105627,71.1489943075356));
#99954=CARTESIAN_POINT('Ctrl Pts',(9.98878898534629,603.246010799224,71.4534198335247));
#99955=CARTESIAN_POINT('Ctrl Pts',(9.31947230013895,603.655393049318,72.3311884350087));
#99956=CARTESIAN_POINT('Ctrl Pts',(8.82689483618176,603.944863634538,72.8693491319149));
#99957=CARTESIAN_POINT('Ctrl Pts',(8.01529581017258,604.388031905717,73.6112320344375));
#99958=CARTESIAN_POINT('Ctrl Pts',(7.73182881330978,604.537533259381,73.8478989536329));
#99959=CARTESIAN_POINT('Ctrl Pts',(7.14908314421362,604.831207252798,74.2916812721146));
#99960=CARTESIAN_POINT('Ctrl Pts',(6.84872810477117,604.976001626505,74.4998846147026));
#99961=CARTESIAN_POINT('Ctrl Pts',(5.91918799038042,605.399129104306,75.0845859838612));
#99962=CARTESIAN_POINT('Ctrl Pts',(5.26207272556291,605.666687613147,75.4217452738926));
#99963=CARTESIAN_POINT('Ctrl Pts',(4.20600812444231,606.019585586432,75.8438524767));
#99964=CARTESIAN_POINT('Ctrl Pts',(3.84458489423226,606.128056920297,75.9693060886928));
#99965=CARTESIAN_POINT('Ctrl Pts',(3.11078512019224,606.319311478279,76.185971800507));
#99966=CARTESIAN_POINT('Ctrl Pts',(2.73707032232845,606.402551374238,76.2777372174655));
#99967=CARTESIAN_POINT('Ctrl Pts',(1.97462989968799,606.539511783188,76.4267647296646));
#99968=CARTESIAN_POINT('Ctrl Pts',(1.58407504305315,606.593371762541,76.4841860202651));
#99969=CARTESIAN_POINT('Ctrl Pts',(0.795241544847691,606.665735849296,76.5609621502088));
#99970=CARTESIAN_POINT('Ctrl Pts',(0.400287481815783,606.684227202053,76.5803315661586));
#99971=CARTESIAN_POINT('Ctrl Pts',(5.83190623966335E-15,606.684227202053,
76.5803315661586));
#99972=CARTESIAN_POINT('',(2.31092134190293,606.120502424978,51.3976052199539));
#99973=CARTESIAN_POINT('Origin',(2.31092134187393,606.494663641934,51.7292728001094));
#99974=CARTESIAN_POINT('',(-2.26224148372674,606.128561192588,77.2104285068931));
#99975=CARTESIAN_POINT('Ctrl Pts',(-2.26224148372674,606.128561192588,77.2104285068931));
#99976=CARTESIAN_POINT('Ctrl Pts',(-1.83032423084503,606.199321946877,77.2901548692284));
#99977=CARTESIAN_POINT('Ctrl Pts',(-1.39473620312201,606.250907869188,77.3470551071421));
#99978=CARTESIAN_POINT('Ctrl Pts',(-0.515891315837579,606.31235552653,77.4146673352173));
#99979=CARTESIAN_POINT('Ctrl Pts',(-0.0702880625902517,606.322061908389,
77.4252220449457));
#99980=CARTESIAN_POINT('Ctrl Pts',(0.814508254993039,606.297917403733,77.3987706058388));
#99981=CARTESIAN_POINT('Ctrl Pts',(1.25591590129853,606.264149217592,77.3618450733092));
#99982=CARTESIAN_POINT('Ctrl Pts',(2.12632669303214,606.156946302591,77.2425878065961));
#99983=CARTESIAN_POINT('Ctrl Pts',(2.55179819911838,606.084174367916,77.1609561180698));
#99984=CARTESIAN_POINT('Ctrl Pts',(3.38538928239685,605.906592410097,76.9566426950186));
#99985=CARTESIAN_POINT('Ctrl Pts',(3.79350628097141,605.801783546111,76.833949796622));
#99986=CARTESIAN_POINT('Ctrl Pts',(4.5939136248181,605.565907235288,76.5485878713385));
#99987=CARTESIAN_POINT('Ctrl Pts',(4.98575248625829,605.434795373065,76.3857550747386));
#99988=CARTESIAN_POINT('Ctrl Pts',(6.11412644163187,605.020347147677,75.850504898419));
#99989=CARTESIAN_POINT('Ctrl Pts',(6.81399404095514,604.713607705726,75.4287590544389));
#99990=CARTESIAN_POINT('Ctrl Pts',(7.79889285265662,604.237467754231,74.7005250396438));
#99991=CARTESIAN_POINT('Ctrl Pts',(8.11734298004477,604.075354707554,74.4406405058552));
#99992=CARTESIAN_POINT('Ctrl Pts',(8.72762915407622,603.75229671606,73.8918331418519));
#99993=CARTESIAN_POINT('Ctrl Pts',(9.01787207664488,603.592262947776,73.6045582479782));
#99994=CARTESIAN_POINT('Ctrl Pts',(9.84637516857155,603.121737222959,72.7037235931987));
#99995=CARTESIAN_POINT('Ctrl Pts',(10.3429614399288,602.820770001216,72.0516283531007));
#99996=CARTESIAN_POINT('Ctrl Pts',(11.0032431948168,602.407067467609,70.9865177450937));
#99997=CARTESIAN_POINT('Ctrl Pts',(11.2093789343219,602.275251835416,70.6157898317709));
#99998=CARTESIAN_POINT('Ctrl Pts',(11.5836014028183,602.032675897713,69.8591636321725));
#99999=CARTESIAN_POINT('Ctrl Pts',(11.7528969072206,601.921164391175,69.4715259668061));
#100000=CARTESIAN_POINT('Ctrl Pts',(12.0554510123091,601.719930759937,68.6768786107822));
#100001=CARTESIAN_POINT('Ctrl Pts',(12.1887140449545,601.630200580394,68.2698726655556));
#100002=CARTESIAN_POINT('Ctrl Pts',(12.4175304640208,601.475114177481,67.4351906357858));
#100003=CARTESIAN_POINT('Ctrl Pts',(12.5132629458602,601.409630372534,67.0052234510874));
#100004=CARTESIAN_POINT('Ctrl Pts',(12.7346497723208,601.257655920815,65.7152869175487));
#100005=CARTESIAN_POINT('Ctrl Pts',(12.7982740854582,601.213319476748,64.8470309669364));
#100006=CARTESIAN_POINT('Ctrl Pts',(12.766112503726,601.235579417349,63.5319360416885));
#100007=CARTESIAN_POINT('Ctrl Pts',(12.7334707525218,601.258186828756,63.0884936792983));
#100008=CARTESIAN_POINT('Ctrl Pts',(12.6260778331749,601.332207022654,62.2172823473981));
#100009=CARTESIAN_POINT('Ctrl Pts',(12.551632369959,601.383407841326,61.788489253183));
#100010=CARTESIAN_POINT('Ctrl Pts',(12.3628457782987,601.51225949665,60.9438749494673));
#100011=CARTESIAN_POINT('Ctrl Pts',(12.2485007430305,601.589915970709,60.5280554739999));
#100012=CARTESIAN_POINT('Ctrl Pts',(11.9802058693947,601.770170646653,59.7090936426398));
#100013=CARTESIAN_POINT('Ctrl Pts',(11.8256357552361,601.873166560103,59.3051045068694));
#100014=CARTESIAN_POINT('Ctrl Pts',(11.3133789750381,602.209683025684,58.1368724774906));
#100015=CARTESIAN_POINT('Ctrl Pts',(10.9053335034014,602.472295759362,57.4071299613224));
#100016=CARTESIAN_POINT('Ctrl Pts',(10.1963986672724,602.907259896225,56.3789236860282));
#100017=CARTESIAN_POINT('Ctrl Pts',(9.94375223192614,603.059090221129,56.0476855370183));
#100018=CARTESIAN_POINT('Ctrl Pts',(9.41478615234259,603.367978324838,55.4180596023799));
#100019=CARTESIAN_POINT('Ctrl Pts',(9.13741954079915,603.525697149408,55.1180679858199));
#100020=CARTESIAN_POINT('Ctrl Pts',(8.55656002383599,603.844325765871,54.5462464538821));
#100021=CARTESIAN_POINT('Ctrl Pts',(8.25307216483238,604.005247212705,54.2744178365614));
#100022=CARTESIAN_POINT('Ctrl Pts',(7.61843493119114,604.326614811804,53.7584611953167));
#100023=CARTESIAN_POINT('Ctrl Pts',(7.28550391450078,604.487856905221,53.513234090336));
#100024=CARTESIAN_POINT('Ctrl Pts',(6.25785460882906,604.956716882825,52.8307763736279));
#100025=CARTESIAN_POINT('Ctrl Pts',(5.53420093242913,605.250586826674,52.4443472052227));
#100026=CARTESIAN_POINT('Ctrl Pts',(4.37964798732873,605.632586367383,51.9682761050355));
#100027=CARTESIAN_POINT('Ctrl Pts',(3.98317189683697,605.750021198994,51.8270164181643));
#100028=CARTESIAN_POINT('Ctrl Pts',(3.16332124464332,605.958246731221,51.5819852864849));
#100029=CARTESIAN_POINT('Ctrl Pts',(2.73846394280183,606.048990746731,51.478279057735));
#100030=CARTESIAN_POINT('Ctrl Pts',(2.31092134190293,606.120502424978,51.3976052199539));
#100031=CARTESIAN_POINT('',(-2.17374032143659,606.502515243277,76.3864221483552));
#100032=CARTESIAN_POINT('Origin',(-2.26224148372674,606.502515243277,76.8785273650246));
#100033=CARTESIAN_POINT('Ctrl Pts',(3.771343681791E-9,606.684206930352,
76.5803595180565));
#100034=CARTESIAN_POINT('Ctrl Pts',(-0.346198564393155,606.684165521778,
76.5804168433102));
#100035=CARTESIAN_POINT('Ctrl Pts',(-0.689932235512485,606.670170944619,
76.5658934870616));
#100036=CARTESIAN_POINT('Ctrl Pts',(-1.03129404442789,606.643008160357,
76.5371136743068));
#100037=CARTESIAN_POINT('Ctrl Pts',(-1.05249997323572,606.641320765768,
76.5353258273818));
#100038=CARTESIAN_POINT('Ctrl Pts',(-1.07369674828705,606.639582538745,
76.5334829566656));
#100039=CARTESIAN_POINT('Ctrl Pts',(-1.09488439167535,606.637793661485,
76.5315851371587));
#100040=CARTESIAN_POINT('Ctrl Pts',(-1.43870745097142,606.6087646071,76.5007882194979));
#100041=CARTESIAN_POINT('Ctrl Pts',(-1.78012200264755,606.566401949312,
76.4555237331009));
#100042=CARTESIAN_POINT('Ctrl Pts',(-2.11922347843876,606.51145981661,76.3961009878374));
#100043=CARTESIAN_POINT('Ctrl Pts',(-2.13740240261687,606.508514418445,
76.3929153880753));
#100044=CARTESIAN_POINT('Ctrl Pts',(-2.1555746787607,606.505532856527,76.3896890929762));
#100045=CARTESIAN_POINT('Ctrl Pts',(-2.17374032143659,606.502515243277,
76.3864221483552));
#100046=CARTESIAN_POINT('Ctrl Pts',(2.24785136038932,634.860698008622,76.3728616211674));
#100047=CARTESIAN_POINT('Ctrl Pts',(2.07645831265176,635.936120444547,76.4046723372692));
#100048=CARTESIAN_POINT('Ctrl Pts',(2.33937824032558,635.234986741416,77.1959965376062));
#100049=CARTESIAN_POINT('Ctrl Pts',(1.40572798249692,634.716125995138,76.529590213006));
#100050=CARTESIAN_POINT('Ctrl Pts',(1.26541701307411,635.830503847675,76.5426302087904));
#100051=CARTESIAN_POINT('Ctrl Pts',(1.4629706737577,635.086599899663,77.3634086157443));
#100052=CARTESIAN_POINT('Ctrl Pts',(0.558874392731051,634.650489722876,
76.5971497221977));
#100053=CARTESIAN_POINT('Ctrl Pts',(0.514725151119972,635.789908982322,
76.5942633105082));
#100054=CARTESIAN_POINT('Ctrl Pts',(0.581630402765628,635.019230511953,
77.4355745853267));
#100055=CARTESIAN_POINT('Ctrl Pts',(-0.706100277663284,634.679151948051,
76.5669850049637));
#100056=CARTESIAN_POINT('Ctrl Pts',(-0.646113299414298,635.809408002983,
76.5691293178845));
#100057=CARTESIAN_POINT('Ctrl Pts',(-0.734851049714807,635.048649217997,
77.4033535057653));
#100058=CARTESIAN_POINT('Ctrl Pts',(-1.12182523736719,634.708561737361,
76.536110530326));
#100059=CARTESIAN_POINT('Ctrl Pts',(-1.02513407763589,635.829024835917,
76.5438803998928));
#100060=CARTESIAN_POINT('Ctrl Pts',(-1.16750341452898,635.078835227031,
77.3703742754706));
#100061=CARTESIAN_POINT('Ctrl Pts',(-1.95026027616437,634.806432676349,
76.4316729163024));
#100062=CARTESIAN_POINT('Ctrl Pts',(-1.7932742144534,635.897133191657,76.4555825442098));
#100063=CARTESIAN_POINT('Ctrl Pts',(-2.02967039801753,635.179289265266,
77.2588170101285));
#100064=CARTESIAN_POINT('Ctrl Pts',(-2.35571831397255,634.873855121138,
76.3591800393728));
#100065=CARTESIAN_POINT('Ctrl Pts',(-2.17101933655468,635.944154964474,
76.3944710230165));
#100066=CARTESIAN_POINT('Ctrl Pts',(-2.45163778157809,635.24849119524,77.1813821711449));
#100067=CARTESIAN_POINT('Ctrl Pts',(-3.1509275003985,635.039899812196,76.1762401766097));
#100068=CARTESIAN_POINT('Ctrl Pts',(-2.92564597397709,636.065276169395,
76.2348538665947));
#100069=CARTESIAN_POINT('Ctrl Pts',(-3.27922604287813,635.418918265005,
76.9859709699881));
#100070=CARTESIAN_POINT('Ctrl Pts',(-3.54067700376127,635.138519958425,
76.0657839944311));
#100071=CARTESIAN_POINT('Ctrl Pts',(-3.29897216237785,636.138164540395,
76.1380212205395));
#100072=CARTESIAN_POINT('Ctrl Pts',(-3.68484527501564,635.52014127825,76.8679847444036));
#100073=CARTESIAN_POINT('Ctrl Pts',(-4.30578941666223,635.361584800423,
75.8078458454146));
#100074=CARTESIAN_POINT('Ctrl Pts',(-4.04402710457129,636.309799217015,
75.9048203360756));
#100075=CARTESIAN_POINT('Ctrl Pts',(-4.48111132932761,635.74909338184,76.592462321494));
#100076=CARTESIAN_POINT('Ctrl Pts',(-4.68185936719358,635.486434419437,
75.6597967341437));
#100077=CARTESIAN_POINT('Ctrl Pts',(-4.4142825517745,636.407595840929,75.7698350030814));
#100078=CARTESIAN_POINT('Ctrl Pts',(-4.87249402091242,635.87723811095,76.434320270781));
#100079=CARTESIAN_POINT('Ctrl Pts',(-5.76664965320651,635.882977449259,
75.1711954372518));
#100080=CARTESIAN_POINT('Ctrl Pts',(-5.47578346481422,636.72231885161,75.3217454446976));
#100081=CARTESIAN_POINT('Ctrl Pts',(-6.00145504788508,636.284247044183,
75.9124092474765));
#100082=CARTESIAN_POINT('Ctrl Pts',(-6.44125011399587,636.178479594726,
74.7843144301781));
#100083=CARTESIAN_POINT('Ctrl Pts',(-6.16307079581405,636.968558930894,
74.9571009510356));
#100084=CARTESIAN_POINT('Ctrl Pts',(-6.70352384989611,636.58754824298,75.4991529048738));
#100085=CARTESIAN_POINT('Ctrl Pts',(-7.39260369019896,636.639599638778,
74.113718938762));
#100086=CARTESIAN_POINT('Ctrl Pts',(-7.158977865901,637.376320023169,74.2892807227981));
#100087=CARTESIAN_POINT('Ctrl Pts',(-7.69361438062197,637.060838120451,
74.7828399123805));
#100088=CARTESIAN_POINT('Ctrl Pts',(-7.69999421515548,636.79667333918,73.8745480813112));
#100089=CARTESIAN_POINT('Ctrl Pts',(-7.47684208610699,637.514346864805,
74.0542734601019));
#100090=CARTESIAN_POINT('Ctrl Pts',(-8.01352130722838,637.222057361665,
74.5273634858686));
#100091=CARTESIAN_POINT('Ctrl Pts',(-8.29275501798799,637.112034149181,
73.366015200935));
#100092=CARTESIAN_POINT('Ctrl Pts',(-8.09137141934416,637.794687681408,
73.5499197260926));
#100093=CARTESIAN_POINT('Ctrl Pts',(-8.63041836958322,637.545741279659,
73.9841609752445));
#100094=CARTESIAN_POINT('Ctrl Pts',(-8.57500490891427,637.268622767296,
73.0994134185157));
#100095=CARTESIAN_POINT('Ctrl Pts',(-8.38578298933439,637.935474512246,
73.2841816609334));
#100096=CARTESIAN_POINT('Ctrl Pts',(-8.92416103428733,637.706462633295,
73.699383292471));
#100097=CARTESIAN_POINT('Ctrl Pts',(-9.38165373201378,637.729995910346,
72.2621847580794));
#100098=CARTESIAN_POINT('Ctrl Pts',(-9.21438704392967,638.346761115296,
72.457713450177));
#100099=CARTESIAN_POINT('Ctrl Pts',(-9.76365581150139,638.180012699049,
72.8050748647866));
#100100=CARTESIAN_POINT('Ctrl Pts',(-9.86648097776597,638.026433701836,
71.6546027950791));
#100101=CARTESIAN_POINT('Ctrl Pts',(-9.72827362326668,638.621434606878,
71.8438171025925));
#100102=CARTESIAN_POINT('Ctrl Pts',(-10.268224529173,638.484274141068,72.1560695767887));
#100103=CARTESIAN_POINT('Ctrl Pts',(-10.5131125646575,638.435650574758,
70.6595371105421));
#100104=CARTESIAN_POINT('Ctrl Pts',(-10.4161108402936,639.005732396094,
70.8199643162107));
#100105=CARTESIAN_POINT('Ctrl Pts',(-10.9411861049551,638.904291127409,
71.093162634049));
#100106=CARTESIAN_POINT('Ctrl Pts',(-10.7157975268765,638.566634249657,
70.3120817185629));
#100107=CARTESIAN_POINT('Ctrl Pts',(-10.6299402839476,639.128103933932,
70.4658892792961));
#100108=CARTESIAN_POINT('Ctrl Pts',(-11.1521242095175,639.038731783309,
70.7220183137494));
#100109=CARTESIAN_POINT('Ctrl Pts',(-11.084674691934,638.808411601172,69.6013374038106));
#100110=CARTESIAN_POINT('Ctrl Pts',(-11.0180928131925,639.354068221639,
69.7407948866329));
#100111=CARTESIAN_POINT('Ctrl Pts',(-11.5360217752982,639.286890263696,
69.9628164177921));
#100112=CARTESIAN_POINT('Ctrl Pts',(-11.2518487421506,638.919811820504,
69.2368447373392));
#100113=CARTESIAN_POINT('Ctrl Pts',(-11.1947990337117,639.458916920981,
69.3678350652566));
#100114=CARTESIAN_POINT('Ctrl Pts',(-11.7100030252518,639.401230614902,
69.5734730530018));
#100115=CARTESIAN_POINT('Ctrl Pts',(-11.5512173099189,639.121328387605,
68.4888783550686));
#100116=CARTESIAN_POINT('Ctrl Pts',(-11.5101732026521,639.648338417762,
68.602538540975));
#100117=CARTESIAN_POINT('Ctrl Pts',(-12.0215617073794,639.608065739894,
68.7745109630704));
#100118=CARTESIAN_POINT('Ctrl Pts',(-11.6834165707129,639.211453174224,
68.1054086939742));
#100119=CARTESIAN_POINT('Ctrl Pts',(-11.6500527589344,639.733596073901,
68.2091225258213));
#100120=CARTESIAN_POINT('Ctrl Pts',(-12.1591440413973,639.700569151504,
68.3648966030017));
#100121=CARTESIAN_POINT('Ctrl Pts',(-11.9111236037372,639.36775953649,67.3181651639018));
#100122=CARTESIAN_POINT('Ctrl Pts',(-11.8901059250353,639.88112388843,67.4020108101632));
#100123=CARTESIAN_POINT('Ctrl Pts',(-12.3961232041754,639.861000864439,
67.5239791695796));
#100124=CARTESIAN_POINT('Ctrl Pts',(-12.0069667791483,639.434178741944,
66.911668961761));
#100125=CARTESIAN_POINT('Ctrl Pts',(-11.9916079185947,639.944196752873,
66.9841120694482));
#100126=CARTESIAN_POINT('Ctrl Pts',(-12.4958690656149,639.929173046546,
67.089768199197));
#100127=CARTESIAN_POINT('Ctrl Pts',(-12.2299344763514,639.589281206055,
65.690004883469));
#100128=CARTESIAN_POINT('Ctrl Pts',(-12.2258063111646,640.090389507445,
65.7350813999209));
#100129=CARTESIAN_POINT('Ctrl Pts',(-12.7279159619353,640.088369114275,
65.7848111091887));
#100130=CARTESIAN_POINT('Ctrl Pts',(-12.2958567378873,639.635861093889,
64.8673118420714));
#100131=CARTESIAN_POINT('Ctrl Pts',(-12.2966228016026,640.135397612622,
64.8820610902705));
#100132=CARTESIAN_POINT('Ctrl Pts',(-12.7965225255398,640.136178350411,
64.9060270614251));
#100133=CARTESIAN_POINT('Ctrl Pts',(-12.2691242107389,639.617099488461,
63.6206371830607));
#100134=CARTESIAN_POINT('Ctrl Pts',(-12.2684356679881,640.117618390571,
63.6017923894247));
#100135=CARTESIAN_POINT('Ctrl Pts',(-12.7687014560783,640.116921573656,
63.5743540715744));
#100136=CARTESIAN_POINT('Ctrl Pts',(-12.2386272268548,639.595678765416,
63.199960706747));
#100137=CARTESIAN_POINT('Ctrl Pts',(-12.2361148149089,640.097213244929,
63.1686064467318));
#100138=CARTESIAN_POINT('Ctrl Pts',(-12.7369626473579,640.094935500868,
63.1249959000212));
#100139=CARTESIAN_POINT('Ctrl Pts',(-12.1360150250495,639.523954342629,
62.3733211263854));
#100140=CARTESIAN_POINT('Ctrl Pts',(-12.1278783154334,640.029266479055,
62.3196016812068));
#100141=CARTESIAN_POINT('Ctrl Pts',(-12.6301721078756,640.021318070172,
62.2419960871396));
#100142=CARTESIAN_POINT('Ctrl Pts',(-12.0642627442628,639.473906022293,
61.966781870534));
#100143=CARTESIAN_POINT('Ctrl Pts',(-12.051866806659,639.981670212924,61.9013451715682));
#100144=CARTESIAN_POINT('Ctrl Pts',(-12.5554981065862,639.96994884287,61.8077390713353));
#100145=CARTESIAN_POINT('Ctrl Pts',(-11.8816140310333,639.34748476487,61.1665622957879));
#100146=CARTESIAN_POINT('Ctrl Pts',(-11.8592631718105,639.862145623747,
61.0802544646277));
#100147=CARTESIAN_POINT('Ctrl Pts',(-12.3654120067485,639.840190980479,
60.9529607510217));
#100148=CARTESIAN_POINT('Ctrl Pts',(-11.7707128919438,639.271105708079,
60.772884098279));
#100149=CARTESIAN_POINT('Ctrl Pts',(-11.7418361923579,639.789708845082,
60.675797521757));
#100150=CARTESIAN_POINT('Ctrl Pts',(-12.2499950342201,639.761796082038,
60.5324417644507));
#100151=CARTESIAN_POINT('Ctrl Pts',(-11.5101835598806,639.093623721097,
59.9980565322958));
#100152=CARTESIAN_POINT('Ctrl Pts',(-11.4672537822119,639.622458948745,
59.8820278090672));
#100153=CARTESIAN_POINT('Ctrl Pts',(-11.9788570767705,639.579629867072,
59.7047869321897));
#100154=CARTESIAN_POINT('Ctrl Pts',(-11.3599469816121,638.992126245118,
59.6161284319978));
#100155=CARTESIAN_POINT('Ctrl Pts',(-11.3083541540516,639.526637535813,
59.490607097474));
#100156=CARTESIAN_POINT('Ctrl Pts',(-11.822502966116,639.47545361389,59.2968193042847));
#100157=CARTESIAN_POINT('Ctrl Pts',(-10.8623141995672,638.660736453396,
58.5132634066805));
#100158=CARTESIAN_POINT('Ctrl Pts',(-10.7793394197786,639.212883066916,
58.3527219119796));
#100159=CARTESIAN_POINT('Ctrl Pts',(-11.3046070446313,639.135317668554,
58.1187624395527));
#100160=CARTESIAN_POINT('Ctrl Pts',(-10.4661234341583,638.402335860221,
57.8261028589119));
#100161=CARTESIAN_POINT('Ctrl Pts',(-10.3567658905553,638.968848969211,
57.6501409533265));
#100162=CARTESIAN_POINT('Ctrl Pts',(-10.8922838620024,638.870097311915,
57.3847524563899));
#100163=CARTESIAN_POINT('Ctrl Pts',(-9.77894881027311,637.975289566371,
56.8598623147942));
#100164=CARTESIAN_POINT('Ctrl Pts',(-9.64506765475275,638.579589485108,
56.6833001238241));
#100165=CARTESIAN_POINT('Ctrl Pts',(-10.1771279455516,638.431780051362,
56.3526354312712));
#100166=CARTESIAN_POINT('Ctrl Pts',(-9.53441356862621,637.826481113671,
56.5491977096817));
#100167=CARTESIAN_POINT('Ctrl Pts',(-9.38815329726699,638.442613968045,
56.3693702079605));
#100168=CARTESIAN_POINT('Ctrl Pts',(-9.92263552743384,638.279044189875,
56.0207905222546));
#100169=CARTESIAN_POINT('Ctrl Pts',(-9.02298980808857,637.524149536963,
55.9593613574982));
#100170=CARTESIAN_POINT('Ctrl Pts',(-8.85332952510693,638.166710178738,
55.7753564682482));
#100171=CARTESIAN_POINT('Ctrl Pts',(-9.39038724050559,637.96873335625,55.390740880118));
#100172=CARTESIAN_POINT('Ctrl Pts',(-8.75507913189951,637.369974370853,
55.6786872175427));
#100173=CARTESIAN_POINT('Ctrl Pts',(-8.57309886107255,638.026809954543,
55.4940908270658));
#100174=CARTESIAN_POINT('Ctrl Pts',(-9.11156762612125,637.810489147573,
55.0909313160959));
#100175=CARTESIAN_POINT('Ctrl Pts',(-8.19463976841408,637.058937244184,
55.1442976661868));
#100176=CARTESIAN_POINT('Ctrl Pts',(-7.98991581692855,637.747341120553,
54.9607215721967));
#100177=CARTESIAN_POINT('Ctrl Pts',(-8.52830801024537,637.491243019589,
54.5201090911091));
#100178=CARTESIAN_POINT('Ctrl Pts',(-7.90211495074035,636.902064014837,
54.8905842355242));
#100179=CARTESIAN_POINT('Ctrl Pts',(-7.6858159143128,637.607600912918,54.7092695072824));
#100180=CARTESIAN_POINT('Ctrl Pts',(-8.22387206608,637.330229543065,54.2490985301589));
#100181=CARTESIAN_POINT('Ctrl Pts',(-7.29112855786415,636.589246765606,
54.4095765831192));
#100182=CARTESIAN_POINT('Ctrl Pts',(-7.05467644855137,637.332247940343,
54.2350465711206));
#100183=CARTESIAN_POINT('Ctrl Pts',(-7.58800735659379,637.009156318244,
53.7352979823133));
#100184=CARTESIAN_POINT('Ctrl Pts',(-6.97101558534129,636.432565121303,
54.1813147654602));
#100185=CARTESIAN_POINT('Ctrl Pts',(-6.72505953251691,637.196145928187,
54.012348036172));
#100186=CARTESIAN_POINT('Ctrl Pts',(-7.25485997662576,636.848339479412,
53.4914744107167));
#100187=CARTESIAN_POINT('Ctrl Pts',(-5.98483237209606,635.977938150039,
53.5471616990657));
#100188=CARTESIAN_POINT('Ctrl Pts',(-5.69764408550223,636.799156817614,
53.3856625261566));
#100189=CARTESIAN_POINT('Ctrl Pts',(-6.22852171087479,636.381714033105,
52.8140885319356));
#100190=CARTESIAN_POINT('Ctrl Pts',(-5.29176338990489,635.693863585674,
53.1889683039969));
#100191=CARTESIAN_POINT('Ctrl Pts',(-4.99883657181527,636.567790532904,
53.0534099549063));
#100192=CARTESIAN_POINT('Ctrl Pts',(-5.50723239645906,636.090141983335,
52.4314756793781));
#100193=CARTESIAN_POINT('Ctrl Pts',(-4.18911713925852,635.325498746096,
52.7483954928647));
#100194=CARTESIAN_POINT('Ctrl Pts',(-3.92944127969268,636.281238286542,
52.6545633889689));
#100195=CARTESIAN_POINT('Ctrl Pts',(-4.35968842339061,635.712054931135,
51.9608675862802));
#100196=CARTESIAN_POINT('Ctrl Pts',(-3.81096175995487,635.212423244034,
52.6178133054263));
#100197=CARTESIAN_POINT('Ctrl Pts',(-3.56120429928059,636.194755031314,
52.5373866738968));
#100198=CARTESIAN_POINT('Ctrl Pts',(-3.96613540033426,635.59599505952,51.8213832724701));
#100199=CARTESIAN_POINT('Ctrl Pts',(-3.0067259866529,635.006038553119,52.3845762519556));
#100200=CARTESIAN_POINT('Ctrl Pts',(-2.78594596547,636.039433841561,52.3295333560857));
#100201=CARTESIAN_POINT('Ctrl Pts',(-3.12915300802187,635.384163329016,
51.5722459548408));
#100202=CARTESIAN_POINT('Ctrl Pts',(-2.57673878083549,634.914240410514,
52.2839936419978));
#100203=CARTESIAN_POINT('Ctrl Pts',(-2.37958814110711,635.973564672946,
52.243142743417));
#100204=CARTESIAN_POINT('Ctrl Pts',(-2.68165673799516,635.289942201056,
51.4648062545748));
#100205=CARTESIAN_POINT('Ctrl Pts',(-2.14707264226455,634.843782554723,
52.2077657609063));
#100206=CARTESIAN_POINT('Ctrl Pts',(-1.98191615578883,635.924076846041,
52.1785498499438));
#100207=CARTESIAN_POINT('Ctrl Pts',(-2.23449661076091,635.217624933568,
51.3833819920685));
#100208=CARTESIAN_POINT('',(-2.22051577456844,634.856083886813,52.2210317180765));
#100209=CARTESIAN_POINT('',(-4.22249464140995E-10,634.666522596339,76.5803346956872));
#100210=CARTESIAN_POINT('Ctrl Pts',(-2.22051577456844,634.856083886813,
52.2210317180765));
#100211=CARTESIAN_POINT('Ctrl Pts',(-2.60483303074393,634.921262988369,
52.2916850774771));
#100212=CARTESIAN_POINT('Ctrl Pts',(-2.98704755411254,635.002835547725,
52.381202132682));
#100213=CARTESIAN_POINT('Ctrl Pts',(-3.72765041168058,635.189582727741,
52.5916868547165));
#100214=CARTESIAN_POINT('Ctrl Pts',(-4.08671405697885,635.294603387999,
52.7124754929602));
#100215=CARTESIAN_POINT('Ctrl Pts',(-5.1345743018316,635.63631712398,53.1183811864826));
#100216=CARTESIAN_POINT('Ctrl Pts',(-5.79438301248105,635.899350427649,
53.4465291776656));
#100217=CARTESIAN_POINT('Ctrl Pts',(-6.7355315478591,636.321527675125,54.0238946887425));
#100218=CARTESIAN_POINT('Ctrl Pts',(-7.04239893277636,636.467639780093,
54.2317409141202));
#100219=CARTESIAN_POINT('Ctrl Pts',(-7.63205469932197,636.761624652416,
54.6710591065219));
#100220=CARTESIAN_POINT('Ctrl Pts',(-7.91508088583165,636.909517049411,
54.9024484325785));
#100221=CARTESIAN_POINT('Ctrl Pts',(-8.73098867449171,637.351170015392,
55.6321883543658));
#100222=CARTESIAN_POINT('Ctrl Pts',(-9.23111241966252,637.64289683962,56.1656879276833));
#100223=CARTESIAN_POINT('Ctrl Pts',(-9.91630154576906,638.059793395881,
57.0451969084296));
#100224=CARTESIAN_POINT('Ctrl Pts',(-10.1324915118317,638.194563834501,
57.3502753776917));
#100225=CARTESIAN_POINT('Ctrl Pts',(-10.5357713613976,638.450345977724,
57.9783769701487));
#100226=CARTESIAN_POINT('Ctrl Pts',(-10.7236262872103,638.571827920009,
58.3023594003029));
#100227=CARTESIAN_POINT('Ctrl Pts',(-11.0712376013219,638.799630368598,
58.9713183751389));
#100228=CARTESIAN_POINT('Ctrl Pts',(-11.2309988089124,638.905958788751,
59.3162894189298));
#100229=CARTESIAN_POINT('Ctrl Pts',(-11.5208797326646,639.100832791066,
60.0290181547742));
#100230=CARTESIAN_POINT('Ctrl Pts',(-11.6501690769847,639.188825002839,
60.3953019668914));
#100231=CARTESIAN_POINT('Ctrl Pts',(-11.9839910541968,639.417577428592,
61.5063440997196));
#100232=CARTESIAN_POINT('Ctrl Pts',(-12.1379146213264,639.525259634802,
62.2699324426638));
#100233=CARTESIAN_POINT('Ctrl Pts',(-12.2580662787846,639.609359342908,
63.4530645764399));
#100234=CARTESIAN_POINT('Ctrl Pts',(-12.2789163285454,639.624011257781,
63.8499267607108));
#100235=CARTESIAN_POINT('Ctrl Pts',(-12.2825378585981,639.626553235025,
64.6358410829958));
#100236=CARTESIAN_POINT('Ctrl Pts',(-12.2655225913637,639.614593960502,
65.0268582260156));
#100237=CARTESIAN_POINT('Ctrl Pts',(-12.1944767448526,639.56483898852,65.8050866022495));
#100238=CARTESIAN_POINT('Ctrl Pts',(-12.1404459138046,639.527041901337,
66.1922977510875));
#100239=CARTESIAN_POINT('Ctrl Pts',(-11.9949724860648,639.425910086977,
66.9629011030374));
#100240=CARTESIAN_POINT('Ctrl Pts',(-11.903019104308,639.362229437876,67.3470686022024));
#100241=CARTESIAN_POINT('Ctrl Pts',(-11.5792106607343,639.139979984994,
68.4638808611085));
#100242=CARTESIAN_POINT('Ctrl Pts',(-11.2984041214378,638.949298291411,
69.1715940183495));
#100243=CARTESIAN_POINT('Ctrl Pts',(-10.7859893300428,638.612393734488,
70.1837668701614));
#100244=CARTESIAN_POINT('Ctrl Pts',(-10.5987639460202,638.490882128964,
70.5144589620626));
#100245=CARTESIAN_POINT('Ctrl Pts',(-10.2001915144139,638.237084423121,
71.1489943075356));
#100246=CARTESIAN_POINT('Ctrl Pts',(-9.98878898534629,638.104736729523,
71.4534198335247));
#100247=CARTESIAN_POINT('Ctrl Pts',(-9.31947230013895,637.695354479429,
72.3311884350087));
#100248=CARTESIAN_POINT('Ctrl Pts',(-8.82689483618176,637.405883894209,
72.8693491319149));
#100249=CARTESIAN_POINT('Ctrl Pts',(-8.01529581017258,636.96271562303,73.6112320344375));
#100250=CARTESIAN_POINT('Ctrl Pts',(-7.73182881330978,636.813214269367,
73.8478989536329));
#100251=CARTESIAN_POINT('Ctrl Pts',(-7.14908314421362,636.51954027595,74.2916812721146));
#100252=CARTESIAN_POINT('Ctrl Pts',(-6.84872810477117,636.374745902242,
74.4998846147026));
#100253=CARTESIAN_POINT('Ctrl Pts',(-5.91918799038042,635.951618424442,
75.0845859838612));
#100254=CARTESIAN_POINT('Ctrl Pts',(-5.26207272556291,635.684059915601,
75.4217452738926));
#100255=CARTESIAN_POINT('Ctrl Pts',(-4.20600812444231,635.331161942316,
75.8438524767));
#100256=CARTESIAN_POINT('Ctrl Pts',(-3.84458489423226,635.22269060845,75.9693060886928));
#100257=CARTESIAN_POINT('Ctrl Pts',(-3.11078512019224,635.031436050469,
76.185971800507));
#100258=CARTESIAN_POINT('Ctrl Pts',(-2.73707032232845,634.94819615451,76.2777372174655));
#100259=CARTESIAN_POINT('Ctrl Pts',(-1.97462989968799,634.81123574556,76.4267647296646));
#100260=CARTESIAN_POINT('Ctrl Pts',(-1.58407504305315,634.757375766206,
76.4841860202651));
#100261=CARTESIAN_POINT('Ctrl Pts',(-0.795241544847691,634.685011679452,
76.5609621502088));
#100262=CARTESIAN_POINT('Ctrl Pts',(-0.400287481815783,634.666520326694,
76.5803315661586));
#100263=CARTESIAN_POINT('Ctrl Pts',(-5.83190623966335E-15,634.666520326694,
76.5803315661586));
#100264=CARTESIAN_POINT('',(-2.31092134190293,635.230245103769,51.3976052199539));
#100265=CARTESIAN_POINT('Origin',(-2.31092134187393,634.856083886813,51.7292728001094));
#100266=CARTESIAN_POINT('',(2.26224148372674,635.222186336159,77.2104285068931));
#100267=CARTESIAN_POINT('Ctrl Pts',(2.26224148372674,635.222186336159,77.2104285068931));
#100268=CARTESIAN_POINT('Ctrl Pts',(1.83032423084503,635.151425581871,77.2901548692284));
#100269=CARTESIAN_POINT('Ctrl Pts',(1.39473620312201,635.099839659559,77.3470551071421));
#100270=CARTESIAN_POINT('Ctrl Pts',(0.515891315837579,635.038392002217,
77.4146673352173));
#100271=CARTESIAN_POINT('Ctrl Pts',(0.0702880625902517,635.028685620358,
77.4252220449457));
#100272=CARTESIAN_POINT('Ctrl Pts',(-0.814508254993039,635.052830125015,
77.3987706058388));
#100273=CARTESIAN_POINT('Ctrl Pts',(-1.25591590129853,635.086598311156,
77.3618450733092));
#100274=CARTESIAN_POINT('Ctrl Pts',(-2.12632669303214,635.193801226157,
77.2425878065961));
#100275=CARTESIAN_POINT('Ctrl Pts',(-2.55179819911838,635.266573160832,
77.1609561180698));
#100276=CARTESIAN_POINT('Ctrl Pts',(-3.38538928239685,635.444155118651,
76.9566426950186));
#100277=CARTESIAN_POINT('Ctrl Pts',(-3.79350628097141,635.548963982637,
76.833949796622));
#100278=CARTESIAN_POINT('Ctrl Pts',(-4.5939136248181,635.784840293459,76.5485878713385));
#100279=CARTESIAN_POINT('Ctrl Pts',(-4.98575248625829,635.915952155682,
76.3857550747386));
#100280=CARTESIAN_POINT('Ctrl Pts',(-6.11412644163187,636.33040038107,75.850504898419));
#100281=CARTESIAN_POINT('Ctrl Pts',(-6.81399404095514,636.637139823021,
75.4287590544389));
#100282=CARTESIAN_POINT('Ctrl Pts',(-7.79889285265662,637.113279774517,
74.7005250396438));
#100283=CARTESIAN_POINT('Ctrl Pts',(-8.11734298004477,637.275392821193,
74.4406405058552));
#100284=CARTESIAN_POINT('Ctrl Pts',(-8.72762915407622,637.598450812687,
73.8918331418519));
#100285=CARTESIAN_POINT('Ctrl Pts',(-9.01787207664488,637.758484580972,
73.6045582479782));
#100286=CARTESIAN_POINT('Ctrl Pts',(-9.84637516857155,638.229010305788,
72.7037235931987));
#100287=CARTESIAN_POINT('Ctrl Pts',(-10.3429614399288,638.529977527531,
72.0516283531007));
#100288=CARTESIAN_POINT('Ctrl Pts',(-11.0032431948168,638.943680061139,
70.9865177450937));
#100289=CARTESIAN_POINT('Ctrl Pts',(-11.2093789343219,639.075495693331,
70.6157898317709));
#100290=CARTESIAN_POINT('Ctrl Pts',(-11.5836014028183,639.318071631035,
69.8591636321725));
#100291=CARTESIAN_POINT('Ctrl Pts',(-11.7528969072206,639.429583137573,
69.4715259668061));
#100292=CARTESIAN_POINT('Ctrl Pts',(-12.0554510123091,639.630816768811,
68.6768786107822));
#100293=CARTESIAN_POINT('Ctrl Pts',(-12.1887140449545,639.720546948354,
68.2698726655556));
#100294=CARTESIAN_POINT('Ctrl Pts',(-12.4175304640208,639.875633351266,
67.4351906357858));
#100295=CARTESIAN_POINT('Ctrl Pts',(-12.5132629458602,639.941117156214,
67.0052234510874));
#100296=CARTESIAN_POINT('Ctrl Pts',(-12.7346497723208,640.093091607933,
65.7152869175487));
#100297=CARTESIAN_POINT('Ctrl Pts',(-12.7982740854582,640.137428052,64.8470309669364));
#100298=CARTESIAN_POINT('Ctrl Pts',(-12.766112503726,640.115168111399,63.5319360416885));
#100299=CARTESIAN_POINT('Ctrl Pts',(-12.7334707525218,640.092560699991,
63.0884936792983));
#100300=CARTESIAN_POINT('Ctrl Pts',(-12.6260778331749,640.018540506094,
62.2172823473981));
#100301=CARTESIAN_POINT('Ctrl Pts',(-12.551632369959,639.967339687422,61.788489253183));
#100302=CARTESIAN_POINT('Ctrl Pts',(-12.3628457782987,639.838488032098,
60.9438749494673));
#100303=CARTESIAN_POINT('Ctrl Pts',(-12.2485007430305,639.760831558039,
60.5280554739999));
#100304=CARTESIAN_POINT('Ctrl Pts',(-11.9802058693947,639.580576882095,
59.7090936426398));
#100305=CARTESIAN_POINT('Ctrl Pts',(-11.8256357552361,639.477580968645,
59.3051045068694));
#100306=CARTESIAN_POINT('Ctrl Pts',(-11.3133789750381,639.141064503064,
58.1368724774906));
#100307=CARTESIAN_POINT('Ctrl Pts',(-10.9053335034014,638.878451769385,
57.4071299613224));
#100308=CARTESIAN_POINT('Ctrl Pts',(-10.1963986672724,638.443487632523,
56.3789236860282));
#100309=CARTESIAN_POINT('Ctrl Pts',(-9.94375223192614,638.291657307618,
56.0476855370183));
#100310=CARTESIAN_POINT('Ctrl Pts',(-9.41478615234259,637.982769203909,
55.4180596023799));
#100311=CARTESIAN_POINT('Ctrl Pts',(-9.13741954079915,637.82505037934,55.1180679858199));
#100312=CARTESIAN_POINT('Ctrl Pts',(-8.55656002383599,637.506421762877,
54.5462464538821));
#100313=CARTESIAN_POINT('Ctrl Pts',(-8.25307216483238,637.345500316042,
54.2744178365614));
#100314=CARTESIAN_POINT('Ctrl Pts',(-7.61843493119114,637.024132716943,
53.7584611953167));
#100315=CARTESIAN_POINT('Ctrl Pts',(-7.28550391450078,636.862890623527,
53.513234090336));
#100316=CARTESIAN_POINT('Ctrl Pts',(-6.25785460882906,636.394030645923,
52.8307763736279));
#100317=CARTESIAN_POINT('Ctrl Pts',(-5.53420093242913,636.100160702073,
52.4443472052227));
#100318=CARTESIAN_POINT('Ctrl Pts',(-4.37964798732873,635.718161161364,
51.9682761050355));
#100319=CARTESIAN_POINT('Ctrl Pts',(-3.98317189683697,635.600726329753,
51.8270164181643));
#100320=CARTESIAN_POINT('Ctrl Pts',(-3.16332124464332,635.392500797527,
51.5819852864849));
#100321=CARTESIAN_POINT('Ctrl Pts',(-2.73846394280183,635.301756782016,
51.478279057735));
#100322=CARTESIAN_POINT('Ctrl Pts',(-2.31092134190293,635.230245103769,
51.3976052199539));
#100323=CARTESIAN_POINT('',(2.17374032143659,634.848232285471,76.3864221483552));
#100324=CARTESIAN_POINT('Origin',(2.26224148372674,634.848232285471,76.8785273650246));
#100325=CARTESIAN_POINT('Ctrl Pts',(-3.77134412588021E-9,634.666540598395,
76.5803595180565));
#100326=CARTESIAN_POINT('Ctrl Pts',(0.346198564424135,634.66658200697,76.5804168433102));
#100327=CARTESIAN_POINT('Ctrl Pts',(0.689932235574015,634.680576584132,
76.565893487059));
#100328=CARTESIAN_POINT('Ctrl Pts',(1.03129404451953,634.707739368398,76.5371136742991));
#100329=CARTESIAN_POINT('Ctrl Pts',(1.05249997329679,634.709426762985,76.5353258273765));
#100330=CARTESIAN_POINT('Ctrl Pts',(1.07369674831757,634.711164990005,76.5334829566629));
#100331=CARTESIAN_POINT('Ctrl Pts',(1.09488439167535,634.712953867263,76.5315851371587));
#100332=CARTESIAN_POINT('Ctrl Pts',(1.43870745103581,634.741982921654,76.5007882194922));
#100333=CARTESIAN_POINT('Ctrl Pts',(1.78012200277545,634.784345579451,76.455523733084));
#100334=CARTESIAN_POINT('Ctrl Pts',(2.11922347862932,634.839287712169,76.396100987804));
#100335=CARTESIAN_POINT('Ctrl Pts',(2.13740240274387,634.842233110324,76.3929153880528));
#100336=CARTESIAN_POINT('Ctrl Pts',(2.15557467882417,634.845214672232,76.3896890929648));
#100337=CARTESIAN_POINT('Ctrl Pts',(2.17374032143659,634.848232285471,76.3864221483552));
#100338=CARTESIAN_POINT('Origin',(21.5,620.675373764374,64.2994740882088));
#100339=CARTESIAN_POINT('',(21.5,620.675373764374,44.8494740882088));
#100340=CARTESIAN_POINT('Origin',(21.5,620.675373764374,64.2994740882088));
#100341=CARTESIAN_POINT('Origin',(21.5,620.675373764374,45.3494740882088));
#100342=CARTESIAN_POINT('Origin',(-47.,620.675373764374,64.2994740882088));
#100343=CARTESIAN_POINT('',(-47.,620.675373764374,44.8494740882088));
#100344=CARTESIAN_POINT('',(-47.,620.675373764374,83.7494740882088));
#100345=CARTESIAN_POINT('Origin',(-47.,620.675373764374,64.2994740882088));
#100346=CARTESIAN_POINT('Origin',(-47.,620.675373764374,64.2994740882088));
#100347=CARTESIAN_POINT('',(-48.,620.675373764374,82.7494740882088));
#100348=CARTESIAN_POINT('Origin',(-47.,620.675373764374,82.7494740882088));
#100349=CARTESIAN_POINT('Origin',(-48.,620.675373764374,64.2994740882088));
#100350=CARTESIAN_POINT('Origin',(0.,646.549217610995,64.2994740882088));
#100351=CARTESIAN_POINT('',(-1.07343961497457E-8,606.684183939705,52.0186534989093));
#100352=CARTESIAN_POINT('Ctrl Pts',(-2.17374032143659,606.502515243277,
76.3864221483552));
#100353=CARTESIAN_POINT('Ctrl Pts',(-2.46707185687862,606.453788029884,
76.3336688327153));
#100354=CARTESIAN_POINT('Ctrl Pts',(-2.75429831334365,606.396546320481,
76.2711602395621));
#100355=CARTESIAN_POINT('Ctrl Pts',(-3.03595174524071,606.33200370037,76.1993630371087));
#100356=CARTESIAN_POINT('Ctrl Pts',(-3.32677393225283,606.265360003505,
76.1252285971402));
#100357=CARTESIAN_POINT('Ctrl Pts',(-3.61165436076205,606.190932157165,
76.0411909881563));
#100358=CARTESIAN_POINT('Ctrl Pts',(-3.89115974378405,606.110012377849,
75.9477342140385));
#100359=CARTESIAN_POINT('Ctrl Pts',(-4.05802307910513,606.061703668643,
75.8919409807596));
#100360=CARTESIAN_POINT('Ctrl Pts',(-4.22297037084448,606.011080391334,
75.8327901578527));
#100361=CARTESIAN_POINT('Ctrl Pts',(-4.38611911179911,605.958410855426,
75.7703798975853));
#100362=CARTESIAN_POINT('Ctrl Pts',(-4.42882625023245,605.944623650278,
75.7540428813797));
#100363=CARTESIAN_POINT('Ctrl Pts',(-4.4713977435419,605.93069957899,75.7374872585257));
#100364=CARTESIAN_POINT('Ctrl Pts',(-4.51383960644833,605.916642373094,
75.7207136183459));
#100365=CARTESIAN_POINT('Ctrl Pts',(-4.68077779163335,605.861350633278,
75.6547372247853));
#100366=CARTESIAN_POINT('Ctrl Pts',(-4.84590667786203,605.803892065816,
75.5852360338964));
#100367=CARTESIAN_POINT('Ctrl Pts',(-5.00922883921225,605.744546045644,
75.5122717295713));
#100368=CARTESIAN_POINT('Ctrl Pts',(-5.1452103593152,605.695134735088,75.4515218782752));
#100369=CARTESIAN_POINT('Ctrl Pts',(-5.27993934023756,605.644414219227,
75.3883704451901));
#100370=CARTESIAN_POINT('Ctrl Pts',(-5.41340686872785,605.592533100018,
75.3228309779361));
#100371=CARTESIAN_POINT('Ctrl Pts',(-5.4767325267563,605.567917329798,75.2917348009286));
#100372=CARTESIAN_POINT('Ctrl Pts',(-5.53988672272686,605.542995856186,
75.2600451580777));
#100373=CARTESIAN_POINT('Ctrl Pts',(-5.60282655347565,605.517797003193,
75.2277765641491));
#100374=CARTESIAN_POINT('Ctrl Pts',(-5.74446489104482,605.461090087969,
75.1551600676419));
#100375=CARTESIAN_POINT('Ctrl Pts',(-5.88451794386309,605.403194028895,
75.0798887530446));
#100376=CARTESIAN_POINT('Ctrl Pts',(-6.02277650795407,605.344367506919,
75.00208867691));
#100377=CARTESIAN_POINT('Ctrl Pts',(-6.14763311325176,605.291243276361,
74.9318300751233));
#100378=CARTESIAN_POINT('Ctrl Pts',(-6.27102683838747,605.237360714913,
74.8595096788036));
#100379=CARTESIAN_POINT('Ctrl Pts',(-6.39282729924325,605.18292181379,74.7852455842724));
#100380=CARTESIAN_POINT('Ctrl Pts',(-6.47083494811976,605.148056176549,
74.7376828134124));
#100381=CARTESIAN_POINT('Ctrl Pts',(-6.54814400546939,605.112980745157,
74.6893515147672));
#100382=CARTESIAN_POINT('Ctrl Pts',(-6.62477499791199,605.07772814186,74.6402582278617));
#100383=CARTESIAN_POINT('Ctrl Pts',(-6.96478303205049,604.921314033637,
74.4224336710075));
#100384=CARTESIAN_POINT('Ctrl Pts',(-7.29157363628114,604.761467878279,
74.1897538732292));
#100385=CARTESIAN_POINT('Ctrl Pts',(-7.60591158708235,604.600369471168,
73.9417908300559));
#100386=CARTESIAN_POINT('Ctrl Pts',(-7.79580795695568,604.503047456359,
73.7919925583507));
#100387=CARTESIAN_POINT('Ctrl Pts',(-7.98115910169857,604.405267574512,
73.6366162396827));
#100388=CARTESIAN_POINT('Ctrl Pts',(-8.16212832796301,604.307503591966,
73.4755645439775));
#100389=CARTESIAN_POINT('Ctrl Pts',(-8.26136891658198,604.253891409531,
73.3872464060831));
#100390=CARTESIAN_POINT('Ctrl Pts',(-8.35931409671926,604.200262850107,
73.2972012703487));
#100391=CARTESIAN_POINT('Ctrl Pts',(-8.45597459854735,604.146704981741,
73.2054245700201));
#100392=CARTESIAN_POINT('Ctrl Pts',(-8.62621244832271,604.052379210854,
73.0437880398146));
#100393=CARTESIAN_POINT('Ctrl Pts',(-8.79257116956151,603.95814323677,72.8764594849325));
#100394=CARTESIAN_POINT('Ctrl Pts',(-8.95390631633433,603.865073190674,
72.704606310153));
#100395=CARTESIAN_POINT('Ctrl Pts',(-9.06095118698477,603.803321791521,
72.5905827930637));
#100396=CARTESIAN_POINT('Ctrl Pts',(-9.16584077110249,603.742048678356,
72.4745092679943));
#100397=CARTESIAN_POINT('Ctrl Pts',(-9.26827482729216,603.681541731399,
72.3566784495144));
#100398=CARTESIAN_POINT('Ctrl Pts',(-9.40788641074879,603.599074327598,
72.1960819861906));
#100399=CARTESIAN_POINT('Ctrl Pts',(-9.54330408966463,603.517830454451,
72.0319079775284));
#100400=CARTESIAN_POINT('Ctrl Pts',(-9.67458462015739,603.438025868564,
71.8640057896189));
#100401=CARTESIAN_POINT('Ctrl Pts',(-9.78480582545456,603.371023110335,
71.7230375786134));
#100402=CARTESIAN_POINT('Ctrl Pts',(-9.89203337317964,603.305082450115,
71.5795402257765));
#100403=CARTESIAN_POINT('Ctrl Pts',(-9.99631546020291,603.240324463723,
71.4334167298244));
#100404=CARTESIAN_POINT('Ctrl Pts',(-10.1466411918896,603.146973899259,
71.2227753620435));
#100405=CARTESIAN_POINT('Ctrl Pts',(-10.2908485193802,603.056075593346,
71.0066806945939));
#100406=CARTESIAN_POINT('Ctrl Pts',(-10.4288865117607,602.968017132758,
70.784690190237));
#100407=CARTESIAN_POINT('Ctrl Pts',(-10.5005094876998,602.922326747849,
70.6695072592333));
#100408=CARTESIAN_POINT('Ctrl Pts',(-10.5704709864211,602.877401174178,
70.5527365289386));
#100409=CARTESIAN_POINT('Ctrl Pts',(-10.6387601151285,602.83329660101,70.4343126036391));
#100410=CARTESIAN_POINT('Ctrl Pts',(-10.724621663596,602.777842870403,70.2854153809878));
#100411=CARTESIAN_POINT('Ctrl Pts',(-10.8079009366217,602.723642207191,
70.1336854355193));
#100412=CARTESIAN_POINT('Ctrl Pts',(-10.888241259658,602.671014635769,69.9796674430985));
#100413=CARTESIAN_POINT('Ctrl Pts',(-10.9945530515871,602.601374245846,
69.7758603367196));
#100414=CARTESIAN_POINT('Ctrl Pts',(-11.0954755518842,602.534655054501,
69.5685147915909));
#100415=CARTESIAN_POINT('Ctrl Pts',(-11.1902371419611,602.471566104083,
69.3589259475648));
#100416=CARTESIAN_POINT('Ctrl Pts',(-11.300099218997,602.3984237779,69.1159386178927));
#100417=CARTESIAN_POINT('Ctrl Pts',(-11.4021973889724,602.329852464716,
68.869301471737));
#100418=CARTESIAN_POINT('Ctrl Pts',(-11.4964066628775,602.266152746647,
68.6186837688837));
#100419=CARTESIAN_POINT('Ctrl Pts',(-11.5906159367827,602.202453028578,
68.3680660660304));
#100420=CARTESIAN_POINT('Ctrl Pts',(-11.6769365272855,602.143624555107,
68.1134679693462));
#100421=CARTESIAN_POINT('Ctrl Pts',(-11.7551965015822,602.089998067109,
67.8545346302323));
#100422=CARTESIAN_POINT('Ctrl Pts',(-11.8169098336505,602.047709920566,
67.6503480165271));
#100423=CARTESIAN_POINT('Ctrl Pts',(-11.8735597973911,602.008694644865,
67.4436368914992));
#100424=CARTESIAN_POINT('Ctrl Pts',(-11.9250862572614,601.973096443384,
67.2341237558232));
#100425=CARTESIAN_POINT('Ctrl Pts',(-11.9407583946926,601.962268998469,
67.1703988528467));
#100426=CARTESIAN_POINT('Ctrl Pts',(-11.9559562743235,601.951757858935,
67.1064145882828));
#100427=CARTESIAN_POINT('Ctrl Pts',(-11.9706774739931,601.941567587219,
67.0421627707268));
#100428=CARTESIAN_POINT('Ctrl Pts',(-11.9954037307114,601.924451640141,
66.9342431058105));
#100429=CARTESIAN_POINT('Ctrl Pts',(-12.018712244929,601.908287348004,66.8257413548535));
#100430=CARTESIAN_POINT('Ctrl Pts',(-12.0405781026576,601.893099709119,
66.716775352046));
#100431=CARTESIAN_POINT('Ctrl Pts',(-12.0731127727702,601.870501701438,
66.5546425421266));
#100432=CARTESIAN_POINT('Ctrl Pts',(-12.1023388533522,601.850161851815,
66.3920691391728));
#100433=CARTESIAN_POINT('Ctrl Pts',(-12.1282540008843,601.832100855068,
66.2292774714516));
#100434=CARTESIAN_POINT('Ctrl Pts',(-12.1502877690817,601.816744900979,
66.0908675370076));
#100435=CARTESIAN_POINT('Ctrl Pts',(-12.1699275035384,601.803036685216,
65.9522990545189));
#100436=CARTESIAN_POINT('Ctrl Pts',(-12.1871477917995,601.79100539956,65.8137029664605));
#100437=CARTESIAN_POINT('Ctrl Pts',(-12.1980348631784,601.783398937709,
65.7260792588519));
#100438=CARTESIAN_POINT('Ctrl Pts',(-12.2079791265231,601.776445852263,
65.6383428164895));
#100439=CARTESIAN_POINT('Ctrl Pts',(-12.2169811144402,601.770146217632,
65.5504516908381));
#100440=CARTESIAN_POINT('Ctrl Pts',(-12.2439507747706,601.751272719049,
65.2871327632072));
#100441=CARTESIAN_POINT('Ctrl Pts',(-12.262381938816,601.738341021169,65.0232227696719));
#100442=CARTESIAN_POINT('Ctrl Pts',(-12.2722764759267,601.731396026852,
64.758554127766));
#100443=CARTESIAN_POINT('Ctrl Pts',(-12.2745803436584,601.729778937733,
64.6969280469448));
#100444=CARTESIAN_POINT('Ctrl Pts',(-12.2764212110178,601.72848654818,64.6352608197646));
#100445=CARTESIAN_POINT('Ctrl Pts',(-12.2777987694388,601.727519657373,
64.5735503018836));
#100446=CARTESIAN_POINT('Ctrl Pts',(-12.2836252561778,601.723430120131,
64.3125410346233));
#100447=CARTESIAN_POINT('Ctrl Pts',(-12.2811683166638,601.725160388178,
64.0507577357569));
#100448=CARTESIAN_POINT('Ctrl Pts',(-12.2702125553129,601.732843354971,
63.7880240573192));
#100449=CARTESIAN_POINT('Ctrl Pts',(-12.2637572833743,601.737370255326,
63.6332180801329));
#100450=CARTESIAN_POINT('Ctrl Pts',(-12.254350682346,601.743964308948,63.4780820905828));
#100451=CARTESIAN_POINT('Ctrl Pts',(-12.2419417245922,601.752657551092,
63.322579412737));
#100452=CARTESIAN_POINT('Ctrl Pts',(-12.2383613410484,601.755165831137,
63.27771188721));
#100453=CARTESIAN_POINT('Ctrl Pts',(-12.2345355379089,601.757845659036,
63.2328883365077));
#100454=CARTESIAN_POINT('Ctrl Pts',(-12.2304658136691,601.760695594299,
63.1881120965528));
#100455=CARTESIAN_POINT('Ctrl Pts',(-12.20802985293,601.77640698699,62.9412654056049));
#100456=CARTESIAN_POINT('Ctrl Pts',(-12.1782497081193,601.797243520989,
62.6965771340082));
#100457=CARTESIAN_POINT('Ctrl Pts',(-12.1414782088463,601.822892192644,
62.4545441951047));
#100458=CARTESIAN_POINT('Ctrl Pts',(-12.1225673535514,601.836082797536,
62.3300714383586));
#100459=CARTESIAN_POINT('Ctrl Pts',(-12.1018066819712,601.850546650797,
62.2063009544923));
#100460=CARTESIAN_POINT('Ctrl Pts',(-12.0792398615636,601.866244252266,
62.083300637742));
#100461=CARTESIAN_POINT('Ctrl Pts',(-12.0338392047362,601.897825192977,
61.8358446350983));
#100462=CARTESIAN_POINT('Ctrl Pts',(-11.9810913904904,601.934449474634,
61.5908900513811));
#100463=CARTESIAN_POINT('Ctrl Pts',(-11.9210791903706,601.975905237726,
61.3483598142781));
#100464=CARTESIAN_POINT('Ctrl Pts',(-11.8825771448038,602.002502024319,
61.1927596159579));
#100465=CARTESIAN_POINT('Ctrl Pts',(-11.8410841234437,602.031088120635,
61.0381575576643));
#100466=CARTESIAN_POINT('Ctrl Pts',(-11.7966129422133,602.061613620413,
60.8845362018886));
#100467=CARTESIAN_POINT('Ctrl Pts',(-11.7145024730305,602.117975134532,
60.6008935989656));
#100468=CARTESIAN_POINT('Ctrl Pts',(-11.622240048691,602.180950916266,60.3206183352987));
#100469=CARTESIAN_POINT('Ctrl Pts',(-11.5200358747597,602.250140176206,
60.0440321693328));
#100470=CARTESIAN_POINT('Ctrl Pts',(-11.4804847370665,602.27691514871,59.9369984043372));
#100471=CARTESIAN_POINT('Ctrl Pts',(-11.4394452245149,602.304620325316,
59.8305169440055));
#100472=CARTESIAN_POINT('Ctrl Pts',(-11.3969311992182,602.333231415316,
59.7246058240927));
#100473=CARTESIAN_POINT('Ctrl Pts',(-11.2825177403899,602.410229388217,
59.4395785307927));
#100474=CARTESIAN_POINT('Ctrl Pts',(-11.158988431834,602.492725506564,59.1623611802148));
#100475=CARTESIAN_POINT('Ctrl Pts',(-11.0267821846615,602.579993779557,
58.8926332895343));
#100476=CARTESIAN_POINT('Ctrl Pts',(-11.0022967669809,602.596156405455,
58.8426780097752));
#100477=CARTESIAN_POINT('Ctrl Pts',(-10.9775138237409,602.612482671629,
58.7929795440708));
#100478=CARTESIAN_POINT('Ctrl Pts',(-10.9524362839605,602.628967901316,
58.7435357446885));
#100479=CARTESIAN_POINT('Ctrl Pts',(-10.7519969306551,602.760730777836,
58.3483421467532));
#100480=CARTESIAN_POINT('Ctrl Pts',(-10.5325668032455,602.902760978284,
57.9690756449635));
#100481=CARTESIAN_POINT('Ctrl Pts',(-10.2952739748061,603.052908390917,
57.6041926021618));
#100482=CARTESIAN_POINT('Ctrl Pts',(-10.1290947826627,603.15805853767,57.3486603567147));
#100483=CARTESIAN_POINT('Ctrl Pts',(-9.95405618215907,603.267227434755,
57.1002579207061));
#100484=CARTESIAN_POINT('Ctrl Pts',(-9.77011972363466,603.379759886329,
56.8587519976395));
#100485=CARTESIAN_POINT('Ctrl Pts',(-9.71724352583042,603.412109580438,
56.7893263108485));
#100486=CARTESIAN_POINT('Ctrl Pts',(-9.66363239874421,603.444736981392,
56.720471086118));
#100487=CARTESIAN_POINT('Ctrl Pts',(-9.60928507234348,603.477626699899,
56.6521803974868));
#100488=CARTESIAN_POINT('Ctrl Pts',(-9.36573391882352,603.625018106469,
56.3461437054854));
#100489=CARTESIAN_POINT('Ctrl Pts',(-9.10609991920284,603.778422086477,
56.0501477801115));
#100490=CARTESIAN_POINT('Ctrl Pts',(-8.83441059956637,603.93369250988,55.7687853847948));
#100491=CARTESIAN_POINT('Ctrl Pts',(-8.65468490819934,604.036405727434,
55.5826608397055));
#100492=CARTESIAN_POINT('Ctrl Pts',(-8.47006004966758,604.139793805599,
55.4030725521529));
#100493=CARTESIAN_POINT('Ctrl Pts',(-8.28039538035885,604.243327157586,
55.2298442866972));
#100494=CARTESIAN_POINT('Ctrl Pts',(-7.9890388931648,604.402371611421,54.9637368504001));
#100495=CARTESIAN_POINT('Ctrl Pts',(-7.68586832487023,604.561762715034,
54.7127055606849));
#100496=CARTESIAN_POINT('Ctrl Pts',(-7.37033208730518,604.71958124259,54.4760819004763));
#100497=CARTESIAN_POINT('Ctrl Pts',(-7.2700391143498,604.769743751461,54.4008712351751));
#100498=CARTESIAN_POINT('Ctrl Pts',(-7.16849659991518,604.819747365336,
54.3271164420992));
#100499=CARTESIAN_POINT('Ctrl Pts',(-7.06568610310642,604.869530328493,
54.25479687612));
#100500=CARTESIAN_POINT('Ctrl Pts',(-6.89206181747092,604.953602788829,
54.1326650571874));
#100501=CARTESIAN_POINT('Ctrl Pts',(-6.71445450113538,605.037163623483,
54.014541313487));
#100502=CARTESIAN_POINT('Ctrl Pts',(-6.53323952933694,605.119585952013,
53.9007405871998));
#100503=CARTESIAN_POINT('Ctrl Pts',(-6.39148708172352,605.184059470349,
53.8117218304641));
#100504=CARTESIAN_POINT('Ctrl Pts',(-6.24726996399549,605.247955635443,
53.7251920165717));
#100505=CARTESIAN_POINT('Ctrl Pts',(-6.1010333037784,605.310847708287,53.6414835032615));
#100506=CARTESIAN_POINT('Ctrl Pts',(-5.9575052790118,605.372574876943,53.5593254619487));
#100507=CARTESIAN_POINT('Ctrl Pts',(-5.81203236066972,605.433334144939,
53.4798854136267));
#100508=CARTESIAN_POINT('Ctrl Pts',(-5.66506348803577,605.492735683132,
53.4034385207339));
#100509=CARTESIAN_POINT('Ctrl Pts',(-5.63106986886025,605.506475145316,
53.3857565006055));
#100510=CARTESIAN_POINT('Ctrl Pts',(-5.59699631957295,605.520142052501,
53.3682344347307));
#100511=CARTESIAN_POINT('Ctrl Pts',(-5.56284856908302,605.533731743956,
53.3508754028169));
#100512=CARTESIAN_POINT('Ctrl Pts',(-5.38268096900712,605.6054325752,53.2592870822194));
#100513=CARTESIAN_POINT('Ctrl Pts',(-5.19987034695042,605.675213610825,
53.1719434243341));
#100514=CARTESIAN_POINT('Ctrl Pts',(-5.01474362923014,605.742546333116,
53.0891303500769));
#100515=CARTESIAN_POINT('Ctrl Pts',(-4.85852202040101,605.799365933943,
53.0192474512071));
#100516=CARTESIAN_POINT('Ctrl Pts',(-4.70043407277484,605.854543653029,
52.9524335003881));
#100517=CARTESIAN_POINT('Ctrl Pts',(-4.54038793193478,605.90783958427,52.8887479043086));
#100518=CARTESIAN_POINT('Ctrl Pts',(-4.32988395211606,605.977938154442,
52.8049841136825));
#100519=CARTESIAN_POINT('Ctrl Pts',(-4.11606910507959,606.044759266673,
52.7266642081674));
#100520=CARTESIAN_POINT('Ctrl Pts',(-3.89880804431973,606.107740093685,
52.6539274618112));
#100521=CARTESIAN_POINT('Ctrl Pts',(-3.75513870481496,606.149387749213,
52.6058284593017));
#100522=CARTESIAN_POINT('Ctrl Pts',(-3.60957076508887,606.189429699183,
52.5600901866311));
#100523=CARTESIAN_POINT('Ctrl Pts',(-3.46260051940716,606.227568994084,
52.5169114539341));
#100524=CARTESIAN_POINT('Ctrl Pts',(-3.30083889264099,606.269546704321,
52.4693871267455));
#100525=CARTESIAN_POINT('Ctrl Pts',(-3.13696220030451,606.309325226518,
52.4248444109981));
#100526=CARTESIAN_POINT('Ctrl Pts',(-2.97184384013739,606.346433279838,
52.3836415514574));
#100527=CARTESIAN_POINT('Ctrl Pts',(-2.88817958080778,606.365235657679,
52.3627643654059));
#100528=CARTESIAN_POINT('Ctrl Pts',(-2.8041970333705,606.383352786247,52.3427440958518));
#100529=CARTESIAN_POINT('Ctrl Pts',(-2.72001197855735,606.400726128442,
52.3236235868221));
#100530=CARTESIAN_POINT('Ctrl Pts',(-2.59111236083403,606.427327253457,
52.2943472941348));
#100531=CARTESIAN_POINT('Ctrl Pts',(-2.46182005847151,606.452184037893,
52.2671471808491));
#100532=CARTESIAN_POINT('Ctrl Pts',(-2.33225003338043,606.475224241091,
52.2420568539227));
#100533=CARTESIAN_POINT('Ctrl Pts',(-2.02166802222565,606.530452081339,
52.181914824994));
#100534=CARTESIAN_POINT('Ctrl Pts',(-1.70858199877496,606.575372497744,
52.1337147382732));
#100535=CARTESIAN_POINT('Ctrl Pts',(-1.39302211019354,606.609207737378,
52.0977046786308));
#100536=CARTESIAN_POINT('Ctrl Pts',(-1.08056553839342,606.642710230454,
52.0620487534219));
#100537=CARTESIAN_POINT('Ctrl Pts',(-0.765683584542685,606.665344269887,
52.0383441545844));
#100538=CARTESIAN_POINT('Ctrl Pts',(-0.448405337689409,606.676388629552,
52.0267929415551));
#100539=CARTESIAN_POINT('Ctrl Pts',(-0.388670115536972,606.678467994541,
52.0246181492923));
#100540=CARTESIAN_POINT('Ctrl Pts',(-0.328849950036206,606.680136641758,
52.0228740510578));
#100541=CARTESIAN_POINT('Ctrl Pts',(-0.268945032176679,606.681389902202,
52.021561847169));
#100542=CARTESIAN_POINT('Ctrl Pts',(-0.17955506691534,606.683260014231,
52.0196037798813));
#100543=CARTESIAN_POINT('Ctrl Pts',(-0.0898586837202595,606.684188838802,
52.0186356114588));
#100544=CARTESIAN_POINT('Ctrl Pts',(-1.0734396260768E-8,606.684183939704,
52.0186534989093));
#100545=CARTESIAN_POINT('',(1.07518174918924E-8,634.666563589043,52.0186534989093));
#100546=CARTESIAN_POINT('',(-1.50397128011561E-15,646.549217610995,52.018616610259));
#100547=CARTESIAN_POINT('Ctrl Pts',(2.24521812585737E-14,634.666520326694,
52.018616610259));
#100548=CARTESIAN_POINT('Ctrl Pts',(-0.373817003726286,634.666520326694,
52.018616610259));
#100549=CARTESIAN_POINT('Ctrl Pts',(-0.751201067837897,634.68307764615,
52.0359697011552));
#100550=CARTESIAN_POINT('Ctrl Pts',(-1.49208745862324,634.747185279649,
52.1039208858558));
#100551=CARTESIAN_POINT('Ctrl Pts',(-1.8582948677369,634.794652262569,52.1544405788509));
#100552=CARTESIAN_POINT('Ctrl Pts',(-2.22051577456844,634.856083886813,
52.2210317180765));
#100553=CARTESIAN_POINT('Ctrl Pts',(2.17374032143659,634.848232285471,76.3864221483552));
#100554=CARTESIAN_POINT('Ctrl Pts',(2.46707185688744,634.896959498865,76.3336688327137));
#100555=CARTESIAN_POINT('Ctrl Pts',(2.75429831336094,634.95420120827,76.2711602395584));
#100556=CARTESIAN_POINT('Ctrl Pts',(3.03595174526615,635.018743828384,76.1993630371022));
#100557=CARTESIAN_POINT('Ctrl Pts',(3.32677393228709,635.085387525251,76.1252285971308));
#100558=CARTESIAN_POINT('Ctrl Pts',(3.61165436080482,635.159815371594,76.0411909881434));
#100559=CARTESIAN_POINT('Ctrl Pts',(3.89115974383501,635.240735150913,75.9477342140214));
#100560=CARTESIAN_POINT('Ctrl Pts',(4.05802307913842,635.289043860115,75.8919409807476));
#100561=CARTESIAN_POINT('Ctrl Pts',(4.22297037086047,635.339667137419,75.8327901578465));
#100562=CARTESIAN_POINT('Ctrl Pts',(4.3861191117982,635.392336673321,75.7703798975857));
#100563=CARTESIAN_POINT('Ctrl Pts',(4.42882625023184,635.40612387847,75.7540428813799));
#100564=CARTESIAN_POINT('Ctrl Pts',(4.47139774354158,635.420047949757,75.7374872585258));
#100565=CARTESIAN_POINT('Ctrl Pts',(4.5138396064483,635.434105155654,75.7207136183459));
#100566=CARTESIAN_POINT('Ctrl Pts',(4.68077779162843,635.489396895468,75.6547372247873));
#100567=CARTESIAN_POINT('Ctrl Pts',(4.84590667785229,635.546855462928,75.5852360339005));
#100568=CARTESIAN_POINT('Ctrl Pts',(5.00922883919779,635.606201483099,75.5122717295777));
#100569=CARTESIAN_POINT('Ctrl Pts',(5.14521035930517,635.655612793656,75.4515218782799));
#100570=CARTESIAN_POINT('Ctrl Pts',(5.27993934023189,635.706333309519,75.3883704451929));
#100571=CARTESIAN_POINT('Ctrl Pts',(5.41340686872647,635.758214428729,75.3228309779368));
#100572=CARTESIAN_POINT('Ctrl Pts',(5.47673252675539,635.782830198949,75.2917348009291));
#100573=CARTESIAN_POINT('Ctrl Pts',(5.53988672272641,635.807751672561,75.2600451580779));
#100574=CARTESIAN_POINT('Ctrl Pts',(5.60282655347567,635.832950525554,75.2277765641491));
#100575=CARTESIAN_POINT('Ctrl Pts',(5.74446489104563,635.889657440779,75.1551600676415));
#100576=CARTESIAN_POINT('Ctrl Pts',(5.88451794386466,635.947553499853,75.0798887530437));
#100577=CARTESIAN_POINT('Ctrl Pts',(6.02277650795639,636.00638002183,75.0020886769087));
#100578=CARTESIAN_POINT('Ctrl Pts',(6.1476331132527,636.059504252387,74.9318300751227));
#100579=CARTESIAN_POINT('Ctrl Pts',(6.27102683838704,636.113386813834,74.8595096788039));
#100580=CARTESIAN_POINT('Ctrl Pts',(6.39282729924149,636.167825714957,74.7852455842735));
#100581=CARTESIAN_POINT('Ctrl Pts',(6.4708349481186,636.202691352198,74.7376828134132));
#100582=CARTESIAN_POINT('Ctrl Pts',(6.54814400546881,636.23776678359,74.6893515147675));
#100583=CARTESIAN_POINT('Ctrl Pts',(6.62477499791198,636.273019386888,74.6402582278617));
#100584=CARTESIAN_POINT('Ctrl Pts',(6.96478303207395,636.429433495122,74.4224336709924));
#100585=CARTESIAN_POINT('Ctrl Pts',(7.29157363632626,636.589279650491,74.1897538731971));
#100586=CARTESIAN_POINT('Ctrl Pts',(7.60591158714745,636.750378057613,73.9417908300045));
#100587=CARTESIAN_POINT('Ctrl Pts',(7.79580795699725,636.84770007241,73.7919925583159));
#100588=CARTESIAN_POINT('Ctrl Pts',(7.98115910171771,636.945479954246,73.6366162396656));
#100589=CARTESIAN_POINT('Ctrl Pts',(8.16212832796075,637.04324393678,73.4755645439795));
#100590=CARTESIAN_POINT('Ctrl Pts',(8.26136891658048,637.096856119215,73.3872464060845));
#100591=CARTESIAN_POINT('Ctrl Pts',(8.35931409671852,637.15048467864,73.2972012703495));
#100592=CARTESIAN_POINT('Ctrl Pts',(8.45597459854733,637.204042547007,73.2054245700202));
#100593=CARTESIAN_POINT('Ctrl Pts',(8.62621244832184,637.298368317893,73.0437880398154));
#100594=CARTESIAN_POINT('Ctrl Pts',(8.79257116955984,637.392604291977,72.8764594849342));
#100595=CARTESIAN_POINT('Ctrl Pts',(8.95390631633191,637.485674338072,72.7046063101555));
#100596=CARTESIAN_POINT('Ctrl Pts',(9.06095118698319,637.547425737225,72.5905827930654));
#100597=CARTESIAN_POINT('Ctrl Pts',(9.16584077110172,637.608698850392,72.4745092679952));
#100598=CARTESIAN_POINT('Ctrl Pts',(9.26827482729214,637.669205797348,72.3566784495144));
#100599=CARTESIAN_POINT('Ctrl Pts',(9.4078864107479,637.751673201148,72.1960819861916));
#100600=CARTESIAN_POINT('Ctrl Pts',(9.5433040896629,637.832917074295,72.0319079775306));
#100601=CARTESIAN_POINT('Ctrl Pts',(9.67458462015488,637.912721660182,71.8640057896221));
#100602=CARTESIAN_POINT('Ctrl Pts',(9.78480582545293,637.979724418411,71.7230375786156));
#100603=CARTESIAN_POINT('Ctrl Pts',(9.89203337317883,638.045665078632,71.5795402257776));
#100604=CARTESIAN_POINT('Ctrl Pts',(9.99631546020288,638.110423065025,71.4334167298244));
#100605=CARTESIAN_POINT('Ctrl Pts',(10.1466411918942,638.203773629491,71.2227753620371));
#100606=CARTESIAN_POINT('Ctrl Pts',(10.290848519389,638.294671935407,71.0066806945808));
#100607=CARTESIAN_POINT('Ctrl Pts',(10.4288865117733,638.382730395997,70.7846901902168));
#100608=CARTESIAN_POINT('Ctrl Pts',(10.500509487708,638.428420780904,70.6695072592196));
#100609=CARTESIAN_POINT('Ctrl Pts',(10.570470986425,638.473346354573,70.5527365289317));
#100610=CARTESIAN_POINT('Ctrl Pts',(10.6387601151285,638.517450927738,70.4343126036392));
#100611=CARTESIAN_POINT('Ctrl Pts',(10.7246216635952,638.572904658344,70.2854153809893));
#100612=CARTESIAN_POINT('Ctrl Pts',(10.80790093662,638.627105321556,70.1336854355224));
#100613=CARTESIAN_POINT('Ctrl Pts',(10.8882412596556,638.679732892978,69.9796674431032));
#100614=CARTESIAN_POINT('Ctrl Pts',(10.9945530515856,638.749373282901,69.7758603367227));
#100615=CARTESIAN_POINT('Ctrl Pts',(11.0954755518835,638.816092474246,69.5685147915925));
#100616=CARTESIAN_POINT('Ctrl Pts',(11.1902371419611,638.879181424665,69.3589259475647));
#100617=CARTESIAN_POINT('Ctrl Pts',(11.3000992189965,638.952323750847,69.1159386178936));
#100618=CARTESIAN_POINT('Ctrl Pts',(11.4021973889716,639.020895064031,68.869301471739));
#100619=CARTESIAN_POINT('Ctrl Pts',(11.4964066628764,639.0845947821,68.6186837688867));
#100620=CARTESIAN_POINT('Ctrl Pts',(11.5906159367812,639.148294500168,68.3680660660344));
#100621=CARTESIAN_POINT('Ctrl Pts',(11.6769365272838,639.207122973639,68.1134679693512));
#100622=CARTESIAN_POINT('Ctrl Pts',(11.7551965015803,639.260749461637,67.8545346302384));
#100623=CARTESIAN_POINT('Ctrl Pts',(11.8169098336493,639.30303760818,67.6503480165316));
#100624=CARTESIAN_POINT('Ctrl Pts',(11.8735597973904,639.342052883881,67.443636891502));
#100625=CARTESIAN_POINT('Ctrl Pts',(11.9250862572612,639.377651085363,67.2341237558242));
#100626=CARTESIAN_POINT('Ctrl Pts',(11.9407583946925,639.388478530278,67.1703988528473));
#100627=CARTESIAN_POINT('Ctrl Pts',(11.9559562743234,639.398989669813,67.1064145882831));
#100628=CARTESIAN_POINT('Ctrl Pts',(11.9706774739931,639.409179941528,67.0421627707268));
#100629=CARTESIAN_POINT('Ctrl Pts',(11.9954037307109,639.426295888606,66.9342431058128));
#100630=CARTESIAN_POINT('Ctrl Pts',(12.018712244928,639.442460180743,66.8257413548581));
#100631=CARTESIAN_POINT('Ctrl Pts',(12.0405781026562,639.457647819627,66.7167753520528));
#100632=CARTESIAN_POINT('Ctrl Pts',(12.0731127727685,639.480245827309,66.5546425421351));
#100633=CARTESIAN_POINT('Ctrl Pts',(12.1023388533504,639.500585676932,66.3920691391829));
#100634=CARTESIAN_POINT('Ctrl Pts',(12.1282540008825,639.518646673678,66.2292774714633));
#100635=CARTESIAN_POINT('Ctrl Pts',(12.1502877690806,639.534002627768,66.0908675370154));
#100636=CARTESIAN_POINT('Ctrl Pts',(12.169927503538,639.547710843531,65.9522990545228));
#100637=CARTESIAN_POINT('Ctrl Pts',(12.1871477917995,639.559742129188,65.8137029664605));
#100638=CARTESIAN_POINT('Ctrl Pts',(12.1980348631781,639.567348591038,65.7260792588543));
#100639=CARTESIAN_POINT('Ctrl Pts',(12.2079791265226,639.574301676484,65.6383428164945));
#100640=CARTESIAN_POINT('Ctrl Pts',(12.2169811144395,639.580601311115,65.5504516908455));
#100641=CARTESIAN_POINT('Ctrl Pts',(12.2439507747694,639.599474809698,65.2871327632205));
#100642=CARTESIAN_POINT('Ctrl Pts',(12.2623819388147,639.612406507578,65.023222769691));
#100643=CARTESIAN_POINT('Ctrl Pts',(12.2722764759257,639.619351501895,64.758554127791));
#100644=CARTESIAN_POINT('Ctrl Pts',(12.2745803436579,639.620968591014,64.6969280469615));
#100645=CARTESIAN_POINT('Ctrl Pts',(12.2764212110176,639.622260980568,64.6352608197729));
#100646=CARTESIAN_POINT('Ctrl Pts',(12.2777987694388,639.623227871375,64.5735503018836));
#100647=CARTESIAN_POINT('Ctrl Pts',(12.2836252561777,639.627317408616,64.3125410346274));
#100648=CARTESIAN_POINT('Ctrl Pts',(12.2811683166639,639.625587140569,64.0507577357652));
#100649=CARTESIAN_POINT('Ctrl Pts',(12.2702125553135,639.617904173777,63.7880240573317));
#100650=CARTESIAN_POINT('Ctrl Pts',(12.2637572833749,639.613377273422,63.6332180801413));
#100651=CARTESIAN_POINT('Ctrl Pts',(12.2543506823463,639.6067832198,63.478082090587));
#100652=CARTESIAN_POINT('Ctrl Pts',(12.2419417245922,639.598089977656,63.322579412737));
#100653=CARTESIAN_POINT('Ctrl Pts',(12.2383613410486,639.595581697611,63.2777118872129));
#100654=CARTESIAN_POINT('Ctrl Pts',(12.2345355379094,639.592901869712,63.2328883365136));
#100655=CARTESIAN_POINT('Ctrl Pts',(12.2304658136699,639.590051934449,63.1881120965615));
#100656=CARTESIAN_POINT('Ctrl Pts',(12.2080298529311,639.574340541758,62.9412654056156));
#100657=CARTESIAN_POINT('Ctrl Pts',(12.1782497081209,639.55350400776,62.6965771340207));
#100658=CARTESIAN_POINT('Ctrl Pts',(12.1414782088484,639.527855336105,62.454544195119));
#100659=CARTESIAN_POINT('Ctrl Pts',(12.122567353553,639.514664731212,62.3300714383681));
#100660=CARTESIAN_POINT('Ctrl Pts',(12.1018066819721,639.500200877951,62.206300954497));
#100661=CARTESIAN_POINT('Ctrl Pts',(12.0792398615636,639.484503276481,62.0833006377421));
#100662=CARTESIAN_POINT('Ctrl Pts',(12.0338392047365,639.452922335771,61.8358446351003));
#100663=CARTESIAN_POINT('Ctrl Pts',(11.9810913904912,639.416298054115,61.590890051385));
#100664=CARTESIAN_POINT('Ctrl Pts',(11.921079190372,639.374842291023,61.3483598142839));
#100665=CARTESIAN_POINT('Ctrl Pts',(11.8825771448056,639.34824550443,61.1927596159649));
#100666=CARTESIAN_POINT('Ctrl Pts',(11.8410841234459,639.319659408115,61.0381575576725));
#100667=CARTESIAN_POINT('Ctrl Pts',(11.796612942216,639.289133908337,60.8845362018978));
#100668=CARTESIAN_POINT('Ctrl Pts',(11.7145024730303,639.232772394216,60.600893598964));
#100669=CARTESIAN_POINT('Ctrl Pts',(11.6222400486871,639.169796612479,60.3206183352867));
#100670=CARTESIAN_POINT('Ctrl Pts',(11.5200358747514,639.100607352536,60.0440321693105));
#100671=CARTESIAN_POINT('Ctrl Pts',(11.4804847370608,639.073832380033,59.9369984043224));
#100672=CARTESIAN_POINT('Ctrl Pts',(11.439445224512,639.046127203429,59.8305169439982));
#100673=CARTESIAN_POINT('Ctrl Pts',(11.3969311992182,639.017516113431,59.7246058240927));
#100674=CARTESIAN_POINT('Ctrl Pts',(11.2825177403853,638.940518140527,59.4395785307811));
#100675=CARTESIAN_POINT('Ctrl Pts',(11.158988431824,638.858022022176,59.1623611801923));
#100676=CARTESIAN_POINT('Ctrl Pts',(11.0267821846454,638.77075374918,58.8926332895015));
#100677=CARTESIAN_POINT('Ctrl Pts',(11.0022967669716,638.754591123286,58.8426780097566));
#100678=CARTESIAN_POINT('Ctrl Pts',(10.9775138237385,638.738264857117,58.7929795440662));
#100679=CARTESIAN_POINT('Ctrl Pts',(10.9524362839652,638.721779627435,58.7435357446977));
#100680=CARTESIAN_POINT('Ctrl Pts',(10.7519969306585,638.590016750914,58.3483421467591));
#100681=CARTESIAN_POINT('Ctrl Pts',(10.5325668032473,638.447986550465,57.9690756449664));
#100682=CARTESIAN_POINT('Ctrl Pts',(10.2952739748061,638.29783913783,57.6041926021619));
#100683=CARTESIAN_POINT('Ctrl Pts',(10.1290947826648,638.192688991078,57.3486603567179));
#100684=CARTESIAN_POINT('Ctrl Pts',(9.95405618216335,638.083520093995,57.1002579207122));
#100685=CARTESIAN_POINT('Ctrl Pts',(9.77011972364139,637.970987642423,56.8587519976483));
#100686=CARTESIAN_POINT('Ctrl Pts',(9.71724352583497,637.938637948312,56.7893263108543));
#100687=CARTESIAN_POINT('Ctrl Pts',(9.66363239874653,637.906010547357,56.7204710861209));
#100688=CARTESIAN_POINT('Ctrl Pts',(9.60928507234349,637.873120828848,56.6521803974868));
#100689=CARTESIAN_POINT('Ctrl Pts',(9.36573391882352,637.725729422279,56.3461437054853));
#100690=CARTESIAN_POINT('Ctrl Pts',(9.10609991920284,637.572325442271,56.0501477801115));
#100691=CARTESIAN_POINT('Ctrl Pts',(8.83441059956637,637.417055018867,55.7687853847949));
#100692=CARTESIAN_POINT('Ctrl Pts',(8.65468490820217,637.314341801315,55.5826608397085));
#100693=CARTESIAN_POINT('Ctrl Pts',(8.47006004967338,637.210953723151,55.4030725521586));
#100694=CARTESIAN_POINT('Ctrl Pts',(8.28039538036778,637.107420371167,55.2298442867054));
#100695=CARTESIAN_POINT('Ctrl Pts',(7.98903889316609,636.948375917327,54.9637368504007));
#100696=CARTESIAN_POINT('Ctrl Pts',(7.68586832486323,636.78898481371,54.7127055606788));
#100697=CARTESIAN_POINT('Ctrl Pts',(7.37033208728924,636.63116628615,54.4760819004643));
#100698=CARTESIAN_POINT('Ctrl Pts',(7.27003911433903,636.581003777281,54.4008712351672));
#100699=CARTESIAN_POINT('Ctrl Pts',(7.16849659990973,636.531000163409,54.3271164420954));
#100700=CARTESIAN_POINT('Ctrl Pts',(7.06568610310641,636.481217200254,54.25479687612));
#100701=CARTESIAN_POINT('Ctrl Pts',(6.89206181747449,636.39714473992,54.1326650571899));
#100702=CARTESIAN_POINT('Ctrl Pts',(6.7144545011427,636.313583905268,54.0145413134919));
#100703=CARTESIAN_POINT('Ctrl Pts',(6.53323952934815,636.23116157674,53.9007405872068));
#100704=CARTESIAN_POINT('Ctrl Pts',(6.39148708173227,636.166688058402,53.8117218304693));
#100705=CARTESIAN_POINT('Ctrl Pts',(6.2472699640017,636.102791893307,53.7251920165753));
#100706=CARTESIAN_POINT('Ctrl Pts',(6.10103330378201,636.039899820462,53.6414835032635));
#100707=CARTESIAN_POINT('Ctrl Pts',(5.95750527901565,635.978172651807,53.5593254619508));
#100708=CARTESIAN_POINT('Ctrl Pts',(5.81203236067384,635.91741338381,53.4798854136289));
#100709=CARTESIAN_POINT('Ctrl Pts',(5.66506348804016,635.858011845617,53.4034385207361));
#100710=CARTESIAN_POINT('Ctrl Pts',(5.63106986886731,635.844272383434,53.3857565006092));
#100711=CARTESIAN_POINT('Ctrl Pts',(5.5969963195827,635.83060547625,53.3682344347357));
#100712=CARTESIAN_POINT('Ctrl Pts',(5.56284856909546,635.817015784796,53.3508754028232));
#100713=CARTESIAN_POINT('Ctrl Pts',(5.38268096901558,635.745314953551,53.2592870822234));
#100714=CARTESIAN_POINT('Ctrl Pts',(5.19987034695471,635.675533917924,53.171943424336));
#100715=CARTESIAN_POINT('Ctrl Pts',(5.01474362923015,635.608201195631,53.0891303500769));
#100716=CARTESIAN_POINT('Ctrl Pts',(4.85852202040539,635.551381594805,53.019247451209));
#100717=CARTESIAN_POINT('Ctrl Pts',(4.70043407278366,635.496203875722,52.9524335003918));
#100718=CARTESIAN_POINT('Ctrl Pts',(4.54038793194821,635.442907944482,52.888747904314));
#100719=CARTESIAN_POINT('Ctrl Pts',(4.32988395212515,635.372809374309,52.8049841136858));
#100720=CARTESIAN_POINT('Ctrl Pts',(4.11606910508421,635.305988262076,52.7266642081689));
#100721=CARTESIAN_POINT('Ctrl Pts',(3.89880804431974,635.243007435063,52.6539274618112));
#100722=CARTESIAN_POINT('Ctrl Pts',(3.75513870481975,635.201359779536,52.6058284593033));
#100723=CARTESIAN_POINT('Ctrl Pts',(3.6095707650986,635.161317829567,52.5600901866341));
#100724=CARTESIAN_POINT('Ctrl Pts',(3.46260051942188,635.123178534668,52.5169114539384));
#100725=CARTESIAN_POINT('Ctrl Pts',(3.30083889265518,635.08120082443,52.4693871267495));
#100726=CARTESIAN_POINT('Ctrl Pts',(3.13696220031812,635.041422302233,52.4248444110017));
#100727=CARTESIAN_POINT('Ctrl Pts',(2.97184384015041,635.004314248912,52.3836415514606));
#100728=CARTESIAN_POINT('Ctrl Pts',(2.8881795808165,634.985511871071,52.3627643654079));
#100729=CARTESIAN_POINT('Ctrl Pts',(2.80419703337489,634.967394742501,52.3427440958528));
#100730=CARTESIAN_POINT('Ctrl Pts',(2.72001197855739,634.950021400306,52.3236235868221));
#100731=CARTESIAN_POINT('Ctrl Pts',(2.59111236083927,634.923420275291,52.294347294136));
#100732=CARTESIAN_POINT('Ctrl Pts',(2.46182005848197,634.898563490856,52.2671471808513));
#100733=CARTESIAN_POINT('Ctrl Pts',(2.33225003339614,634.875523287659,52.2420568539257));
#100734=CARTESIAN_POINT('Ctrl Pts',(2.0216680222383,634.820295447411,52.181914824996));
#100735=CARTESIAN_POINT('Ctrl Pts',(1.70858199878448,634.775375031004,52.1337147382744));
#100736=CARTESIAN_POINT('Ctrl Pts',(1.39302211019991,634.74153979137,52.0977046786315));
#100737=CARTESIAN_POINT('Ctrl Pts',(1.08056553841527,634.708037298296,52.0620487534243));
#100738=CARTESIAN_POINT('Ctrl Pts',(0.765683584580269,634.685403258863,
52.0383441545871));
#100739=CARTESIAN_POINT('Ctrl Pts',(0.448405337742959,634.674358899197,
52.0267929415571));
#100740=CARTESIAN_POINT('Ctrl Pts',(0.388670115572721,634.672279534207,
52.0246181492933));
#100741=CARTESIAN_POINT('Ctrl Pts',(0.328849950054106,634.67061088699,52.0228740510582));
#100742=CARTESIAN_POINT('Ctrl Pts',(0.26894503217668,634.669357626546,52.0215618471691));
#100743=CARTESIAN_POINT('Ctrl Pts',(0.179555066921117,634.667487514516,
52.0196037798815));
#100744=CARTESIAN_POINT('Ctrl Pts',(0.0898586837318516,634.666558689946,
52.0186356114589));
#100745=CARTESIAN_POINT('Ctrl Pts',(1.07518175474036E-8,634.666563589043,
52.0186534989093));
#100746=CARTESIAN_POINT('Ctrl Pts',(1.7398767070424E-11,606.684227202053,
52.018616610259));
#100747=CARTESIAN_POINT('Ctrl Pts',(0.373817003740921,606.684227202053,
52.0186166102595));
#100748=CARTESIAN_POINT('Ctrl Pts',(0.75120106784948,606.667669882597,52.035969701156));
#100749=CARTESIAN_POINT('Ctrl Pts',(1.49208745862893,606.603562249098,52.1039208858566));
#100750=CARTESIAN_POINT('Ctrl Pts',(1.85829486773971,606.556095266178,52.1544405788514));
#100751=CARTESIAN_POINT('Ctrl Pts',(2.22051577456844,606.494663641934,52.2210317180765));
#100752=CARTESIAN_POINT('Origin',(-48.,620.675373764374,64.2994740882088));
#100753=CARTESIAN_POINT('',(-48.,620.675373764374,44.8494740882088));
#100754=CARTESIAN_POINT('Ctrl Pts',(-3.85030552837329,608.045280920111,
79.0907977188138));
#100755=CARTESIAN_POINT('Ctrl Pts',(-4.23115754611984,607.932105616136,
78.99415899786));
#100756=CARTESIAN_POINT('Ctrl Pts',(-4.60131346252692,607.807253127989,
78.8852799373076));
#100757=CARTESIAN_POINT('Ctrl Pts',(-4.96211414895984,607.673156473991,
78.7647299399134));
#100758=CARTESIAN_POINT('Ctrl Pts',(-5.34276158691742,607.531683495412,
78.6375487859429));
#100759=CARTESIAN_POINT('Ctrl Pts',(-5.71299620598676,607.379921133396,
78.4973774780135));
#100760=CARTESIAN_POINT('Ctrl Pts',(-6.07436314690284,607.220681681377,
78.3448595458295));
#100761=CARTESIAN_POINT('Ctrl Pts',(-6.27213868897694,607.133530186936,
78.2613867283182));
#100762=CARTESIAN_POINT('Ctrl Pts',(-6.46725754698847,607.044138294261,
78.1742152209262));
#100763=CARTESIAN_POINT('Ctrl Pts',(-6.65996976734686,606.952962317827,
78.0834474967339));
#100764=CARTESIAN_POINT('Ctrl Pts',(-6.66518312762042,606.950495773606,
78.080991996784));
#100765=CARTESIAN_POINT('Ctrl Pts',(-6.67039454639831,606.948028009746,
78.0785339506688));
#100766=CARTESIAN_POINT('Ctrl Pts',(-6.67560403513433,606.945559032559,
78.0760733579906));
#100767=CARTESIAN_POINT('Ctrl Pts',(-6.8578343467733,606.859193075165,77.9900006945705));
#100768=CARTESIAN_POINT('Ctrl Pts',(-7.03785733736652,606.771178203692,
77.9006116068874));
#100769=CARTESIAN_POINT('Ctrl Pts',(-7.215789858865,606.6817674534,77.8079341656738));
#100770=CARTESIAN_POINT('Ctrl Pts',(-7.39804086769688,606.590186671518,
77.7130074090872));
#100771=CARTESIAN_POINT('Ctrl Pts',(-7.5780991625022,606.497140675157,77.614630588693));
#100772=CARTESIAN_POINT('Ctrl Pts',(-7.75606262292596,606.402883414968,
77.5127908409613));
#100773=CARTESIAN_POINT('Ctrl Pts',(-7.8179153405013,606.370123500769,77.4773955685869));
#100774=CARTESIAN_POINT('Ctrl Pts',(-7.87951473545424,606.337217167687,
77.4415816227428));
#100775=CARTESIAN_POINT('Ctrl Pts',(-7.94086400011092,606.304174852542,
77.4053473424493));
#100776=CARTESIAN_POINT('Ctrl Pts',(-8.121437580548,606.206919095931,77.2986964516231));
#100777=CARTESIAN_POINT('Ctrl Pts',(-8.30015667393309,606.108308982384,
77.1882091735264));
#100778=CARTESIAN_POINT('Ctrl Pts',(-8.47654659987535,606.008907743947,
77.0741437637344));
#100779=CARTESIAN_POINT('Ctrl Pts',(-8.65758128459169,605.906889038713,
76.9570747452605));
#100780=CARTESIAN_POINT('Ctrl Pts',(-8.83616203701266,605.804037747601,
76.8362367877207));
#100781=CARTESIAN_POINT('Ctrl Pts',(-9.01180166947103,605.700983120861,
76.7119523503828));
#100782=CARTESIAN_POINT('Ctrl Pts',(-9.05844940407669,605.67361307453,76.6789439264445));
#100783=CARTESIAN_POINT('Ctrl Pts',(-9.10488984292617,605.646228758214,
76.6456926236426));
#100784=CARTESIAN_POINT('Ctrl Pts',(-9.15111422548108,605.618842082703,
76.612204957696));
#100785=CARTESIAN_POINT('Ctrl Pts',(-9.15898657611739,605.614177931438,
76.6065017631101));
#100786=CARTESIAN_POINT('Ctrl Pts',(-9.1668522498693,605.609513942502,76.6007919954538));
#100787=CARTESIAN_POINT('Ctrl Pts',(-9.17471122726756,605.60485016159,76.5950756732529));
#100788=CARTESIAN_POINT('Ctrl Pts',(-9.60207382531122,605.351238854893,
76.2842283220931));
#100789=CARTESIAN_POINT('Ctrl Pts',(-10.0116117983045,605.097205235008,
75.953330317504));
#100790=CARTESIAN_POINT('Ctrl Pts',(-10.4040324386218,604.845763559111,
75.6011406067169));
#100791=CARTESIAN_POINT('Ctrl Pts',(-10.7191297461544,604.64386644429,75.3183470474384));
#100792=CARTESIAN_POINT('Ctrl Pts',(-11.0231911890468,604.44364022255,75.0218264745212));
#100793=CARTESIAN_POINT('Ctrl Pts',(-11.3165906288581,604.246631862434,
74.7109552956669));
#100794=CARTESIAN_POINT('Ctrl Pts',(-11.3211660968142,604.243559581725,
74.7061073616756));
#100795=CARTESIAN_POINT('Ctrl Pts',(-11.3257389714887,604.240488082105,
74.701255936195));
#100796=CARTESIAN_POINT('Ctrl Pts',(-11.330309255645,604.23741736854,74.6964010155038));
#100797=CARTESIAN_POINT('Ctrl Pts',(-11.5510374470401,604.089113011908,
74.4619259091729));
#100798=CARTESIAN_POINT('Ctrl Pts',(-11.7657533239914,603.942514229819,
74.2189269147374));
#100799=CARTESIAN_POINT('Ctrl Pts',(-11.9729190514427,603.799244900531,
73.9689066228666));
#100800=CARTESIAN_POINT('Ctrl Pts',(-12.0734225150265,603.729739852587,
73.8476128856814));
#100801=CARTESIAN_POINT('Ctrl Pts',(-12.1721485958898,603.661018499151,
73.7246659781166));
#100802=CARTESIAN_POINT('Ctrl Pts',(-12.2689186597508,603.593267506438,
73.6002344485137));
#100803=CARTESIAN_POINT('Ctrl Pts',(-12.2725876177275,603.590698782855,
73.5955167286437));
#100804=CARTESIAN_POINT('Ctrl Pts',(-12.2762537641056,603.588131453901,
73.5907968737177));
#100805=CARTESIAN_POINT('Ctrl Pts',(-12.2799170881477,603.585565530419,
73.5860748940442));
#100806=CARTESIAN_POINT('Ctrl Pts',(-12.5761628621236,603.378064370561,
73.2042177318029));
#100807=CARTESIAN_POINT('Ctrl Pts',(-12.8553373541657,603.178825518264,
72.8071138322945));
#100808=CARTESIAN_POINT('Ctrl Pts',(-13.1169859722107,602.989662224037,
72.3937997341821));
#100809=CARTESIAN_POINT('Ctrl Pts',(-13.1196323729917,602.987748963828,
72.3896193385041));
#100810=CARTESIAN_POINT('Ctrl Pts',(-13.1222769834676,602.985836732372,
72.3854372806603));
#100811=CARTESIAN_POINT('Ctrl Pts',(-13.124919803262,602.983925531487,72.3812535595345));
#100812=CARTESIAN_POINT('Ctrl Pts',(-13.3868026742264,602.794540399873,
71.9666793603881));
#100813=CARTESIAN_POINT('Ctrl Pts',(-13.631110707103,602.615257919091,71.5357863466911));
#100814=CARTESIAN_POINT('Ctrl Pts',(-13.856691485181,602.448092654014,71.0868685526235));
#100815=CARTESIAN_POINT('Ctrl Pts',(-13.8582610272093,602.446929554429,
71.0837450801759));
#100816=CARTESIAN_POINT('Ctrl Pts',(-13.859829662386,602.445767041551,71.0806207352235));
#100817=CARTESIAN_POINT('Ctrl Pts',(-13.8613973903024,602.444605116074,
71.0774955172258));
#100818=CARTESIAN_POINT('Ctrl Pts',(-14.0874235511567,602.277085260077,
70.6269192287555));
#100819=CARTESIAN_POINT('Ctrl Pts',(-14.2932373615726,602.12276713293,70.1602556258246));
#100820=CARTESIAN_POINT('Ctrl Pts',(-14.4749373298438,601.985591928934,
69.6841332957598));
#100821=CARTESIAN_POINT('Ctrl Pts',(-14.475477179548,601.985184366985,69.6827186862722));
#100822=CARTESIAN_POINT('Ctrl Pts',(-14.476016816648,601.984776956179,69.6813039927107));
#100823=CARTESIAN_POINT('Ctrl Pts',(-14.476556241042,601.984369696621,69.6798892152476));
#100824=CARTESIAN_POINT('Ctrl Pts',(-14.6585293164953,601.846982001182,
69.2026186118272));
#100825=CARTESIAN_POINT('Ctrl Pts',(-14.8173572004353,601.726014684511,
68.7137722568826));
#100826=CARTESIAN_POINT('Ctrl Pts',(-14.9519074395826,601.623084951773,
68.2126302314325));
#100827=CARTESIAN_POINT('Ctrl Pts',(-14.9521319248731,601.622913222528,
68.2117941198516));
#100828=CARTESIAN_POINT('Ctrl Pts',(-14.9523563424351,601.622741543562,
68.2109579739804));
#100829=CARTESIAN_POINT('Ctrl Pts',(-14.95258069226,601.622569914884,68.210121793814));
#100830=CARTESIAN_POINT('Ctrl Pts',(-15.0195558479621,601.571333603616,
67.9604969194963));
#100831=CARTESIAN_POINT('Ctrl Pts',(-15.0804980243008,601.524576095695,
67.7077995412209));
#100832=CARTESIAN_POINT('Ctrl Pts',(-15.1351710050067,601.48254956767,67.4519333432102));
#100833=CARTESIAN_POINT('Ctrl Pts',(-15.135636996097,601.482191365367,67.4497525334749));
#100834=CARTESIAN_POINT('Ctrl Pts',(-15.1361025388452,601.481833501261,
67.4475714348023));
#100835=CARTESIAN_POINT('Ctrl Pts',(-15.1365676327062,601.48147597581,67.4453900497329));
#100836=CARTESIAN_POINT('Ctrl Pts',(-15.1908350502443,601.439759701831,
67.1908647929737));
#100837=CARTESIAN_POINT('Ctrl Pts',(-15.2390028207857,601.402644801267,
66.9323762776556));
#100838=CARTESIAN_POINT('Ctrl Pts',(-15.2801892173651,601.370866225702,
66.6740242960524));
#100839=CARTESIAN_POINT('Ctrl Pts',(-15.2807701109302,601.370418020188,
66.6703804957663));
#100840=CARTESIAN_POINT('Ctrl Pts',(-15.2813496618532,601.369970844881,
66.666736612685));
#100841=CARTESIAN_POINT('Ctrl Pts',(-15.2819278700575,601.369524699882,
66.6630926470816));
#100842=CARTESIAN_POINT('Ctrl Pts',(-15.3731745585429,601.299118826362,
66.0880406298869));
#100843=CARTESIAN_POINT('Ctrl Pts',(-15.4310118252878,601.254354048509,
65.5107688555495));
#100844=CARTESIAN_POINT('Ctrl Pts',(-15.4552801915147,601.235537263915,
64.9313506760282));
#100845=CARTESIAN_POINT('Ctrl Pts',(-15.4748377843986,601.220373036994,
64.4644043328481));
#100846=CARTESIAN_POINT('Ctrl Pts',(-15.4725946351504,601.222060296525,
63.9960640263858));
#100847=CARTESIAN_POINT('Ctrl Pts',(-15.4484868316277,601.240744657969,
63.526368979289));
#100848=CARTESIAN_POINT('Ctrl Pts',(-15.4479899849941,601.24112973088,63.5166888604538));
#100849=CARTESIAN_POINT('Ctrl Pts',(-15.4474835199924,601.241522257243,
63.5070072900479));
#100850=CARTESIAN_POINT('Ctrl Pts',(-15.4469674516523,601.241922223809,
63.4973243783675));
#100851=CARTESIAN_POINT('Ctrl Pts',(-15.4286622195785,601.25610926116,63.1538660964509));
#100852=CARTESIAN_POINT('Ctrl Pts',(-15.3982529686908,601.279665380914,
62.8085899300613));
#100853=CARTESIAN_POINT('Ctrl Pts',(-15.3564213514686,601.311998214373,
62.4665526792109));
#100854=CARTESIAN_POINT('Ctrl Pts',(-15.3350964847613,601.328480803609,
62.2921893801648));
#100855=CARTESIAN_POINT('Ctrl Pts',(-15.3108039221149,601.347243706909,
62.1186678639537));
#100856=CARTESIAN_POINT('Ctrl Pts',(-15.283637958771,601.368205423024,61.9466564924111));
#100857=CARTESIAN_POINT('Ctrl Pts',(-15.2816660309461,601.369726995837,
61.9341705000882));
#100858=CARTESIAN_POINT('Ctrl Pts',(-15.2796790199361,601.371260110549,
61.9216904451658));
#100859=CARTESIAN_POINT('Ctrl Pts',(-15.2776769461705,601.372804744798,
61.9092163265372));
#100860=CARTESIAN_POINT('Ctrl Pts',(-15.1964258864429,601.43549133098,61.4029735620699));
#100861=CARTESIAN_POINT('Ctrl Pts',(-15.0903354122302,601.517167712133,
60.906367091332));
#100862=CARTESIAN_POINT('Ctrl Pts',(-14.9606030100877,601.616433700872,
60.4188422252059));
#100863=CARTESIAN_POINT('Ctrl Pts',(-14.9567124177469,601.619410624826,
60.4042216641215));
#100864=CARTESIAN_POINT('Ctrl Pts',(-14.9528005558405,601.622403377454,
60.3896092743672));
#100865=CARTESIAN_POINT('Ctrl Pts',(-14.9488674344808,601.625411931282,
60.3750050482591));
#100866=CARTESIAN_POINT('Ctrl Pts',(-14.8183427926634,601.725253857031,
59.8903489170524));
#100867=CARTESIAN_POINT('Ctrl Pts',(-14.6644248370208,601.842487872357,
59.4147167113827));
#100868=CARTESIAN_POINT('Ctrl Pts',(-14.4874575536325,601.976141950479,
58.9477239471356));
#100869=CARTESIAN_POINT('Ctrl Pts',(-14.4812763675599,601.980810275101,
58.9314126317608));
#100870=CARTESIAN_POINT('Ctrl Pts',(-14.4750668043185,601.98549878938,58.9151121429094));
#100871=CARTESIAN_POINT('Ctrl Pts',(-14.4688293500762,601.990207092219,
58.898823461902));
#100872=CARTESIAN_POINT('Ctrl Pts',(-14.3830461531583,602.054959995219,
58.6748065671682));
#100873=CARTESIAN_POINT('Ctrl Pts',(-14.292004696505,602.123442202462,58.4530694500958));
#100874=CARTESIAN_POINT('Ctrl Pts',(-14.1969736437625,602.194605881907,
58.2361648853124));
#100875=CARTESIAN_POINT('Ctrl Pts',(-14.094982172067,602.270981847324,58.0033734435543));
#100876=CARTESIAN_POINT('Ctrl Pts',(-13.9880772628478,602.350687445523,
57.7752684237754));
#100877=CARTESIAN_POINT('Ctrl Pts',(-13.8764789934297,602.433436002756,
57.5515702123706));
#100878=CARTESIAN_POINT('Ctrl Pts',(-13.8680348690463,602.439697202983,
57.5346440043631));
#100879=CARTESIAN_POINT('Ctrl Pts',(-13.8595642190567,602.445975710707,
57.5177427581886));
#100880=CARTESIAN_POINT('Ctrl Pts',(-13.851067080703,602.452271426782,57.5008664006862));
#100881=CARTESIAN_POINT('Ctrl Pts',(-13.5414068385151,602.681705488394,
56.8858432324252));
#100882=CARTESIAN_POINT('Ctrl Pts',(-13.1966130805123,602.933991273143,
56.3038699396781));
#100883=CARTESIAN_POINT('Ctrl Pts',(-12.818575692922,603.204311674987,55.7515264358009));
#100884=CARTESIAN_POINT('Ctrl Pts',(-12.6579969944005,603.319135498601,
55.516907840125));
#100885=CARTESIAN_POINT('Ctrl Pts',(-12.4914199381588,603.437213717574,
55.2876357592081));
#100886=CARTESIAN_POINT('Ctrl Pts',(-12.3189883302193,603.558178954703,
55.0634499517658));
#100887=CARTESIAN_POINT('Ctrl Pts',(-12.3063145884526,603.567069912668,
55.046972270758));
#100888=CARTESIAN_POINT('Ctrl Pts',(-12.293608875228,603.575976591379,55.0305223394531));
#100889=CARTESIAN_POINT('Ctrl Pts',(-12.2808711596615,603.584898854644,
55.0141001141053));
#100890=CARTESIAN_POINT('Ctrl Pts',(-12.1059805186862,603.70740279448,54.788620631358));
#100891=CARTESIAN_POINT('Ctrl Pts',(-11.9251378242665,603.832790898451,
54.5684575845009));
#100892=CARTESIAN_POINT('Ctrl Pts',(-11.7381263933771,603.960807456315,
54.3533266754511));
#100893=CARTESIAN_POINT('Ctrl Pts',(-11.621570829978,604.040594247718,54.2192455436742));
#100894=CARTESIAN_POINT('Ctrl Pts',(-11.5026183161173,604.121402448223,
54.0871197659894));
#100895=CARTESIAN_POINT('Ctrl Pts',(-11.3812089157723,604.203173369559,
53.9568866869203));
#100896=CARTESIAN_POINT('Ctrl Pts',(-11.3665916244721,604.213018318744,
53.9412070538089));
#100897=CARTESIAN_POINT('Ctrl Pts',(-11.3519440806364,604.222873520687,
53.9255610169989));
#100898=CARTESIAN_POINT('Ctrl Pts',(-11.3372665071724,604.23273864033,53.909948683445));
#100899=CARTESIAN_POINT('Ctrl Pts',(-11.1445926511092,604.362238972701,
53.7050041457561));
#100900=CARTESIAN_POINT('Ctrl Pts',(-10.9471021948111,604.493214313288,
53.5062326251606));
#100901=CARTESIAN_POINT('Ctrl Pts',(-10.745312746339,604.624903460212,53.313822665779));
#100902=CARTESIAN_POINT('Ctrl Pts',(-10.6147258174735,604.71012536548,53.1893056215578));
#100903=CARTESIAN_POINT('Ctrl Pts',(-10.4823376624323,604.795646602209,
53.0674534899227));
#100904=CARTESIAN_POINT('Ctrl Pts',(-10.3482814114362,604.881262749726,
52.9483262480232));
#100905=CARTESIAN_POINT('Ctrl Pts',(-10.3323385786133,604.891444773441,
52.9341588691196));
#100906=CARTESIAN_POINT('Ctrl Pts',(-10.316370473426,604.901629819377,52.9200274595625));
#100907=CARTESIAN_POINT('Ctrl Pts',(-10.3003769198535,604.911817706811,
52.9059318994444));
#100908=CARTESIAN_POINT('Ctrl Pts',(-9.82420777102504,605.215137270266,
52.4862708883196));
#100909=CARTESIAN_POINT('Ctrl Pts',(-9.32605084326132,605.520676590294,
52.0987968357783));
#100910=CARTESIAN_POINT('Ctrl Pts',(-8.80356011337631,605.822413129915,
51.7419140852932));
#100911=CARTESIAN_POINT('Ctrl Pts',(-8.55658179181229,605.965042232878,
51.5732176899919));
#100912=CARTESIAN_POINT('Ctrl Pts',(-8.30416681543672,606.10682215787,51.4113565816857));
#100913=CARTESIAN_POINT('Ctrl Pts',(-8.04607025545264,606.247119801894,
51.256162100614));
#100914=CARTESIAN_POINT('Ctrl Pts',(-8.02850322970694,606.25666898893,51.2455989786384));
#100915=CARTESIAN_POINT('Ctrl Pts',(-8.01090956281672,606.266211131474,
51.2350670302149));
#100916=CARTESIAN_POINT('Ctrl Pts',(-7.9932890588355,606.275745937602,51.2245662881426));
#100917=CARTESIAN_POINT('Ctrl Pts',(-7.59780332812586,606.48975115405,50.9888809946957));
#100918=CARTESIAN_POINT('Ctrl Pts',(-7.18882425917877,606.700057952479,
50.7689174218948));
#100919=CARTESIAN_POINT('Ctrl Pts',(-6.76412222102934,606.903391967464,
50.5650277071314));
#100920=CARTESIAN_POINT('Ctrl Pts',(-6.32001855033077,607.116014875577,
50.3518237132475));
#100921=CARTESIAN_POINT('Ctrl Pts',(-5.8641859945191,607.318324825404,50.1588849102787));
#100922=CARTESIAN_POINT('Ctrl Pts',(-5.39617905494641,607.50523847829,49.9868909337918));
#100923=CARTESIAN_POINT('Ctrl Pts',(-5.37904744986577,607.512080536847,
49.9805950167182));
#100924=CARTESIAN_POINT('Ctrl Pts',(-5.36189899496725,607.518902273776,
49.9743268675902));
#100925=CARTESIAN_POINT('Ctrl Pts',(-5.34473356176528,607.525703405737,
49.9680865467441));
#100926=CARTESIAN_POINT('Ctrl Pts',(-5.05505639185856,607.640476661693,
49.8627773208862));
#100927=CARTESIAN_POINT('Ctrl Pts',(-4.7604858066973,607.749407504922,49.7653700783089));
#100928=CARTESIAN_POINT('Ctrl Pts',(-4.46054827631106,607.851090892826,
49.6761957671012));
#100929=CARTESIAN_POINT('Ctrl Pts',(-4.29218546500682,607.90816844837,49.6261398847589));
#100930=CARTESIAN_POINT('Ctrl Pts',(-4.12213195856964,607.96296293255,49.5786775358458));
#100931=CARTESIAN_POINT('Ctrl Pts',(-3.95030718844,608.015230706238,49.5338627639009));
#100932=CARTESIAN_POINT('Ctrl Pts',(-3.93446701216018,608.020049166047,
49.5297313811729));
#100933=CARTESIAN_POINT('Ctrl Pts',(-3.918608077318,608.024846507359,49.5256222106105));
#100934=CARTESIAN_POINT('Ctrl Pts',(-3.90273095451652,608.029622392916,
49.5215354186));
#100935=CARTESIAN_POINT('Ctrl Pts',(-3.55379715979371,608.13458271168,49.4317194070769));
#100936=CARTESIAN_POINT('Ctrl Pts',(-3.19571883730709,608.229248742951,
49.3526530596434));
#100937=CARTESIAN_POINT('Ctrl Pts',(-2.83439734133167,608.310054485557,
49.2860999619015));
#100938=CARTESIAN_POINT('Ctrl Pts',(-2.69666016753091,608.340857952102,
49.260729659573));
#100939=CARTESIAN_POINT('Ctrl Pts',(-2.55845161164899,608.369647675702,
49.2371774467656));
#100940=CARTESIAN_POINT('Ctrl Pts',(-2.4200977988402,608.396227713108,49.2155398450576));
#100941=CARTESIAN_POINT('Ctrl Pts',(-2.40660419108442,608.398820056548,
49.2134295359574));
#100942=CARTESIAN_POINT('Ctrl Pts',(-2.39310738388888,608.401392124616,
49.2113367450485));
#100943=CARTESIAN_POINT('Ctrl Pts',(-2.37960737536317,608.40394385778,49.209261482295));
#100944=CARTESIAN_POINT('Ctrl Pts',(-1.98661162622564,608.478226795045,
49.1488489693005));
#100945=CARTESIAN_POINT('Ctrl Pts',(-1.59091824851033,608.535255871218,
49.1033073919222));
#100946=CARTESIAN_POINT('Ctrl Pts',(-1.19224235498086,608.573554311811,
49.072890147475));
#100947=CARTESIAN_POINT('Ctrl Pts',(-1.07867395166442,608.584464158176,
49.0642253700424));
#100948=CARTESIAN_POINT('Ctrl Pts',(-0.964863484237993,608.593853827031,
49.0567881087316));
#100949=CARTESIAN_POINT('Ctrl Pts',(-0.850804267018435,608.601688592408,
49.0505847395293));
#100950=CARTESIAN_POINT('Ctrl Pts',(-0.467771498280798,608.627999240051,
49.0297526337251));
#100951=CARTESIAN_POINT('Ctrl Pts',(-0.0819322950985286,608.636758310879,
49.0228304603039));
#100952=CARTESIAN_POINT('Ctrl Pts',(0.306952880974604,608.627117381494,
49.0304624743328));
#100953=CARTESIAN_POINT('Ctrl Pts',(0.454443680653595,608.623460907881,
49.0333570353024));
#100954=CARTESIAN_POINT('Ctrl Pts',(0.602372687010726,608.617157325412,
49.038345428801));
#100955=CARTESIAN_POINT('Ctrl Pts',(0.750753219933458,608.608158800935,
49.0454640244197));
#100956=CARTESIAN_POINT('Ctrl Pts',(0.757600042190903,608.607743575996,
49.0457925025426));
#100957=CARTESIAN_POINT('Ctrl Pts',(0.764445410940781,608.607322738532,
49.0461253700537));
#100958=CARTESIAN_POINT('Ctrl Pts',(0.77128932685212,608.60689629941,49.0464626238936));
#100959=CARTESIAN_POINT('Ctrl Pts',(1.0999295210194,608.586418982362,49.0626573242459));
#100960=CARTESIAN_POINT('Ctrl Pts',(1.42500065461206,608.553042141358,49.0889528591604));
#100961=CARTESIAN_POINT('Ctrl Pts',(1.74665485822711,608.507994127727,49.1249902270901));
#100962=CARTESIAN_POINT('Ctrl Pts',(1.94934880633034,608.479606624518,49.1476995724145));
#100963=CARTESIAN_POINT('Ctrl Pts',(2.15068565983306,608.446583546877,49.1742781049698));
#100964=CARTESIAN_POINT('Ctrl Pts',(2.35070124101387,608.409224348695,49.2046424827418));
#100965=CARTESIAN_POINT('Ctrl Pts',(2.5214420972517,608.377333125781,49.2305626627063));
#100966=CARTESIAN_POINT('Ctrl Pts',(2.69150512765591,608.342225093235,49.2592881187915));
#100967=CARTESIAN_POINT('Ctrl Pts',(2.86062884454046,608.304125672787,49.2907367311987));
#100968=CARTESIAN_POINT('Ctrl Pts',(3.03567001919357,608.264693194413,49.3232856968811));
#100969=CARTESIAN_POINT('Ctrl Pts',(3.20970492776411,608.222056535811,49.3587517991215));
#100970=CARTESIAN_POINT('Ctrl Pts',(3.38245717567461,608.176507008384,49.3970067274567));
#100971=CARTESIAN_POINT('Ctrl Pts',(3.54860965817915,608.132697638895,49.4338001781227));
#100972=CARTESIAN_POINT('Ctrl Pts',(3.71357570183652,608.0861943321,49.4731731008924));
#100973=CARTESIAN_POINT('Ctrl Pts',(3.87712128125395,608.037287038732,49.5149800517143));
#100974=CARTESIAN_POINT('',(-3.85030552837329,633.305466608637,79.0907977188138));
#100975=CARTESIAN_POINT('',(3.87712128125394,633.313460490016,49.5149800517143));
#100976=CARTESIAN_POINT('Ctrl Pts',(-3.85030552837329,633.305466608637,
79.0907977188139));
#100977=CARTESIAN_POINT('Ctrl Pts',(-4.23115754609872,633.418641912605,
78.9941589978653));
#100978=CARTESIAN_POINT('Ctrl Pts',(-4.60131346248585,633.543494400745,
78.8852799373196));
#100979=CARTESIAN_POINT('Ctrl Pts',(-4.96211414889978,633.677591054735,
78.7647299399334));
#100980=CARTESIAN_POINT('Ctrl Pts',(-5.34276158684725,633.819064033309,
78.637548785968));
#100981=CARTESIAN_POINT('Ctrl Pts',(-5.71299620590704,633.970826395318,
78.4973774780445));
#100982=CARTESIAN_POINT('Ctrl Pts',(-6.07436314681395,634.130065847331,
78.344859545867));
#100983=CARTESIAN_POINT('Ctrl Pts',(-6.27213868891848,634.217217341785,
78.2613867283443));
#100984=CARTESIAN_POINT('Ctrl Pts',(-6.46725754695957,634.306609234473,
78.1742152209399));
#100985=CARTESIAN_POINT('Ctrl Pts',(-6.65996976734683,634.39778521092,78.083447496734));
#100986=CARTESIAN_POINT('Ctrl Pts',(-6.66518312762043,634.400251755141,
78.0809919967841));
#100987=CARTESIAN_POINT('Ctrl Pts',(-6.67039454639835,634.402719519002,
78.0785339506688));
#100988=CARTESIAN_POINT('Ctrl Pts',(-6.67560403513441,634.405188496189,
78.0760733579906));
#100989=CARTESIAN_POINT('Ctrl Pts',(-6.85783434677776,634.491554453585,
77.9900006945685));
#100990=CARTESIAN_POINT('Ctrl Pts',(-7.03785733737531,634.57956932506,77.9006116068831));
#100991=CARTESIAN_POINT('Ctrl Pts',(-7.21578985887797,634.668980075354,
77.8079341656671));
#100992=CARTESIAN_POINT('Ctrl Pts',(-7.39804086771728,634.76056085724,77.7130074090763));
#100993=CARTESIAN_POINT('Ctrl Pts',(-7.57809916252988,634.853606853605,
77.6146305886777));
#100994=CARTESIAN_POINT('Ctrl Pts',(-7.75606262296074,634.947864113798,
77.5127908409413));
#100995=CARTESIAN_POINT('Ctrl Pts',(-7.81791534052439,634.980624027991,
77.4773955685734));
#100996=CARTESIAN_POINT('Ctrl Pts',(-7.87951473546575,635.013530361067,
77.441581622736));
#100997=CARTESIAN_POINT('Ctrl Pts',(-7.94086400011093,635.046572676206,
77.4053473424492));
#100998=CARTESIAN_POINT('Ctrl Pts',(-8.12143758056441,635.143828432826,
77.2986964516133));
#100999=CARTESIAN_POINT('Ctrl Pts',(-8.30015667396553,635.242438546382,
77.1882091735063));
#101000=CARTESIAN_POINT('Ctrl Pts',(-8.47654659992338,635.341839784828,
77.0741437637033));
#101001=CARTESIAN_POINT('Ctrl Pts',(-8.65758128464239,635.443858490064,
76.9570747452268));
#101002=CARTESIAN_POINT('Ctrl Pts',(-8.83616203706591,635.546709781178,
76.8362367876842));
#101003=CARTESIAN_POINT('Ctrl Pts',(-9.01180166952668,635.649764407919,
76.7119523503434));
#101004=CARTESIAN_POINT('Ctrl Pts',(-9.05844940411363,635.677134454239,
76.6789439264181));
#101005=CARTESIAN_POINT('Ctrl Pts',(-9.10488984294456,635.704518770545,
76.6456926236292));
#101006=CARTESIAN_POINT('Ctrl Pts',(-9.15111422548109,635.731905446044,
76.6122049576959));
#101007=CARTESIAN_POINT('Ctrl Pts',(-9.1589865761174,635.73656959731,76.60650176311));
#101008=CARTESIAN_POINT('Ctrl Pts',(-9.1668522498693,635.741233586245,76.6007919954539));
#101009=CARTESIAN_POINT('Ctrl Pts',(-9.17471122726756,635.745897367157,
76.5950756732529));
#101010=CARTESIAN_POINT('Ctrl Pts',(-9.60207382528573,635.99950867384,76.2842283221116));
#101011=CARTESIAN_POINT('Ctrl Pts',(-10.0116117982556,636.253542293709,
75.9533303175435));
#101012=CARTESIAN_POINT('Ctrl Pts',(-10.4040324385516,636.504983969591,
75.6011406067799));
#101013=CARTESIAN_POINT('Ctrl Pts',(-10.7191297461092,636.706881084428,
75.3183470474824));
#101014=CARTESIAN_POINT('Ctrl Pts',(-11.023191189025,636.907107306183,75.0218264745442));
#101015=CARTESIAN_POINT('Ctrl Pts',(-11.316590628858,637.104115666314,74.7109552956668));
#101016=CARTESIAN_POINT('Ctrl Pts',(-11.321166096814,637.107187947022,74.7061073616755));
#101017=CARTESIAN_POINT('Ctrl Pts',(-11.3257389714886,637.110259446643,
74.7012559361948));
#101018=CARTESIAN_POINT('Ctrl Pts',(-11.3303092556449,637.113330160208,
74.6964010155037));
#101019=CARTESIAN_POINT('Ctrl Pts',(-11.5510374470378,637.261634516839,
74.4619259091749));
#101020=CARTESIAN_POINT('Ctrl Pts',(-11.7657533239874,637.408233298925,
74.2189269147418));
#101021=CARTESIAN_POINT('Ctrl Pts',(-11.972919051437,637.551502628213,73.9689066228734));
#101022=CARTESIAN_POINT('Ctrl Pts',(-12.0734225150228,637.621007676158,
73.847612885686));
#101023=CARTESIAN_POINT('Ctrl Pts',(-12.1721485958881,637.689729029595,
73.724665978119));
#101024=CARTESIAN_POINT('Ctrl Pts',(-12.2689186597508,637.757480022309,
73.6002344485137));
#101025=CARTESIAN_POINT('Ctrl Pts',(-12.2725876177276,637.760048745892,
73.5955167286437));
#101026=CARTESIAN_POINT('Ctrl Pts',(-12.2762537641056,637.762616074847,
73.5907968737177));
#101027=CARTESIAN_POINT('Ctrl Pts',(-12.2799170881477,637.765181998328,
73.5860748940442));
#101028=CARTESIAN_POINT('Ctrl Pts',(-12.5761628621236,637.972683158187,
73.2042177318029));
#101029=CARTESIAN_POINT('Ctrl Pts',(-12.8553373541657,638.171922010484,
72.8071138322945));
#101030=CARTESIAN_POINT('Ctrl Pts',(-13.1169859722108,638.361085304711,
72.393799734182));
#101031=CARTESIAN_POINT('Ctrl Pts',(-13.1196323729917,638.36299856492,72.3896193385041));
#101032=CARTESIAN_POINT('Ctrl Pts',(-13.1222769834676,638.364910796376,
72.3854372806603));
#101033=CARTESIAN_POINT('Ctrl Pts',(-13.124919803262,638.36682199726,72.3812535595345));
#101034=CARTESIAN_POINT('Ctrl Pts',(-13.3868026742264,638.556207128875,
71.966679360388));
#101035=CARTESIAN_POINT('Ctrl Pts',(-13.631110707103,638.735489609657,71.5357863466911));
#101036=CARTESIAN_POINT('Ctrl Pts',(-13.8566914851811,638.902654874734,
71.0868685526236));
#101037=CARTESIAN_POINT('Ctrl Pts',(-13.8582610272094,638.903817974319,
71.0837450801759));
#101038=CARTESIAN_POINT('Ctrl Pts',(-13.8598296623861,638.904980487196,
71.0806207352236));
#101039=CARTESIAN_POINT('Ctrl Pts',(-13.8613973903024,638.906142412673,
71.0774955172259));
#101040=CARTESIAN_POINT('Ctrl Pts',(-14.0874235511568,639.073662268671,
70.6269192287556));
#101041=CARTESIAN_POINT('Ctrl Pts',(-14.2932373615726,639.227980395818,
70.1602556258246));
#101042=CARTESIAN_POINT('Ctrl Pts',(-14.4749373298438,639.365155599813,
69.6841332957598));
#101043=CARTESIAN_POINT('Ctrl Pts',(-14.475477179548,639.365563161763,69.6827186862722));
#101044=CARTESIAN_POINT('Ctrl Pts',(-14.476016816648,639.365970572568,69.6813039927107));
#101045=CARTESIAN_POINT('Ctrl Pts',(-14.476556241042,639.366377832127,69.6798892152477));
#101046=CARTESIAN_POINT('Ctrl Pts',(-14.6585293164953,639.503765527566,
69.2026186118272));
#101047=CARTESIAN_POINT('Ctrl Pts',(-14.8173572004353,639.624732844237,
68.7137722568825));
#101048=CARTESIAN_POINT('Ctrl Pts',(-14.9519074395826,639.727662576974,
68.2126302314325));
#101049=CARTESIAN_POINT('Ctrl Pts',(-14.9521319248731,639.727834306219,
68.2117941198516));
#101050=CARTESIAN_POINT('Ctrl Pts',(-14.9523563424351,639.728005985186,
68.2109579739804));
#101051=CARTESIAN_POINT('Ctrl Pts',(-14.95258069226,639.728177613864,68.210121793814));
#101052=CARTESIAN_POINT('Ctrl Pts',(-15.0195558479621,639.779413925132,
67.9604969194963));
#101053=CARTESIAN_POINT('Ctrl Pts',(-15.0804980243008,639.826171433052,
67.7077995412209));
#101054=CARTESIAN_POINT('Ctrl Pts',(-15.1351710050066,639.868197961077,
67.4519333432102));
#101055=CARTESIAN_POINT('Ctrl Pts',(-15.135636996097,639.868556163381,67.4497525334749));
#101056=CARTESIAN_POINT('Ctrl Pts',(-15.1361025388452,639.868914027486,
67.4475714348023));
#101057=CARTESIAN_POINT('Ctrl Pts',(-15.1365676327062,639.869271552937,
67.4453900497329));
#101058=CARTESIAN_POINT('Ctrl Pts',(-15.1908350502443,639.910987826917,
67.1908647929736));
#101059=CARTESIAN_POINT('Ctrl Pts',(-15.2390028207857,639.94810272748,66.9323762776555));
#101060=CARTESIAN_POINT('Ctrl Pts',(-15.2801892173651,639.979881303045,
66.6740242960524));
#101061=CARTESIAN_POINT('Ctrl Pts',(-15.2807701109302,639.980329508559,
66.6703804957663));
#101062=CARTESIAN_POINT('Ctrl Pts',(-15.2813496618532,639.980776683867,
66.6667366126849));
#101063=CARTESIAN_POINT('Ctrl Pts',(-15.2819278700575,639.981222828865,
66.6630926470815));
#101064=CARTESIAN_POINT('Ctrl Pts',(-15.3731745585433,640.051628702386,
66.0880406298841));
#101065=CARTESIAN_POINT('Ctrl Pts',(-15.4310118252884,640.096393480239,
65.5107688555439));
#101066=CARTESIAN_POINT('Ctrl Pts',(-15.4552801915151,640.115210264833,
64.9313506760199));
#101067=CARTESIAN_POINT('Ctrl Pts',(-15.4748377843986,640.130374491754,
64.4644043328425));
#101068=CARTESIAN_POINT('Ctrl Pts',(-15.4725946351503,640.128687232222,
63.9960640263831));
#101069=CARTESIAN_POINT('Ctrl Pts',(-15.4484868316277,640.110002870779,
63.5263689792891));
#101070=CARTESIAN_POINT('Ctrl Pts',(-15.4479899849941,640.109617797867,
63.5166888604539));
#101071=CARTESIAN_POINT('Ctrl Pts',(-15.4474835199924,640.109225271504,
63.5070072900479));
#101072=CARTESIAN_POINT('Ctrl Pts',(-15.4469674516523,640.108825304938,
63.4973243783675));
#101073=CARTESIAN_POINT('Ctrl Pts',(-15.4286622195784,640.094638267587,
63.1538660964489));
#101074=CARTESIAN_POINT('Ctrl Pts',(-15.3982529686904,640.071082147833,
62.8085899300572));
#101075=CARTESIAN_POINT('Ctrl Pts',(-15.3564213514678,640.038749314374,
62.4665526792047));
#101076=CARTESIAN_POINT('Ctrl Pts',(-15.3350964847608,640.022266725138,
62.2921893801607));
#101077=CARTESIAN_POINT('Ctrl Pts',(-15.3108039221145,640.003503821838,
62.1186678639517));
#101078=CARTESIAN_POINT('Ctrl Pts',(-15.283637958771,639.982542105723,61.9466564924111));
#101079=CARTESIAN_POINT('Ctrl Pts',(-15.2816660309461,639.98102053291,61.9341705000882));
#101080=CARTESIAN_POINT('Ctrl Pts',(-15.2796790199361,639.979487418199,
61.9216904451658));
#101081=CARTESIAN_POINT('Ctrl Pts',(-15.2776769461705,639.977942783949,
61.9092163265373));
#101082=CARTESIAN_POINT('Ctrl Pts',(-15.1964258864429,639.915256197767,
61.40297356207));
#101083=CARTESIAN_POINT('Ctrl Pts',(-15.0903354122302,639.833579816615,
60.9063670913321));
#101084=CARTESIAN_POINT('Ctrl Pts',(-14.9606030100877,639.734313827876,
60.4188422252059));
#101085=CARTESIAN_POINT('Ctrl Pts',(-14.9567124177469,639.731336903922,
60.4042216641216));
#101086=CARTESIAN_POINT('Ctrl Pts',(-14.9528005558405,639.728344151294,
60.3896092743672));
#101087=CARTESIAN_POINT('Ctrl Pts',(-14.9488674344808,639.725335597466,
60.3750050482591));
#101088=CARTESIAN_POINT('Ctrl Pts',(-14.8183427926634,639.625493671717,
59.8903489170524));
#101089=CARTESIAN_POINT('Ctrl Pts',(-14.6644248370209,639.508259656391,
59.4147167113827));
#101090=CARTESIAN_POINT('Ctrl Pts',(-14.4874575536325,639.374605578268,
58.9477239471356));
#101091=CARTESIAN_POINT('Ctrl Pts',(-14.4812763675599,639.369937253647,
58.9314126317608));
#101092=CARTESIAN_POINT('Ctrl Pts',(-14.4750668043185,639.365248739367,
58.9151121429094));
#101093=CARTESIAN_POINT('Ctrl Pts',(-14.4688293500763,639.360540436529,
58.898823461902));
#101094=CARTESIAN_POINT('Ctrl Pts',(-14.3830461531583,639.295787533528,
58.6748065671682));
#101095=CARTESIAN_POINT('Ctrl Pts',(-14.292004696505,639.227305326286,58.4530694500958));
#101096=CARTESIAN_POINT('Ctrl Pts',(-14.1969736437625,639.156141646841,
58.2361648853124));
#101097=CARTESIAN_POINT('Ctrl Pts',(-14.094982172067,639.079765681423,58.0033734435543));
#101098=CARTESIAN_POINT('Ctrl Pts',(-13.9880772628478,639.000060083224,
57.7752684237754));
#101099=CARTESIAN_POINT('Ctrl Pts',(-13.8764789934297,638.917311525991,
57.5515702123706));
#101100=CARTESIAN_POINT('Ctrl Pts',(-13.8680348690463,638.911050325764,
57.5346440043631));
#101101=CARTESIAN_POINT('Ctrl Pts',(-13.8595642190568,638.904771818041,
57.5177427581885));
#101102=CARTESIAN_POINT('Ctrl Pts',(-13.851067080703,638.898476101966,57.5008664006861));
#101103=CARTESIAN_POINT('Ctrl Pts',(-13.5414068385364,638.66904204037,56.8858432324675));
#101104=CARTESIAN_POINT('Ctrl Pts',(-13.1966130805598,638.416756255639,
56.3038699397583));
#101105=CARTESIAN_POINT('Ctrl Pts',(-12.818575693,638.146435853816,55.751526435915));
#101106=CARTESIAN_POINT('Ctrl Pts',(-12.6579969944544,638.031612030185,
55.5169078401994));
#101107=CARTESIAN_POINT('Ctrl Pts',(-12.4914199381867,637.913533811193,
55.2876357592445));
#101108=CARTESIAN_POINT('Ctrl Pts',(-12.3189883302193,637.792568574045,
55.0634499517658));
#101109=CARTESIAN_POINT('Ctrl Pts',(-12.3063145884526,637.783677616079,
55.046972270758));
#101110=CARTESIAN_POINT('Ctrl Pts',(-12.2936088752279,637.774770937369,
55.0305223394531));
#101111=CARTESIAN_POINT('Ctrl Pts',(-12.2808711596615,637.765848674103,
55.0141001141053));
#101112=CARTESIAN_POINT('Ctrl Pts',(-12.1059805186987,637.643344734276,
54.7886206313742));
#101113=CARTESIAN_POINT('Ctrl Pts',(-11.9251378242925,637.517956630315,
54.5684575845326));
#101114=CARTESIAN_POINT('Ctrl Pts',(-11.7381263934176,637.38994007246,54.3533266754976));
#101115=CARTESIAN_POINT('Ctrl Pts',(-11.6215708300055,637.310153281049,
54.2192455437048));
#101116=CARTESIAN_POINT('Ctrl Pts',(-11.5026183161313,637.229345080535,
54.0871197660045));
#101117=CARTESIAN_POINT('Ctrl Pts',(-11.3812089157723,637.147574159189,
53.9568866869203));
#101118=CARTESIAN_POINT('Ctrl Pts',(-11.3665916244721,637.137729210003,
53.941207053809));
#101119=CARTESIAN_POINT('Ctrl Pts',(-11.3519440806364,637.12787400806,53.9255610169989));
#101120=CARTESIAN_POINT('Ctrl Pts',(-11.3372665071724,637.118008888418,
53.9099486834451));
#101121=CARTESIAN_POINT('Ctrl Pts',(-11.1445926511122,636.988508556048,
53.7050041457592));
#101122=CARTESIAN_POINT('Ctrl Pts',(-10.9471021948171,636.857533215464,
53.5062326251667));
#101123=CARTESIAN_POINT('Ctrl Pts',(-10.7453127463482,636.725844068542,
53.3138226657878));
#101124=CARTESIAN_POINT('Ctrl Pts',(-10.6147258174797,636.640622163272,
53.1893056215636));
#101125=CARTESIAN_POINT('Ctrl Pts',(-10.4823376624354,636.55510092654,53.0674534899255));
#101126=CARTESIAN_POINT('Ctrl Pts',(-10.3482814114362,636.469484779022,
52.9483262480233));
#101127=CARTESIAN_POINT('Ctrl Pts',(-10.3323385786133,636.459302755307,
52.9341588691196));
#101128=CARTESIAN_POINT('Ctrl Pts',(-10.316370473426,636.449117709371,52.9200274595626));
#101129=CARTESIAN_POINT('Ctrl Pts',(-10.3003769198535,636.438929821937,
52.9059318994444));
#101130=CARTESIAN_POINT('Ctrl Pts',(-9.82420777099613,636.135610258463,
52.4862708882941));
#101131=CARTESIAN_POINT('Ctrl Pts',(-9.32605084320083,635.830070938416,
52.0987968357312));
#101132=CARTESIAN_POINT('Ctrl Pts',(-8.80356011328112,635.528334398778,
51.741914085228));
#101133=CARTESIAN_POINT('Ctrl Pts',(-8.55658179174747,635.385705295833,
51.5732176899501));
#101134=CARTESIAN_POINT('Ctrl Pts',(-8.3041668154036,635.24392537086,51.4113565816656));
#101135=CARTESIAN_POINT('Ctrl Pts',(-8.04607025545269,635.103627726854,
51.2561621006139));
#101136=CARTESIAN_POINT('Ctrl Pts',(-8.028503229707,635.094078539818,51.2455989786384));
#101137=CARTESIAN_POINT('Ctrl Pts',(-8.01090956281682,635.084536397273,
51.2350670302149));
#101138=CARTESIAN_POINT('Ctrl Pts',(-7.99328905883562,635.075001591146,
51.2245662881425));
#101139=CARTESIAN_POINT('Ctrl Pts',(-7.59780332812596,634.860996374697,
50.9888809946957));
#101140=CARTESIAN_POINT('Ctrl Pts',(-7.18882425917893,634.650689576269,
50.7689174218947));
#101141=CARTESIAN_POINT('Ctrl Pts',(-6.76412222102952,634.447355561283,
50.5650277071313));
#101142=CARTESIAN_POINT('Ctrl Pts',(-6.32001855033099,634.23473265317,50.3518237132473));
#101143=CARTESIAN_POINT('Ctrl Pts',(-5.86418599451931,634.032422703343,
50.1588849102784));
#101144=CARTESIAN_POINT('Ctrl Pts',(-5.39617905494653,633.845509050457,
49.9868909337916));
#101145=CARTESIAN_POINT('Ctrl Pts',(-5.37904744986588,633.838666991901,
49.980595016718));
#101146=CARTESIAN_POINT('Ctrl Pts',(-5.36189899496736,633.831845254971,
49.97432686759));
#101147=CARTESIAN_POINT('Ctrl Pts',(-5.34473356176537,633.82504412301,49.9680865467439));
#101148=CARTESIAN_POINT('Ctrl Pts',(-5.055056391868,633.710270867058,49.8627773208895));
#101149=CARTESIAN_POINT('Ctrl Pts',(-4.76048580671642,633.601340023833,
49.7653700783152));
#101150=CARTESIAN_POINT('Ctrl Pts',(-4.46054827634026,633.499656635932,
49.6761957671099));
#101151=CARTESIAN_POINT('Ctrl Pts',(-4.29218546502649,633.442579080384,
49.6261398847644));
#101152=CARTESIAN_POINT('Ctrl Pts',(-4.12213195857958,633.387784596201,
49.5786775358484));
#101153=CARTESIAN_POINT('Ctrl Pts',(-3.95030718844002,633.335516822509,
49.5338627639008));
#101154=CARTESIAN_POINT('Ctrl Pts',(-3.93446701216019,633.3306983627,49.5297313811729));
#101155=CARTESIAN_POINT('Ctrl Pts',(-3.91860807731799,633.325901021388,
49.5256222106105));
#101156=CARTESIAN_POINT('Ctrl Pts',(-3.90273095451649,633.321125135832,
49.5215354185999));
#101157=CARTESIAN_POINT('Ctrl Pts',(-3.55379715982543,633.216164817077,
49.431719407085));
#101158=CARTESIAN_POINT('Ctrl Pts',(-3.19571883737219,633.121498785814,
49.3526530596577));
#101159=CARTESIAN_POINT('Ctrl Pts',(-2.8343973414302,633.040693043213,49.2860999619196));
#101160=CARTESIAN_POINT('Ctrl Pts',(-2.69666016759681,633.009889576659,
49.2607296595842));
#101161=CARTESIAN_POINT('Ctrl Pts',(-2.55845161168197,632.981099853051,
49.2371774467707));
#101162=CARTESIAN_POINT('Ctrl Pts',(-2.42009779884018,632.954519815639,
49.2155398450577));
#101163=CARTESIAN_POINT('Ctrl Pts',(-2.40660419108441,632.9519274722,49.2134295359574));
#101164=CARTESIAN_POINT('Ctrl Pts',(-2.39310738388887,632.949355404132,
49.2113367450486));
#101165=CARTESIAN_POINT('Ctrl Pts',(-2.37960737536316,632.946803670967,
49.209261482295));
#101166=CARTESIAN_POINT('Ctrl Pts',(-1.98661162623389,632.872520733704,
49.1488489693019));
#101167=CARTESIAN_POINT('Ctrl Pts',(-1.59091824852693,632.815491657532,
49.1033073919242));
#101168=CARTESIAN_POINT('Ctrl Pts',(-1.19224235500595,632.777193216939,
49.0728901474769));
#101169=CARTESIAN_POINT('Ctrl Pts',(-1.07867395168118,632.766283370573,
49.0642253700436));
#101170=CARTESIAN_POINT('Ctrl Pts',(-0.964863484246403,632.756893701717,
49.0567881087321));
#101171=CARTESIAN_POINT('Ctrl Pts',(-0.850804267018436,632.74905893634,
49.0505847395294));
#101172=CARTESIAN_POINT('Ctrl Pts',(-0.467771498273324,632.722748288696,
49.0297526337247));
#101173=CARTESIAN_POINT('Ctrl Pts',(-0.0819322950834558,632.713989217867,
49.0228304603037));
#101174=CARTESIAN_POINT('Ctrl Pts',(0.306952880997389,632.723630147254,
49.0304624743333));
#101175=CARTESIAN_POINT('Ctrl Pts',(0.454443680668833,632.727286620868,
49.0333570353029));
#101176=CARTESIAN_POINT('Ctrl Pts',(0.602372687018365,632.733590203336,
49.0383454288014));
#101177=CARTESIAN_POINT('Ctrl Pts',(0.750753219933457,632.742588727813,
49.0454640244198));
#101178=CARTESIAN_POINT('Ctrl Pts',(0.757600042190907,632.743003952751,
49.0457925025427));
#101179=CARTESIAN_POINT('Ctrl Pts',(0.764445410940789,632.743424790216,
49.0461253700538));
#101180=CARTESIAN_POINT('Ctrl Pts',(0.771289326852132,632.743851229338,
49.0464626238936));
#101181=CARTESIAN_POINT('Ctrl Pts',(1.09992952098518,632.764328546383,49.0626573242443));
#101182=CARTESIAN_POINT('Ctrl Pts',(1.42500065454434,632.797705387382,49.0889528591549));
#101183=CARTESIAN_POINT('Ctrl Pts',(1.74665485812661,632.842753401007,49.1249902270789));
#101184=CARTESIAN_POINT('Ctrl Pts',(1.9493488062638,632.871140904219,49.1476995724057));
#101185=CARTESIAN_POINT('Ctrl Pts',(2.1506856598,632.904163981864,49.1742781049647));
#101186=CARTESIAN_POINT('Ctrl Pts',(2.35070124101388,632.941523180052,49.2046424827418));
#101187=CARTESIAN_POINT('Ctrl Pts',(2.52144209724989,632.973414402967,49.2305626627061));
#101188=CARTESIAN_POINT('Ctrl Pts',(2.6915051276523,633.008522435512,49.2592881187909));
#101189=CARTESIAN_POINT('Ctrl Pts',(2.86062884453507,633.046621855959,49.2907367311976));
#101190=CARTESIAN_POINT('Ctrl Pts',(3.03567001918768,633.086054334334,49.3232856968799));
#101191=CARTESIAN_POINT('Ctrl Pts',(3.20970492775773,633.128690992935,49.3587517991202));
#101192=CARTESIAN_POINT('Ctrl Pts',(3.38245717566776,633.174240520362,49.3970067274552));
#101193=CARTESIAN_POINT('Ctrl Pts',(3.54860965817462,633.218049889852,49.4338001781216));
#101194=CARTESIAN_POINT('Ctrl Pts',(3.71357570183427,633.264553196647,49.4731731008918));
#101195=CARTESIAN_POINT('Ctrl Pts',(3.87712128125395,633.313460490017,49.5149800517143));
#101196=CARTESIAN_POINT('Ctrl Pts',(3.87712128125394,633.313460490016,49.5149800517143));
#101197=CARTESIAN_POINT('Ctrl Pts',(4.87153021748849,633.610832324939,49.7691795549397));
#101198=CARTESIAN_POINT('Ctrl Pts',(5.79934294385505,633.989640531339,50.1085862160764));
#101199=CARTESIAN_POINT('Ctrl Pts',(7.12166692125997,634.616737672023,50.7337821806858));
#101200=CARTESIAN_POINT('Ctrl Pts',(7.55227759129253,634.836898028831,50.9628773512951));
#101201=CARTESIAN_POINT('Ctrl Pts',(8.38321347944639,635.285514008744,51.4559004400492));
#101202=CARTESIAN_POINT('Ctrl Pts',(8.78304187688083,635.513563386631,51.7192666405192));
#101203=CARTESIAN_POINT('Ctrl Pts',(9.94055760102618,636.200191042852,52.5603722809289));
#101204=CARTESIAN_POINT('Ctrl Pts',(10.6569237854819,636.661081997033,53.1884290403189));
#101205=CARTESIAN_POINT('Ctrl Pts',(11.6536196238761,637.330472386105,54.2454145926918));
#101206=CARTESIAN_POINT('Ctrl Pts',(11.9710603883753,637.548934443444,54.6156007098022));
#101207=CARTESIAN_POINT('Ctrl Pts',(12.5694073935915,637.967870605571,55.385215476498));
#101208=CARTESIAN_POINT('Ctrl Pts',(12.8514309701718,638.169106179423,55.7857953218243));
#101209=CARTESIAN_POINT('Ctrl Pts',(13.3802712808598,638.551424741988,56.6209194460713));
#101210=CARTESIAN_POINT('Ctrl Pts',(13.6270976333542,638.732524744703,57.0554488359468));
#101211=CARTESIAN_POINT('Ctrl Pts',(14.0830317948412,639.070375015612,57.9622402793));
#101212=CARTESIAN_POINT('Ctrl Pts',(14.288866825385,639.22469547035,58.4281588815737));
#101213=CARTESIAN_POINT('Ctrl Pts',(14.6541428180436,639.500434064949,59.3835018865815));
#101214=CARTESIAN_POINT('Ctrl Pts',(14.813802564089,639.622021221983,59.8733378707772));
#101215=CARTESIAN_POINT('Ctrl Pts',(15.0845904681104,639.829156459885,60.8791319779345));
#101216=CARTESIAN_POINT('Ctrl Pts',(15.1961319187924,639.9150275833,61.3988026843396));
#101217=CARTESIAN_POINT('Ctrl Pts',(15.445895886564,640.107734649545,62.9621091081608));
#101218=CARTESIAN_POINT('Ctrl Pts',(15.5031899681929,640.152399140232,64.0148308425101));
#101219=CARTESIAN_POINT('Ctrl Pts',(15.4344186449233,640.09911226955,65.3443173476824));
#101220=CARTESIAN_POINT('Ctrl Pts',(15.4134449473779,640.082865124052,65.6117770146501));
#101221=CARTESIAN_POINT('Ctrl Pts',(15.3578567110548,640.039860261308,66.1405396918101));
#101222=CARTESIAN_POINT('Ctrl Pts',(15.3232550273986,640.013112515011,66.4025181324823));
#101223=CARTESIAN_POINT('Ctrl Pts',(15.1997028143738,639.917778456694,67.1815043824831));
#101224=CARTESIAN_POINT('Ctrl Pts',(15.0910612840211,639.834128771633,67.6915802539796));
#101225=CARTESIAN_POINT('Ctrl Pts',(14.8233372862475,639.629293421513,68.694153518926));
#101226=CARTESIAN_POINT('Ctrl Pts',(14.6637788819681,639.50774336639,69.1878707203431));
#101227=CARTESIAN_POINT('Ctrl Pts',(14.2965526740649,639.2304637143,70.1529519783302));
#101228=CARTESIAN_POINT('Ctrl Pts',(14.0918748017888,639.07699695793,70.6169548967642));
#101229=CARTESIAN_POINT('Ctrl Pts',(13.4200658305586,638.578980164138,71.9594073502309));
#101230=CARTESIAN_POINT('Ctrl Pts',(12.8958575906797,638.196942223385,72.7887618167445));
#101231=CARTESIAN_POINT('Ctrl Pts',(12.0012587128913,637.569843325258,73.9468631187593));
#101232=CARTESIAN_POINT('Ctrl Pts',(11.683780665072,637.35107315101,74.3193541873481));
#101233=CARTESIAN_POINT('Ctrl Pts',(11.0214171690138,636.905565899513,75.0259744723523));
#101234=CARTESIAN_POINT('Ctrl Pts',(10.6774393735486,636.67938676523,75.3595543546866));
#101235=CARTESIAN_POINT('Ctrl Pts',(9.60714722132492,635.996881119879,76.3061032107106));
#101236=CARTESIAN_POINT('Ctrl Pts',(8.84327964705721,635.536024385843,76.865511939863));
#101237=CARTESIAN_POINT('Ctrl Pts',(7.60921202386664,634.866673624162,77.6043583167633));
#101238=CARTESIAN_POINT('Ctrl Pts',(7.1813427653491,634.646547948635,77.8345316034363));
#101239=CARTESIAN_POINT('Ctrl Pts',(6.29818432438025,634.224889583467,78.2566267740411));
#101240=CARTESIAN_POINT('Ctrl Pts',(5.84582286264931,634.024672538662,78.4473366643001));
#101241=CARTESIAN_POINT('Ctrl Pts',(4.91622538701958,633.654268625565,78.7878860584469));
#101242=CARTESIAN_POINT('Ctrl Pts',(4.43900471573538,633.484057011527,78.9377439866561));
#101243=CARTESIAN_POINT('Ctrl Pts',(3.45473183503186,633.184919007639,79.1941909352119));
#101244=CARTESIAN_POINT('Ctrl Pts',(2.94362350959894,633.055356583509,79.3013079500641));
#101245=CARTESIAN_POINT('Ctrl Pts',(1.90950562370682,632.856171648375,79.4634826852088));
#101246=CARTESIAN_POINT('Ctrl Pts',(1.38650131959488,632.786121706041,79.5190163918644));
#101247=CARTESIAN_POINT('Ctrl Pts',(0.592249243454403,632.731168797606,
79.5625292223074));
#101248=CARTESIAN_POINT('Ctrl Pts',(0.325874264894089,632.721192165362,
79.5703863596371));
#101249=CARTESIAN_POINT('Ctrl Pts',(-0.21025693007535,632.718683864069,
79.5723645937365));
#101250=CARTESIAN_POINT('Ctrl Pts',(-0.48111240188688,632.726286108066,
79.5663806670725));
#101251=CARTESIAN_POINT('Ctrl Pts',(-1.81787718546613,632.807108441004,
79.5024445409065));
#101252=CARTESIAN_POINT('Ctrl Pts',(-2.84910806661434,633.007947305093,
79.3448450590357));
#101253=CARTESIAN_POINT('Ctrl Pts',(-3.85030552837329,633.305466608637,
79.0907977188138));
#101254=CARTESIAN_POINT('Ctrl Pts',(-31.4841643694399,640.028384824678,
66.2394387527688));
#101255=CARTESIAN_POINT('Ctrl Pts',(-31.5102422866113,640.037345033595,
66.1500520616432));
#101256=CARTESIAN_POINT('Ctrl Pts',(-31.5344697491162,640.045722080512,
66.0600041335432));
#101257=CARTESIAN_POINT('Ctrl Pts',(-31.5568948002686,640.053514660279,
65.9693158656704));
#101258=CARTESIAN_POINT('Ctrl Pts',(-31.5799157801734,640.061514321951,
65.8762176257544));
#101259=CARTESIAN_POINT('Ctrl Pts',(-31.6010376935118,640.068898248738,
65.7824435675418));
#101260=CARTESIAN_POINT('Ctrl Pts',(-31.6202693727863,640.075651611604,
65.6879866773397));
#101261=CARTESIAN_POINT('Ctrl Pts',(-31.6248896050321,640.07727404428,65.6652942871582));
#101262=CARTESIAN_POINT('Ctrl Pts',(-31.6294005338969,640.078860015917,
65.6425623950765));
#101263=CARTESIAN_POINT('Ctrl Pts',(-31.6338018813918,640.080409188182,
65.6197907592958));
#101264=CARTESIAN_POINT('Ctrl Pts',(-31.654946100996,640.087851463219,65.5103950643971));
#101265=CARTESIAN_POINT('Ctrl Pts',(-31.6735752186302,640.094449440729,
65.3999871588139));
#101266=CARTESIAN_POINT('Ctrl Pts',(-31.6895226485726,640.100117970976,
65.2892446570257));
#101267=CARTESIAN_POINT('Ctrl Pts',(-31.7041726680797,640.105325335361,
65.1875116619713));
#101268=CARTESIAN_POINT('Ctrl Pts',(-31.7165598903944,640.109748371004,
65.085497360404));
#101269=CARTESIAN_POINT('Ctrl Pts',(-31.7265914867054,640.113333580631,
64.9837326301969));
#101270=CARTESIAN_POINT('Ctrl Pts',(-31.7270906099686,640.11351196316,64.9786693139858));
#101271=CARTESIAN_POINT('Ctrl Pts',(-31.7275839622651,640.113688290221,
64.9736061633852));
#101272=CARTESIAN_POINT('Ctrl Pts',(-31.7280715338081,640.113862555796,
64.9685432194279));
#101273=CARTESIAN_POINT('Ctrl Pts',(-31.764504511737,640.126884263006,64.5902230978285));
#101274=CARTESIAN_POINT('Ctrl Pts',(-31.7700166160656,640.128859737276,
64.2118862669711));
#101275=CARTESIAN_POINT('Ctrl Pts',(-31.7446624416281,640.119794168933,
63.8336029368517));
#101276=CARTESIAN_POINT('Ctrl Pts',(-31.7418698618535,640.118795661848,
63.7919377515238));
#101277=CARTESIAN_POINT('Ctrl Pts',(-31.7387028782001,640.117663227655,
63.7502732253699));
#101278=CARTESIAN_POINT('Ctrl Pts',(-31.7351615999219,640.116396885934,
63.7086094597171));
#101279=CARTESIAN_POINT('Ctrl Pts',(-31.7342761400163,640.11608025032,63.6981918672244));
#101280=CARTESIAN_POINT('Ctrl Pts',(-31.7333672691212,640.115755243257,
63.6877743355871));
#101281=CARTESIAN_POINT('Ctrl Pts',(-31.7324349885411,640.11542186466,63.6773568521116));
#101282=CARTESIAN_POINT('Ctrl Pts',(-31.7131811671587,640.108536800135,
63.4622109289096));
#101283=CARTESIAN_POINT('Ctrl Pts',(-31.683622095357,640.097991917248,63.245890825627));
#101284=CARTESIAN_POINT('Ctrl Pts',(-31.6441613654705,640.084079144946,
63.0327241328211));
#101285=CARTESIAN_POINT('Ctrl Pts',(-31.6075834037094,640.071182757711,
62.8351301410067));
#101286=CARTESIAN_POINT('Ctrl Pts',(-31.5626857917352,640.055459282476,
62.6406026984657));
#101287=CARTESIAN_POINT('Ctrl Pts',(-31.5096017754345,640.037144233563,
62.4489753179586));
#101288=CARTESIAN_POINT('Ctrl Pts',(-31.5054732129836,640.035719796821,
62.4340716678045));
#101289=CARTESIAN_POINT('Ctrl Pts',(-31.5012951264941,640.034279706936,
62.4191858432772));
#101290=CARTESIAN_POINT('Ctrl Pts',(-31.4970675917481,640.032824078575,
62.4043178063035));
#101291=CARTESIAN_POINT('Ctrl Pts',(-31.3960489687264,639.998041260346,
62.0490401534014));
#101292=CARTESIAN_POINT('Ctrl Pts',(-31.2670264883458,639.954378011182,
61.7038445239479));
#101293=CARTESIAN_POINT('Ctrl Pts',(-31.1086646817577,639.903345001752,
61.3690067539261));
#101294=CARTESIAN_POINT('Ctrl Pts',(-31.0920627526296,639.89799493393,61.3339038901288));
#101295=CARTESIAN_POINT('Ctrl Pts',(-31.0751383343455,639.892563878665,
61.2989148348993));
#101296=CARTESIAN_POINT('Ctrl Pts',(-31.0578898612242,639.887053582625,
61.2640398858555));
#101297=CARTESIAN_POINT('Ctrl Pts',(-31.0492646062338,639.884298109251,
61.246600352155));
#101298=CARTESIAN_POINT('Ctrl Pts',(-31.0405577742687,639.881522719423,
61.2291887088941));
#101299=CARTESIAN_POINT('Ctrl Pts',(-31.0317691561598,639.878727630602,
61.2118050194646));
#101300=CARTESIAN_POINT('Ctrl Pts',(-30.8901561041094,639.833689712945,
60.9316975798752));
#101301=CARTESIAN_POINT('Ctrl Pts',(-30.7301960856141,639.784493060366,
60.6647961351979));
#101302=CARTESIAN_POINT('Ctrl Pts',(-30.552570698745,639.732879161611,60.4117938284315));
#101303=CARTESIAN_POINT('Ctrl Pts',(-30.5000976258482,639.717631679708,
60.3370533382344));
#101304=CARTESIAN_POINT('Ctrl Pts',(-30.4460831214046,639.702173469663,
60.2635256557381));
#101305=CARTESIAN_POINT('Ctrl Pts',(-30.390545271495,639.686549959976,60.1912282413397));
#101306=CARTESIAN_POINT('Ctrl Pts',(-30.3775068190579,639.682882076032,
60.1742551968214));
#101307=CARTESIAN_POINT('Ctrl Pts',(-30.3643834596268,639.679204897354,
60.1573491022777));
#101308=CARTESIAN_POINT('Ctrl Pts',(-30.3511754754658,639.675519029086,
60.1405102847351));
#101309=CARTESIAN_POINT('Ctrl Pts',(-30.235121732026,639.643132647847,59.9925537315534));
#101310=CARTESIAN_POINT('Ctrl Pts',(-30.1123925773292,639.610042934629,
59.849656540082));
#101311=CARTESIAN_POINT('Ctrl Pts',(-29.9827850448132,639.57663347586,59.7120039038443));
#101312=CARTESIAN_POINT('Ctrl Pts',(-29.9677860070962,639.572767113138,
59.696073833711));
#101313=CARTESIAN_POINT('Ctrl Pts',(-29.9526930083797,639.568896032035,
59.6802121620136));
#101314=CARTESIAN_POINT('Ctrl Pts',(-29.9375060153829,639.565020925164,
59.6644195965418));
#101315=CARTESIAN_POINT('Ctrl Pts',(-29.8373419011642,639.539463091078,
59.5602614967747));
#101316=CARTESIAN_POINT('Ctrl Pts',(-29.7327995153621,639.513674609795,
59.458939882618));
#101317=CARTESIAN_POINT('Ctrl Pts',(-29.6252314154097,639.48817571714,59.3617773359258));
#101318=CARTESIAN_POINT('Ctrl Pts',(-29.5921376179513,639.480330871045,
59.3318848525389));
#101319=CARTESIAN_POINT('Ctrl Pts',(-29.5587577612501,639.47251345882,59.3023858391177));
#101320=CARTESIAN_POINT('Ctrl Pts',(-29.5251319616347,639.464738635874,
59.273318160203));
#101321=CARTESIAN_POINT('Ctrl Pts',(-29.5086752766871,639.460933586976,
59.2590922491607));
#101322=CARTESIAN_POINT('Ctrl Pts',(-29.4921556791454,639.457137728834,
59.244965869578));
#101323=CARTESIAN_POINT('Ctrl Pts',(-29.4755774290304,639.453352761744,
59.2309432594684));
#101324=CARTESIAN_POINT('Ctrl Pts',(-29.3099773946231,639.415544749685,
59.0908714967353));
#101325=CARTESIAN_POINT('Ctrl Pts',(-29.1378119106167,639.378613173181,
58.9601884052983));
#101326=CARTESIAN_POINT('Ctrl Pts',(-28.9590308976962,639.343172368862,
58.8390285950504));
#101327=CARTESIAN_POINT('Ctrl Pts',(-28.8087859082244,639.313388427128,
58.7372076347721));
#101328=CARTESIAN_POINT('Ctrl Pts',(-28.6538691499679,639.284657645377,
58.6421117181841));
#101329=CARTESIAN_POINT('Ctrl Pts',(-28.4942662542453,639.257346611503,
58.5537968335703));
#101330=CARTESIAN_POINT('Ctrl Pts',(-28.4769007957699,639.254375057494,
58.5441878070262));
#101331=CARTESIAN_POINT('Ctrl Pts',(-28.459478271223,639.251420060263,58.5346582250449));
#101332=CARTESIAN_POINT('Ctrl Pts',(-28.4419987306746,639.248482115936,
58.5252082343139));
#101333=CARTESIAN_POINT('Ctrl Pts',(-28.2888749865063,639.222745224608,
58.4424247103949));
#101334=CARTESIAN_POINT('Ctrl Pts',(-28.1308888550333,639.198321952111,
58.3657956999464));
#101335=CARTESIAN_POINT('Ctrl Pts',(-27.9696009617568,639.175673567212,
58.2959953699951));
#101336=CARTESIAN_POINT('Ctrl Pts',(-27.8035137347293,639.152351249782,
58.2241180392686));
#101337=CARTESIAN_POINT('Ctrl Pts',(-27.6339267596476,639.130911539138,
58.1594826664216));
#101338=CARTESIAN_POINT('Ctrl Pts',(-27.4625791838735,639.111850435863,
58.1027857638719));
#101339=CARTESIAN_POINT('Ctrl Pts',(-27.4162113318999,639.106692368051,
58.087443185648));
#101340=CARTESIAN_POINT('Ctrl Pts',(-27.3697146769788,639.101708413567,
58.0726816677735));
#101341=CARTESIAN_POINT('Ctrl Pts',(-27.3231238847891,639.096908229404,
58.0585144074595));
#101342=CARTESIAN_POINT('Ctrl Pts',(-27.3077052706593,639.095319671153,
58.0538259377042));
#101343=CARTESIAN_POINT('Ctrl Pts',(-27.2922743593198,639.093750967214,
58.0492017474521));
#101344=CARTESIAN_POINT('Ctrl Pts',(-27.2768323473444,639.092202478353,
58.0446423518745));
#101345=CARTESIAN_POINT('Ctrl Pts',(-27.0730982847699,639.071772502834,
57.9844880024676));
#101346=CARTESIAN_POINT('Ctrl Pts',(-26.8663796549633,639.054639627356,
57.9348961994572));
#101347=CARTESIAN_POINT('Ctrl Pts',(-26.6567340260135,639.041091703772,
57.8960408616036));
#101348=CARTESIAN_POINT('Ctrl Pts',(-26.4648399672041,639.028690939406,
57.8604755673283));
#101349=CARTESIAN_POINT('Ctrl Pts',(-26.270493782847,639.019293785622,57.8339051264844));
#101350=CARTESIAN_POINT('Ctrl Pts',(-26.0737540205691,639.013111701195,
57.8164286107964));
#101351=CARTESIAN_POINT('Ctrl Pts',(-26.0625619002153,639.01276001513,57.8154344077707));
#101352=CARTESIAN_POINT('Ctrl Pts',(-26.0513595866431,639.012418650729,
57.8144693989542));
#101353=CARTESIAN_POINT('Ctrl Pts',(-26.0401473720418,639.012087666317,
57.8135336570049));
#101354=CARTESIAN_POINT('Ctrl Pts',(-25.9356392028654,639.009002586677,
57.8048116799985));
#101355=CARTESIAN_POINT('Ctrl Pts',(-25.8309402583624,639.006848581643,
57.7987137325091));
#101356=CARTESIAN_POINT('Ctrl Pts',(-25.7263828388109,639.005616381943,
57.7952202807389));
#101357=CARTESIAN_POINT('Ctrl Pts',(-25.6276871999166,639.004453262796,
57.7919226816218));
#101358=CARTESIAN_POINT('Ctrl Pts',(-25.5291178586403,639.004111297681,
57.7909452136726));
#101359=CARTESIAN_POINT('Ctrl Pts',(-25.4309523482839,639.004568492207,
57.7922313210019));
#101360=CARTESIAN_POINT('Ctrl Pts',(-25.294918478184,639.005202054245,57.7940135575199));
#101361=CARTESIAN_POINT('Ctrl Pts',(-25.1593220246081,639.007368336825,
57.8001370969469));
#101362=CARTESIAN_POINT('Ctrl Pts',(-25.0241528026831,639.011027220461,
57.8105033392556));
#101363=CARTESIAN_POINT('Ctrl Pts',(-24.9473593427915,639.01310593579,57.8163926948472));
#101364=CARTESIAN_POINT('Ctrl Pts',(-24.8707038305026,639.015666741267,
57.8236523823281));
#101365=CARTESIAN_POINT('Ctrl Pts',(-24.7941852298226,639.01870474031,57.8322713177254));
#101366=CARTESIAN_POINT('Ctrl Pts',(-24.7886039418909,639.018926332802,
57.832899985261));
#101367=CARTESIAN_POINT('Ctrl Pts',(-24.783023664907,639.019150453516,57.8335358543738));
#101368=CARTESIAN_POINT('Ctrl Pts',(-24.7774444134025,639.019377099508,
57.8341789177943));
#101369=CARTESIAN_POINT('Ctrl Pts',(-24.5718967014472,639.02772706634,57.8578703062588));
#101370=CARTESIAN_POINT('Ctrl Pts',(-24.3672912611834,639.039490474857,
57.8913676774045));
#101371=CARTESIAN_POINT('Ctrl Pts',(-24.1636900166142,639.054489501827,
57.9346799113559));
#101372=CARTESIAN_POINT('Ctrl Pts',(-24.1607192710785,639.054708352613,
57.9353118801138));
#101373=CARTESIAN_POINT('Ctrl Pts',(-24.157748731861,639.054927892726,57.9359459397558));
#101374=CARTESIAN_POINT('Ctrl Pts',(-24.1547783995907,639.055148121579,
57.9365820902092));
#101375=CARTESIAN_POINT('Ctrl Pts',(-23.9761114704639,639.068394994095,
57.9748468490423));
#101376=CARTESIAN_POINT('Ctrl Pts',(-23.7981202073762,639.084173694413,
58.020803853977));
#101377=CARTESIAN_POINT('Ctrl Pts',(-23.6236786700018,639.101975805995,
58.073492891561));
#101378=CARTESIAN_POINT('Ctrl Pts',(-23.5968668085346,639.104712010667,
58.0815912561925));
#101379=CARTESIAN_POINT('Ctrl Pts',(-23.5701387392797,639.107495996677,
58.0898485859262));
#101380=CARTESIAN_POINT('Ctrl Pts',(-23.5435048114214,639.110325898878,
58.0982613196408));
#101381=CARTESIAN_POINT('Ctrl Pts',(-23.5429448698536,639.110385393666,
58.0984381857543));
#101382=CARTESIAN_POINT('Ctrl Pts',(-23.5423849693564,639.110444908808,
58.0986151207343));
#101383=CARTESIAN_POINT('Ctrl Pts',(-23.5418251100215,639.110504444289,
58.0987921245494));
#101384=CARTESIAN_POINT('Ctrl Pts',(-23.1762012421074,639.149384911802,
58.2143869097244));
#101385=CARTESIAN_POINT('Ctrl Pts',(-22.8243998969131,639.197144672671,
58.3597501602455));
#101386=CARTESIAN_POINT('Ctrl Pts',(-22.485780010064,639.251242388907,58.534088114487));
#101387=CARTESIAN_POINT('Ctrl Pts',(-22.4521163261309,639.256620479479,
58.5514198129993));
#101388=CARTESIAN_POINT('Ctrl Pts',(-22.4185829180421,639.262061250877,
58.5690378848413));
#101389=CARTESIAN_POINT('Ctrl Pts',(-22.3851791566599,639.267562233714,
58.5869415569959));
#101390=CARTESIAN_POINT('Ctrl Pts',(-22.3824169167542,639.268017123633,
58.5884220560666));
#101391=CARTESIAN_POINT('Ctrl Pts',(-22.3796555707751,639.268472436214,
58.5899045687243));
#101392=CARTESIAN_POINT('Ctrl Pts',(-22.3768951241845,639.268928168783,
58.5913890909715));
#101393=CARTESIAN_POINT('Ctrl Pts',(-22.2816916837795,639.284645664844,
58.6425879171943));
#101394=CARTESIAN_POINT('Ctrl Pts',(-22.1873305987372,639.300901973426,
58.6963061579081));
#101395=CARTESIAN_POINT('Ctrl Pts',(-22.0942798727876,639.317549730656,
58.7522616622872));
#101396=CARTESIAN_POINT('Ctrl Pts',(-22.0053194489196,639.333465689661,
58.8057574876718));
#101397=CARTESIAN_POINT('Ctrl Pts',(-21.9175571859603,639.349739080634,
58.8612974640396));
#101398=CARTESIAN_POINT('Ctrl Pts',(-21.8313793586397,639.366234879066,
58.9185972031316));
#101399=CARTESIAN_POINT('Ctrl Pts',(-21.7404851365708,639.383633470009,
58.9790328786581));
#101400=CARTESIAN_POINT('Ctrl Pts',(-21.6513542120641,639.401277476804,
59.0414157758743));
#101401=CARTESIAN_POINT('Ctrl Pts',(-21.5639768145986,639.419098754486,
59.1057211509867));
#101402=CARTESIAN_POINT('Ctrl Pts',(-21.4860588850607,639.434990702506,
59.1630648329029));
#101403=CARTESIAN_POINT('Ctrl Pts',(-21.4095352908753,639.451023925407,
59.2219381824051));
#101404=CARTESIAN_POINT('Ctrl Pts',(-21.3344208389071,639.467153202096,
59.2823508523678));
#101405=CARTESIAN_POINT('Ctrl Pts',(-21.3303712812063,639.468022760948,
59.2856078100699));
#101406=CARTESIAN_POINT('Ctrl Pts',(-21.3263252327256,639.468892694763,
59.2888695173619));
#101407=CARTESIAN_POINT('Ctrl Pts',(-21.3222826740452,639.469763001685,
59.2921359995237));
#101408=CARTESIAN_POINT('Ctrl Pts',(-21.0528504262188,639.52776803483,59.509843570628));
#101409=CARTESIAN_POINT('Ctrl Pts',(-20.8009946645294,639.586975366306,
59.7470704016645));
#101410=CARTESIAN_POINT('Ctrl Pts',(-20.5670888588777,639.645312005445,
60.004810465092));
#101411=CARTESIAN_POINT('Ctrl Pts',(-20.5213856139102,639.656710498533,
60.0551707253855));
#101412=CARTESIAN_POINT('Ctrl Pts',(-20.4763676412837,639.66807589812,60.1063140803729));
#101413=CARTESIAN_POINT('Ctrl Pts',(-20.432037699356,639.679392953574,60.1582478620834));
#101414=CARTESIAN_POINT('Ctrl Pts',(-20.4285403996402,639.680285784313,
60.1623450476902));
#101415=CARTESIAN_POINT('Ctrl Pts',(-20.4250475423573,639.68117828926,60.1664471954375));
#101416=CARTESIAN_POINT('Ctrl Pts',(-20.4215591732656,639.682070449002,
60.1705542466145));
#101417=CARTESIAN_POINT('Ctrl Pts',(-20.287610486405,639.716328184557,60.3282594944146));
#101418=CARTESIAN_POINT('Ctrl Pts',(-20.1603042570768,639.75007161128,60.4931698430411));
#101419=CARTESIAN_POINT('Ctrl Pts',(-20.0421702953158,639.782219628577,
60.6620380239489));
#101420=CARTESIAN_POINT('Ctrl Pts',(-20.039477867816,639.782952323938,60.6658867506599));
#101421=CARTESIAN_POINT('Ctrl Pts',(-20.0367898122911,639.783684290105,
60.6697379704284));
#101422=CARTESIAN_POINT('Ctrl Pts',(-20.0341061280847,639.784415522889,
60.6735916845282));
#101423=CARTESIAN_POINT('Ctrl Pts',(-19.9157181298536,639.816673113164,
60.8435943610537));
#101424=CARTESIAN_POINT('Ctrl Pts',(-19.8058462866112,639.847499911429,
61.0184341585709));
#101425=CARTESIAN_POINT('Ctrl Pts',(-19.7044789025187,639.876528688321,
61.1981599173521));
#101426=CARTESIAN_POINT('Ctrl Pts',(-19.7027270351528,639.877030374019,
61.2012660021588));
#101427=CARTESIAN_POINT('Ctrl Pts',(-19.7009776841107,639.87753152646,61.2043735352324));
#101428=CARTESIAN_POINT('Ctrl Pts',(-19.6992308514509,639.87803214358,61.2074825179746));
#101429=CARTESIAN_POINT('Ctrl Pts',(-19.5329119435344,639.925696750844,
61.5034940514717));
#101430=CARTESIAN_POINT('Ctrl Pts',(-19.3894177738832,639.968502028101,
61.8126262806501));
#101431=CARTESIAN_POINT('Ctrl Pts',(-19.2704812976807,640.004691234995,
62.1360898569805));
#101432=CARTESIAN_POINT('Ctrl Pts',(-19.2423582110331,640.013248342399,
62.2125743340303));
#101433=CARTESIAN_POINT('Ctrl Pts',(-19.2156080374183,640.021435685137,
62.2898599650054));
#101434=CARTESIAN_POINT('Ctrl Pts',(-19.1902534503917,640.029230307342,
62.3679625261942));
#101435=CARTESIAN_POINT('Ctrl Pts',(-4.39560350684949,633.478027683157,
78.9419118149793));
#101436=CARTESIAN_POINT('Ctrl Pts',(-4.65179838529719,633.049363360682,
79.3159462734001));
#101437=CARTESIAN_POINT('Ctrl Pts',(-4.46675582291307,633.642397176786,
79.3699798038619));
#101438=CARTESIAN_POINT('Ctrl Pts',(-3.22222729143504,633.085349971256,
79.2841755866806));
#101439=CARTESIAN_POINT('Ctrl Pts',(-3.35828013222165,632.570904879132,
79.710778768011));
#101440=CARTESIAN_POINT('Ctrl Pts',(-3.27436645787075,633.244650561051,
79.722255531377));
#101441=CARTESIAN_POINT('Ctrl Pts',(-2.00765458360981,632.817733196177,
79.4940431330352));
#101442=CARTESIAN_POINT('Ctrl Pts',(-2.13704517639042,632.270842624481,
79.9301149240665));
#101443=CARTESIAN_POINT('Ctrl Pts',(-2.04015348412621,632.973589782311,
79.9382527125224));
#101444=CARTESIAN_POINT('Ctrl Pts',(-0.46947699470708,632.726029746276,
79.5665829488807));
#101445=CARTESIAN_POINT('Ctrl Pts',(-0.504033715610802,632.159949720998,
80.0123807664003));
#101446=CARTESIAN_POINT('Ctrl Pts',(-0.477078115453726,632.880703862599,
80.0129132419871));
#101447=CARTESIAN_POINT('Ctrl Pts',(-0.198525207359669,632.718703826906,
79.5723490852243));
#101448=CARTESIAN_POINT('Ctrl Pts',(-0.213567627251543,632.151013403264,
80.0189726826106));
#101449=CARTESIAN_POINT('Ctrl Pts',(-0.201739610759609,632.873283461515,
80.018847964929));
#101450=CARTESIAN_POINT('Ctrl Pts',(0.337797886426132,632.721726429248,
79.569965145871));
#101451=CARTESIAN_POINT('Ctrl Pts',(0.363172475404082,632.154718369797,
80.01623327854));
#101452=CARTESIAN_POINT('Ctrl Pts',(0.343267231354877,632.876345052986,
80.016394319429));
#101453=CARTESIAN_POINT('Ctrl Pts',(0.604500980807282,632.731966644653,
79.5618998035946));
#101454=CARTESIAN_POINT('Ctrl Pts',(0.648999446052346,632.16720503038,80.0070154560596));
#101455=CARTESIAN_POINT('Ctrl Pts',(0.614288243293599,632.886717335452,
80.0080931677934));
#101456=CARTESIAN_POINT('Ctrl Pts',(1.40038494278016,632.787851132862,79.517642720174));
#101457=CARTESIAN_POINT('Ctrl Pts',(1.49988036818683,632.235238567253,79.9564789876384));
#101458=CARTESIAN_POINT('Ctrl Pts',(1.42305709514243,632.9433225857,79.9625420908729));
#101459=CARTESIAN_POINT('Ctrl Pts',(1.92534113326012,632.858717853151,79.4614512450883));
#101460=CARTESIAN_POINT('Ctrl Pts',(2.05434637538845,632.319756788193,79.8936395733644));
#101461=CARTESIAN_POINT('Ctrl Pts',(1.95650990903739,633.015102751413,79.9047081360849));
#101462=CARTESIAN_POINT('Ctrl Pts',(2.70496406063899,633.00998734159,79.3382254829299));
#101463=CARTESIAN_POINT('Ctrl Pts',(2.88633995891351,632.502364612948,79.7536174784857));
#101464=CARTESIAN_POINT('Ctrl Pts',(2.74875593427252,633.168323516404,79.777879100916));
#101465=CARTESIAN_POINT('Ctrl Pts',(2.96456958631008,633.068167782713,79.290410633663));
#101466=CARTESIAN_POINT('Ctrl Pts',(3.15905718679442,632.571231832849,79.7002947629951));
#101467=CARTESIAN_POINT('Ctrl Pts',(3.01256338076222,633.227254078587,79.7286663835033));
#101468=CARTESIAN_POINT('Ctrl Pts',(3.47518780032947,633.196825535093,79.1831150315862));
#101469=CARTESIAN_POINT('Ctrl Pts',(3.69386701621685,632.722884585209,79.5809202469059));
#101470=CARTESIAN_POINT('Ctrl Pts',(3.53144620093892,633.35757070182,79.6182338532211));
#101471=CARTESIAN_POINT('Ctrl Pts',(3.72621041294374,633.267215716703,79.1237090131227));
#101472=CARTESIAN_POINT('Ctrl Pts',(3.95514895647901,632.804991870565,79.5154433630724));
#101473=CARTESIAN_POINT('Ctrl Pts',(3.78653130909377,633.428868298287,79.5570911547537));
#101474=CARTESIAN_POINT('Ctrl Pts',(4.46772555015823,633.493945812143,78.9291150218726));
#101475=CARTESIAN_POINT('Ctrl Pts',(4.71519034053282,633.065022733312,79.3041392307203));
#101476=CARTESIAN_POINT('Ctrl Pts',(4.54004264997885,633.658520109168,79.3568092233317));
#101477=CARTESIAN_POINT('Ctrl Pts',(4.94672040811002,633.665752738284,78.7776297759102));
#101478=CARTESIAN_POINT('Ctrl Pts',(5.20619063282509,633.259960181782,79.1411907055206));
#101479=CARTESIAN_POINT('Ctrl Pts',(5.02678739774566,633.832540815926,79.2008962492214));
#101480=CARTESIAN_POINT('Ctrl Pts',(5.8792429321931,634.039167473233,78.4336864380197));
#101481=CARTESIAN_POINT('Ctrl Pts',(6.15788846175844,633.681186892879,78.7714177057809));
#101482=CARTESIAN_POINT('Ctrl Pts',(5.97439705300667,634.210767970231,78.8468983899839));
#101483=CARTESIAN_POINT('Ctrl Pts',(6.33275437617335,634.240803603263,78.241207083469));
#101484=CARTESIAN_POINT('Ctrl Pts',(6.61701333922231,633.904629068291,78.5679319403425));
#101485=CARTESIAN_POINT('Ctrl Pts',(6.43524462113633,634.415001804823,78.6487931851204));
#101486=CARTESIAN_POINT('Ctrl Pts',(7.21772555207048,634.665027590137,77.8154792735));
#101487=CARTESIAN_POINT('Ctrl Pts',(7.50949169824814,634.372005257329,78.1180713169069));
#101488=CARTESIAN_POINT('Ctrl Pts',(7.33453041364423,634.844691731002,78.2106205359385));
#101489=CARTESIAN_POINT('Ctrl Pts',(7.64567757896693,634.886000066787,77.5837558363346));
#101490=CARTESIAN_POINT('Ctrl Pts',(7.93961757498883,634.612643284557,77.8759092393284));
#101491=CARTESIAN_POINT('Ctrl Pts',(7.76940426542435,635.068510841072,77.9721240183561));
#101492=CARTESIAN_POINT('Ctrl Pts',(8.87989624832361,635.557552829048,76.8401851017735));
#101493=CARTESIAN_POINT('Ctrl Pts',(9.14486309090704,635.321780212489,77.1186234238837));
#101494=CARTESIAN_POINT('Ctrl Pts',(9.0235661087087,635.74870553549,77.2068280660124));
#101495=CARTESIAN_POINT('Ctrl Pts',(9.64297366367729,636.019085537869,76.277848672361));
#101496=CARTESIAN_POINT('Ctrl Pts',(9.91195517002788,635.815649296021,76.5412806704512));
#101497=CARTESIAN_POINT('Ctrl Pts',(9.79898624522685,636.216183412484,76.6280570123386));
#101498=CARTESIAN_POINT('Ctrl Pts',(10.7111493226909,636.701555729233,75.3274439525344));
#101499=CARTESIAN_POINT('Ctrl Pts',(10.996929204677,636.553856661763,75.5414473133398));
#101500=CARTESIAN_POINT('Ctrl Pts',(10.8844475000821,636.907453239766,75.6498569210074));
#101501=CARTESIAN_POINT('Ctrl Pts',(11.0542671299848,636.927552573915,74.9926611496337));
#101502=CARTESIAN_POINT('Ctrl Pts',(11.3383050337577,636.792333613069,75.1981903967951));
#101503=CARTESIAN_POINT('Ctrl Pts',(11.2331134421883,637.136361142634,75.3052878963191));
#101504=CARTESIAN_POINT('Ctrl Pts',(11.7146199608134,637.372368504535,74.2838589448406));
#101505=CARTESIAN_POINT('Ctrl Pts',(11.9934013858358,637.259648873769,74.4717373421274));
#101506=CARTESIAN_POINT('Ctrl Pts',(11.9041426976532,637.586906313537,74.5757653364059));
#101507=CARTESIAN_POINT('Ctrl Pts',(12.0280511690333,637.588636973812,73.9137447966116));
#101508=CARTESIAN_POINT('Ctrl Pts',(12.3052838069643,637.486813840008,74.0929439227344));
#101509=CARTESIAN_POINT('Ctrl Pts',(12.2226419987782,637.805960726912,74.1948314957367));
#101510=CARTESIAN_POINT('Ctrl Pts',(12.9129429279531,638.209511050012,72.7621724811206));
#101511=CARTESIAN_POINT('Ctrl Pts',(13.1682069587253,638.125157961639,72.9350760877257));
#101512=CARTESIAN_POINT('Ctrl Pts',(13.1218292556881,638.434824297819,73.0096082212392));
#101513=CARTESIAN_POINT('Ctrl Pts',(13.4325731745126,638.588343288914,71.9369957714403));
#101514=CARTESIAN_POINT('Ctrl Pts',(13.691058719412,638.52474293751,72.0905203676822));
#101515=CARTESIAN_POINT('Ctrl Pts',(13.6498656696272,638.818539589406,72.1603061192183));
#101516=CARTESIAN_POINT('Ctrl Pts',(14.0995518794942,639.0829155774,70.5995413985153));
#101517=CARTESIAN_POINT('Ctrl Pts',(14.3599543505595,639.04443639772,70.7113989853479));
#101518=CARTESIAN_POINT('Ctrl Pts',(14.3276327741606,639.319486592683,70.7837383555535));
#101519=CARTESIAN_POINT('Ctrl Pts',(14.3029634008898,639.235458993974,70.136985137629));
#101520=CARTESIAN_POINT('Ctrl Pts',(14.5622961369223,639.203195170246,70.2399143740041));
#101521=CARTESIAN_POINT('Ctrl Pts',(14.5343332153866,639.47399527342,70.3076585181821));
#101522=CARTESIAN_POINT('Ctrl Pts',(14.6682015611194,639.511275540645,69.174113632982));
#101523=CARTESIAN_POINT('Ctrl Pts',(14.9241336165254,639.488901670915,69.2600256603411));
#101524=CARTESIAN_POINT('Ctrl Pts',(14.9054756223491,639.753364437729,69.3166364965849));
#101525=CARTESIAN_POINT('Ctrl Pts',(14.8267650211877,639.632077828551,68.6819292751415));
#101526=CARTESIAN_POINT('Ctrl Pts',(15.0820212400289,639.614532434591,68.7582297164531));
#101527=CARTESIAN_POINT('Ctrl Pts',(15.0666029583495,639.875723200025,68.8100615928647));
#101528=CARTESIAN_POINT('Ctrl Pts',(15.0928587745384,639.835676376718,67.6825720627153));
#101529=CARTESIAN_POINT('Ctrl Pts',(15.345642317407,639.82511616596,67.7418790685988));
#101530=CARTESIAN_POINT('Ctrl Pts',(15.3369981776382,640.081944211076,67.781486615588));
#101531=CARTESIAN_POINT('Ctrl Pts',(15.2008187183865,639.918802146937,67.1742916843792));
#101532=CARTESIAN_POINT('Ctrl Pts',(15.4531593768323,639.911476842323,67.2238371821344));
#101533=CARTESIAN_POINT('Ctrl Pts',(15.4467037685615,640.166141047895,67.2583447276789));
#101534=CARTESIAN_POINT('Ctrl Pts',(15.3236190583423,640.013555762971,66.3983126284387));
#101535=CARTESIAN_POINT('Ctrl Pts',(15.5750769362233,640.009593564889,66.4333318182824));
#101536=CARTESIAN_POINT('Ctrl Pts',(15.5714893985198,640.262115321071,66.4596770533946));
#101537=CARTESIAN_POINT('Ctrl Pts',(15.3580154032569,640.0401443868,66.1373887935008));
#101538=CARTESIAN_POINT('Ctrl Pts',(15.6092008209444,640.037099666513,66.1679286147603));
#101539=CARTESIAN_POINT('Ctrl Pts',(15.6064418001331,640.289046455888,66.191124442761));
#101540=CARTESIAN_POINT('Ctrl Pts',(15.4132989948751,640.082912766178,65.6108481462777));
#101541=CARTESIAN_POINT('Ctrl Pts',(15.6639728424716,640.081280555054,65.6327189571251));
#101542=CARTESIAN_POINT('Ctrl Pts',(15.6626190527797,640.332365724081,65.649189292362));
#101543=CARTESIAN_POINT('Ctrl Pts',(15.4341736765461,640.099082778176,65.3445748221907));
#101544=CARTESIAN_POINT('Ctrl Pts',(15.6846836179855,640.098005681656,65.361885527254));
#101545=CARTESIAN_POINT('Ctrl Pts',(15.6838311981551,640.34874403735,65.37513074784));
#101546=CARTESIAN_POINT('Ctrl Pts',(15.5027734069943,640.152235313522,64.0208357993163));
#101547=CARTESIAN_POINT('Ctrl Pts',(15.7525074770034,640.152789798181,64.019253662881));
#101548=CARTESIAN_POINT('Ctrl Pts',(15.7535397227803,640.402581126806,64.0126917270571));
#101549=CARTESIAN_POINT('Ctrl Pts',(15.4463052101678,640.10821736367,62.972460326068));
#101550=CARTESIAN_POINT('Ctrl Pts',(15.6953430710373,640.106377717465,62.9419553492361));
#101551=CARTESIAN_POINT('Ctrl Pts',(15.6961577000033,640.357995398756,62.9336548017417));
#101552=CARTESIAN_POINT('Ctrl Pts',(15.1990606178882,639.917447559145,61.4152823525307));
#101553=CARTESIAN_POINT('Ctrl Pts',(15.4514130025606,639.910073207687,61.3655583025674));
#101554=CARTESIAN_POINT('Ctrl Pts',(15.4449172446521,640.164769008981,61.3309552205203));
#101555=CARTESIAN_POINT('Ctrl Pts',(15.0885616588025,639.832373608348,60.897431997035));
#101556=CARTESIAN_POINT('Ctrl Pts',(15.3413681900166,639.821688428962,60.8377615984788));
#101557=CARTESIAN_POINT('Ctrl Pts',(15.3326315846512,640.078598890309,60.7979635436387));
#101558=CARTESIAN_POINT('Ctrl Pts',(14.8199878745666,639.626907879806,59.894490282593));
#101559=CARTESIAN_POINT('Ctrl Pts',(15.0752901365765,639.609169825034,59.8177577361634));
#101560=CARTESIAN_POINT('Ctrl Pts',(15.0597162431557,639.870486649284,59.7656992724498));
#101561=CARTESIAN_POINT('Ctrl Pts',(14.6615322304544,639.506218060285,59.405821548259));
#101562=CARTESIAN_POINT('Ctrl Pts',(14.9175497152663,639.48368395994,59.3196546068316));
#101563=CARTESIAN_POINT('Ctrl Pts',(14.8986984980326,639.748241829529,59.2627428795189));
#101564=CARTESIAN_POINT('Ctrl Pts',(14.2987645730368,639.2323098162,58.452368034267));
#101565=CARTESIAN_POINT('Ctrl Pts',(14.5581603558448,639.199949590199,58.3493442354962));
#101566=CARTESIAN_POINT('Ctrl Pts',(14.5300665302068,639.470805547583,58.2814141988727));
#101567=CARTESIAN_POINT('Ctrl Pts',(14.0943650477466,639.079019607747,57.987427888935));
#101568=CARTESIAN_POINT('Ctrl Pts',(14.3547106916411,639.040317082871,57.8751573631045));
#101569=CARTESIAN_POINT('Ctrl Pts',(14.3223620118629,639.315540381266,57.8028805682137));
#101570=CARTESIAN_POINT('Ctrl Pts',(13.6407992303396,638.7427973154,57.0811428907972));
#101571=CARTESIAN_POINT('Ctrl Pts',(13.905352230957,638.691285108647,56.9519457897139));
#101572=CARTESIAN_POINT('Ctrl Pts',(13.8614639308801,638.97498749143,56.870100046218));
#101573=CARTESIAN_POINT('Ctrl Pts',(13.3950963108816,638.562439030259,56.6466171892939));
#101574=CARTESIAN_POINT('Ctrl Pts',(13.660997958786,638.503183284432,56.5087094937084));
#101575=CARTESIAN_POINT('Ctrl Pts',(13.611788274916,638.792305710012,56.4228707819826));
#101576=CARTESIAN_POINT('Ctrl Pts',(12.8683162606274,638.181402354979,55.8111128357767));
#101577=CARTESIAN_POINT('Ctrl Pts',(13.1390236076535,638.106466963312,55.6564090278324));
#101578=CARTESIAN_POINT('Ctrl Pts',(13.0764921418282,638.406361283186,55.5629408541681));
#101579=CARTESIAN_POINT('Ctrl Pts',(12.5872314290769,637.980708173654,55.4101487566788));
#101580=CARTESIAN_POINT('Ctrl Pts',(12.8594650095397,637.896519710106,55.2468622237164));
#101581=CARTESIAN_POINT('Ctrl Pts',(12.7908624053289,638.203081725356,55.1502548367754));
#101582=CARTESIAN_POINT('Ctrl Pts',(11.9905202907966,637.562607910276,54.6394524585066));
#101583=CARTESIAN_POINT('Ctrl Pts',(12.2679641743712,637.459493978226,54.4591095196187));
#101584=CARTESIAN_POINT('Ctrl Pts',(12.1845042755668,637.779596359876,54.3570282351227));
#101585=CARTESIAN_POINT('Ctrl Pts',(11.6738674877948,637.344499438125,54.2686527469967));
#101586=CARTESIAN_POINT('Ctrl Pts',(11.9529310376215,637.230395235121,54.0796602679055));
#101587=CARTESIAN_POINT('Ctrl Pts',(11.8627313233714,637.558678274829,53.9753888666545));
#101588=CARTESIAN_POINT('Ctrl Pts',(10.6782856421904,636.675211836513,53.2086614405224));
#101589=CARTESIAN_POINT('Ctrl Pts',(10.945265328937,636.512855335653,52.9711566209328));
#101590=CARTESIAN_POINT('Ctrl Pts',(10.8510402072694,636.880761580352,52.8843970456025));
#101591=CARTESIAN_POINT('Ctrl Pts',(9.9619956407393,636.213789414038,52.5782081758289));
#101592=CARTESIAN_POINT('Ctrl Pts',(10.2261851601175,636.022124234935,52.325672618392));
#101593=CARTESIAN_POINT('Ctrl Pts',(10.1231644802855,636.41339474604,52.2355170621796));
#101594=CARTESIAN_POINT('Ctrl Pts',(8.80321427157986,635.525430893182,51.7332383677212));
#101595=CARTESIAN_POINT('Ctrl Pts',(9.09775647626564,635.303078691545,51.4706442472987));
#101596=CARTESIAN_POINT('Ctrl Pts',(8.94566114499843,635.716178886036,51.3658592810726));
#101597=CARTESIAN_POINT('Ctrl Pts',(8.40274055580763,635.296654083887,51.468542205798));
#101598=CARTESIAN_POINT('Ctrl Pts',(8.69719315797,635.057159081061,51.1963055952873));
#101599=CARTESIAN_POINT('Ctrl Pts',(8.53871075522488,635.484455070077,51.0934261046552));
#101600=CARTESIAN_POINT('Ctrl Pts',(7.56992268932879,634.846289649222,50.9728170395581));
#101601=CARTESIAN_POINT('Ctrl Pts',(7.86343028959298,634.569343605214,50.6785875112157));
#101602=CARTESIAN_POINT('Ctrl Pts',(7.69242405624649,635.028288789374,50.5832101346318));
#101603=CARTESIAN_POINT('Ctrl Pts',(7.13789769244056,634.625016491671,50.7422564476865));
#101604=CARTESIAN_POINT('Ctrl Pts',(7.42930129741495,634.32828122725,50.4376325390388));
#101605=CARTESIAN_POINT('Ctrl Pts',(7.25341144010781,634.804165183149,50.3459105384044));
#101606=CARTESIAN_POINT('Ctrl Pts',(5.64937448274455,633.917920325537,50.0365737439137));
#101607=CARTESIAN_POINT('Ctrl Pts',(5.86838675369824,633.517703145266,49.6620231583277));
#101608=CARTESIAN_POINT('Ctrl Pts',(5.74078325583842,634.087945275018,49.619586152077));
#101609=CARTESIAN_POINT('Ctrl Pts',(4.53678997843346,633.475322195353,49.6490480272297));
#101610=CARTESIAN_POINT('Ctrl Pts',(4.73821803522549,633.030778025867,49.2624552965428));
#101611=CARTESIAN_POINT('Ctrl Pts',(4.6102062721931,633.639651657831,49.2207424753189));
#101612=CARTESIAN_POINT('Ctrl Pts',(3.32305067587215,633.158508245587,49.3839240770566));
#101613=CARTESIAN_POINT('Ctrl Pts',(3.5382678177423,632.678855162063,48.9831770877134));
#101614=CARTESIAN_POINT('Ctrl Pts',(3.3768462630334,633.318759264595,48.9478721490979));
#101615=CARTESIAN_POINT('',(3.93978362444746,633.475903764133,49.082928510463));
#101616=CARTESIAN_POINT('Origin',(3.87712128127698,633.475903764132,49.3249479946959));
#101617=CARTESIAN_POINT('',(3.44556542901615E-11,632.874615496758,80.0177796115133));
#101618=CARTESIAN_POINT('Ctrl Pts',(6.89110032669561E-11,632.874615496766,
80.0177787907144));
#101619=CARTESIAN_POINT('Ctrl Pts',(0.0236086443784427,632.874614137695,
80.0177797817517));
#101620=CARTESIAN_POINT('Ctrl Pts',(0.0471977207100217,632.874679616131,
80.0177272377913));
#101621=CARTESIAN_POINT('Ctrl Pts',(0.0707638231545093,632.874812004893,
80.017621142111));
#101622=CARTESIAN_POINT('Ctrl Pts',(0.343491007326591,632.876344121384,
80.0163933117468));
#101623=CARTESIAN_POINT('Ctrl Pts',(0.614496441609097,632.886726575974,
80.0080814531982));
#101624=CARTESIAN_POINT('Ctrl Pts',(0.883878526644417,632.90557635702,79.992909437795));
#101625=CARTESIAN_POINT('Ctrl Pts',(1.24943310899451,632.931155726327,79.9723208386927));
#101626=CARTESIAN_POINT('Ctrl Pts',(1.61199825336115,632.972352866,79.9391295369995));
#101627=CARTESIAN_POINT('Ctrl Pts',(1.97182100459663,633.027965414741,79.8936222931219));
#101628=CARTESIAN_POINT('Ctrl Pts',(2.14338863407486,633.054482118102,79.8719239154363));
#101629=CARTESIAN_POINT('Ctrl Pts',(2.31433265226697,633.084276807937,79.8474250872979));
#101630=CARTESIAN_POINT('Ctrl Pts',(2.48467918176861,633.117222497334,79.8201546029834));
#101631=CARTESIAN_POINT('Ctrl Pts',(2.64668359998503,633.148554789569,79.7942195929849));
#101632=CARTESIAN_POINT('Ctrl Pts',(2.80854164377702,633.182836792382,79.7656811760263));
#101633=CARTESIAN_POINT('Ctrl Pts',(2.96931905952992,633.219691119353,79.7347565578901));
#101634=CARTESIAN_POINT('Ctrl Pts',(3.07072240523473,633.242935379383,79.7152522031959));
#101635=CARTESIAN_POINT('Ctrl Pts',(3.17169670908156,633.267201801138,79.6947984620929));
#101636=CARTESIAN_POINT('Ctrl Pts',(3.27200870695423,633.292396349908,79.6734492843488));
#101637=CARTESIAN_POINT('Ctrl Pts',(3.53149735464351,633.357570003389,79.6182228968818));
#101638=CARTESIAN_POINT('Ctrl Pts',(3.78656458821259,633.428865125024,79.5570823750604));
#101639=CARTESIAN_POINT('Ctrl Pts',(4.0377054944055,633.50540597798,79.4903295169232));
#101640=CARTESIAN_POINT('Ctrl Pts',(4.40729347692622,633.618046247752,79.3920936120663));
#101641=CARTESIAN_POINT('Ctrl Pts',(4.76841289981949,633.741996318891,79.2817479196209));
#101642=CARTESIAN_POINT('Ctrl Pts',(5.12226678865164,633.875000842973,79.1597571080153));
#101643=CARTESIAN_POINT('Ctrl Pts',(5.24929534886485,633.922747593057,79.1159641255257));
#101644=CARTESIAN_POINT('Ctrl Pts',(5.37538735228987,633.971661476884,79.0706700669597));
#101645=CARTESIAN_POINT('Ctrl Pts',(5.50059773443487,634.021638914138,79.0238952610022));
#101646=CARTESIAN_POINT('Ctrl Pts',(5.57281046246084,634.050462459135,78.9969187732444));
#101647=CARTESIAN_POINT('Ctrl Pts',(5.64472953797076,634.079640403287,78.9694492784864));
#101648=CARTESIAN_POINT('Ctrl Pts',(5.71636225209789,634.109157580105,78.9414864057523));
#101649=CARTESIAN_POINT('Ctrl Pts',(6.11454307894412,634.273233086873,78.7860507235792));
#101650=CARTESIAN_POINT('Ctrl Pts',(6.5037096819656,634.447710875873,78.6154339417837));
#101651=CARTESIAN_POINT('Ctrl Pts',(6.8848883010362,634.629844770744,78.4297064786912));
#101652=CARTESIAN_POINT('Ctrl Pts',(7.33445681558759,634.844656568862,78.2106563653939));
#101653=CARTESIAN_POINT('Ctrl Pts',(7.76935072835594,635.068481784423,77.9721566871374));
#101654=CARTESIAN_POINT('Ctrl Pts',(8.187458217611,635.295242394859,77.7170253648745));
#101655=CARTESIAN_POINT('Ctrl Pts',(8.18746947767835,635.295248501757,77.717018493924));
#101656=CARTESIAN_POINT('Ctrl Pts',(8.18748073773472,635.295254608657,77.717011622961));
#101657=CARTESIAN_POINT('Ctrl Pts',(8.18749199778011,635.29526071556,77.7170047519856));
#101658=CARTESIAN_POINT('Ctrl Pts',(8.77466513792119,635.613714974938,77.3587067097642));
#101659=CARTESIAN_POINT('Ctrl Pts',(9.33198431948961,635.939124765157,76.966537584401));
#101660=CARTESIAN_POINT('Ctrl Pts',(9.86244451563549,636.264283914362,76.5388820043299));
#101661=CARTESIAN_POINT('Ctrl Pts',(10.0299804477179,636.366979350387,76.4038149875433));
#101662=CARTESIAN_POINT('Ctrl Pts',(10.1948374647139,636.469649728038,76.2652085142118));
#101663=CARTESIAN_POINT('Ctrl Pts',(10.357110568178,636.572067980441,76.1230125476066));
#101664=CARTESIAN_POINT('Ctrl Pts',(10.4125855674164,636.607080883706,76.0744011574826));
#101665=CARTESIAN_POINT('Ctrl Pts',(10.4677585361306,636.642065479229,76.0253703145275));
#101666=CARTESIAN_POINT('Ctrl Pts',(10.5226333425913,636.677012430926,75.9759179749726));
#101667=CARTESIAN_POINT('Ctrl Pts',(10.8021362240136,636.855013490539,75.7240342365111));
#101668=CARTESIAN_POINT('Ctrl Pts',(11.0737787493323,637.032122690786,75.4611186031081));
#101669=CARTESIAN_POINT('Ctrl Pts',(11.3375596732538,637.207320538843,75.1864000604822));
#101670=CARTESIAN_POINT('Ctrl Pts',(11.4152479295857,637.258919476045,75.1054904774791));
#101671=CARTESIAN_POINT('Ctrl Pts',(11.4922757377262,637.310368726257,75.023534546417));
#101672=CARTESIAN_POINT('Ctrl Pts',(11.5686281331514,637.361633525872,74.9405265476199));
#101673=CARTESIAN_POINT('Ctrl Pts',(11.7428614430288,637.478617880682,74.7511053998464));
#101674=CARTESIAN_POINT('Ctrl Pts',(11.9125329809655,637.593944005337,74.5572877444706));
#101675=CARTESIAN_POINT('Ctrl Pts',(12.0772418647245,637.707053445441,74.3595533209396));
#101676=CARTESIAN_POINT('Ctrl Pts',(12.1335432671804,637.745716934401,74.2919630058059));
#101677=CARTESIAN_POINT('Ctrl Pts',(12.1892651384294,637.784121561834,74.2239153125423));
#101678=CARTESIAN_POINT('Ctrl Pts',(12.2443925060635,637.822245533895,74.1554302041703));
#101679=CARTESIAN_POINT('Ctrl Pts',(12.3387364620062,637.887490193579,74.0382260581302));
#101680=CARTESIAN_POINT('Ctrl Pts',(12.4314151262027,637.951963329841,73.9196466444437));
#101681=CARTESIAN_POINT('Ctrl Pts',(12.5223735539977,638.015572404099,73.7997538153798));
#101682=CARTESIAN_POINT('Ctrl Pts',(12.7691297819456,638.188134041407,73.4745030060267));
#101683=CARTESIAN_POINT('Ctrl Pts',(13.0038431244469,638.354709108044,73.1391451429892));
#101684=CARTESIAN_POINT('Ctrl Pts',(13.2260892248535,638.514262005761,72.7931543850006));
#101685=CARTESIAN_POINT('Ctrl Pts',(13.4204829916068,638.653819409589,72.490523893018));
#101686=CARTESIAN_POINT('Ctrl Pts',(13.6053390538305,638.788004415294,72.1797589167343));
#101687=CARTESIAN_POINT('Ctrl Pts',(13.7803977512332,638.916136677922,71.8605255759729));
#101688=CARTESIAN_POINT('Ctrl Pts',(13.8914471872943,638.997418075061,71.6580181713742));
#101689=CARTESIAN_POINT('Ctrl Pts',(13.9985704807448,639.076258682161,71.4520750410272));
#101690=CARTESIAN_POINT('Ctrl Pts',(14.1017118649645,639.152494301075,71.242591313036));
#101691=CARTESIAN_POINT('Ctrl Pts',(14.2070716057042,639.230369589492,71.0286020260264));
#101692=CARTESIAN_POINT('Ctrl Pts',(14.3082384476158,639.305518787928,70.81089177479));
#101693=CARTESIAN_POINT('Ctrl Pts',(14.4050208561385,639.377709197237,70.5892424956487));
#101694=CARTESIAN_POINT('Ctrl Pts',(14.5157812425591,639.46032583959,70.3355811104624));
#101695=CARTESIAN_POINT('Ctrl Pts',(14.6208678960897,639.539123655019,70.0765942455148));
#101696=CARTESIAN_POINT('Ctrl Pts',(14.7199048617496,639.61367514778,69.8121463246681));
#101697=CARTESIAN_POINT('Ctrl Pts',(14.7921227929364,639.668038228658,69.6193104312928));
#101698=CARTESIAN_POINT('Ctrl Pts',(14.8606224440704,639.71976485242,69.4248390807865));
#101699=CARTESIAN_POINT('Ctrl Pts',(14.9252970870176,639.768724787416,69.2290149637919));
#101700=CARTESIAN_POINT('Ctrl Pts',(15.0269343231625,639.845666108592,68.9212742308732));
#101701=CARTESIAN_POINT('Ctrl Pts',(15.1192104490316,639.915845082243,68.6099443406549));
#101702=CARTESIAN_POINT('Ctrl Pts',(15.2018005707495,639.978833650544,68.2957740937441));
#101703=CARTESIAN_POINT('Ctrl Pts',(15.3370175067359,640.081958831023,67.781413086861));
#101704=CARTESIAN_POINT('Ctrl Pts',(15.446711258392,640.16614656396,67.2582968021332));
#101705=CARTESIAN_POINT('Ctrl Pts',(15.5298941967001,640.230123458173,66.7258995592192));
#101706=CARTESIAN_POINT('Ctrl Pts',(15.5492380442097,640.245001019737,66.6020927871707));
#101707=CARTESIAN_POINT('Ctrl Pts',(15.567145084157,640.258784059514,66.4777831582835));
#101708=CARTESIAN_POINT('Ctrl Pts',(15.5835932838998,640.271451481493,66.3529610769457));
#101709=CARTESIAN_POINT('Ctrl Pts',(15.6025152015847,640.286024013424,66.2093664474262));
#101710=CARTESIAN_POINT('Ctrl Pts',(15.6195051466467,640.299119194904,66.0651039293665));
#101711=CARTESIAN_POINT('Ctrl Pts',(15.6345304353988,640.310705016247,65.9201567812727));
#101712=CARTESIAN_POINT('Ctrl Pts',(15.6626204963928,640.332364927982,65.6491753513615));
#101713=CARTESIAN_POINT('Ctrl Pts',(15.6838314901426,640.348739893915,65.3751252063361));
#101714=CARTESIAN_POINT('Ctrl Pts',(15.6977729274255,640.359499433045,65.1026424621912));
#101715=CARTESIAN_POINT('Ctrl Pts',(15.7020662908531,640.362812908611,65.0187294893299));
#101716=CARTESIAN_POINT('Ctrl Pts',(15.7056890266772,640.365606360559,64.934880886641));
#101717=CARTESIAN_POINT('Ctrl Pts',(15.7086425189985,640.367881244341,64.8510957582209));
#101718=CARTESIAN_POINT('Ctrl Pts',(15.7263165930932,640.381494438539,64.3497148820873));
#101719=CARTESIAN_POINT('Ctrl Pts',(15.7200248924218,640.376502649213,63.8506118554521));
#101720=CARTESIAN_POINT('Ctrl Pts',(15.690054723568,640.35337768455,63.3537494689463));
#101721=CARTESIAN_POINT('Ctrl Pts',(15.6600845547142,640.330252719886,62.8568870824406));
#101722=CARTESIAN_POINT('Ctrl Pts',(15.6064372952925,640.288992245354,62.3622858632638));
#101723=CARTESIAN_POINT('Ctrl Pts',(15.5294020172295,640.229744984429,61.8699005539026));
#101724=CARTESIAN_POINT('Ctrl Pts',(15.5291562735781,640.229555984809,61.8683298376432));
#101725=CARTESIAN_POINT('Ctrl Pts',(15.5289102911643,640.229366802534,61.8667591390815));
#101726=CARTESIAN_POINT('Ctrl Pts',(15.5286640699994,640.229177437613,61.8651884582589));
#101727=CARTESIAN_POINT('Ctrl Pts',(15.4868770628328,640.197039691489,61.5986230278086));
#101728=CARTESIAN_POINT('Ctrl Pts',(15.4379580369842,640.159463399778,61.3322197252253));
#101729=CARTESIAN_POINT('Ctrl Pts',(15.3824805581748,640.11694984057,61.0681260116128));
#101730=CARTESIAN_POINT('Ctrl Pts',(15.3358122267536,640.081186916342,60.8459671605322));
#101731=CARTESIAN_POINT('Ctrl Pts',(15.2845038713041,640.041930974165,60.6254434697092));
#101732=CARTESIAN_POINT('Ctrl Pts',(15.2289186178845,639.999496500196,60.4078240107633));
#101733=CARTESIAN_POINT('Ctrl Pts',(15.2181659569586,639.991287785077,60.3657267258008));
#101734=CARTESIAN_POINT('Ctrl Pts',(15.2072508201014,639.982958720179,60.3237283373609));
#101735=CARTESIAN_POINT('Ctrl Pts',(15.196175503333,639.974511334344,60.2818374278755));
#101736=CARTESIAN_POINT('Ctrl Pts',(15.0967816925709,639.898701505458,59.9058935865296));
#101737=CARTESIAN_POINT('Ctrl Pts',(14.9842779945857,639.813199116241,59.5366531114232));
#101738=CARTESIAN_POINT('Ctrl Pts',(14.8591459849512,639.718652910703,59.1739255763155));
#101739=CARTESIAN_POINT('Ctrl Pts',(14.8126284390092,639.683505569327,59.0390824228484));
#101740=CARTESIAN_POINT('Ctrl Pts',(14.7643660978975,639.647108703488,58.9051391515317));
#101741=CARTESIAN_POINT('Ctrl Pts',(14.7143850694044,639.609496653593,58.7720853460318));
#101742=CARTESIAN_POINT('Ctrl Pts',(14.5736911865015,639.503620774218,58.3975461039397));
#101743=CARTESIAN_POINT('Ctrl Pts',(14.4193228109465,639.388070847762,58.0299622878074));
#101744=CARTESIAN_POINT('Ctrl Pts',(14.2516172400983,639.263553359904,57.6694867820626));
#101745=CARTESIAN_POINT('Ctrl Pts',(14.1996634649568,639.224978889583,57.5578145026341));
#101746=CARTESIAN_POINT('Ctrl Pts',(14.1464260882526,639.185541476775,57.4468157386464));
#101747=CARTESIAN_POINT('Ctrl Pts',(14.0919132979964,639.145261719478,57.3364909682744));
#101748=CARTESIAN_POINT('Ctrl Pts',(13.9337411446871,639.028387570924,57.0163769838124));
#101749=CARTESIAN_POINT('Ctrl Pts',(13.7664884987757,638.905649173198,56.7052436349986));
#101750=CARTESIAN_POINT('Ctrl Pts',(13.5905541920495,638.777739522865,56.4024860662582));
#101751=CARTESIAN_POINT('Ctrl Pts',(13.5102146755004,638.719330224185,56.2642333447919));
#101752=CARTESIAN_POINT('Ctrl Pts',(13.4280641419558,638.659838944025,56.1277259803299));
#101753=CARTESIAN_POINT('Ctrl Pts',(13.3441406912912,638.599331136345,55.9929065938881));
#101754=CARTESIAN_POINT('Ctrl Pts',(13.18094216384,638.481666943148,55.7307352321897));
#101755=CARTESIAN_POINT('Ctrl Pts',(13.0110358717025,638.360152379953,55.4749525005651));
#101756=CARTESIAN_POINT('Ctrl Pts',(12.834515971694,638.235208319465,55.2252918717908));
#101757=CARTESIAN_POINT('Ctrl Pts',(12.72157305542,638.155265227711,55.065551244863));
#101758=CARTESIAN_POINT('Ctrl Pts',(12.605960880953,638.073943984384,54.908370053597));
#101759=CARTESIAN_POINT('Ctrl Pts',(12.4876834913283,637.991338466186,54.7536417333294));
#101760=CARTESIAN_POINT('Ctrl Pts',(12.3260424195162,637.878447536303,54.5421858362462));
#101761=CARTESIAN_POINT('Ctrl Pts',(12.1591272633341,637.762955719753,54.3349982249623));
#101762=CARTESIAN_POINT('Ctrl Pts',(11.9873446890174,637.645441249947,54.1324570254279));
#101763=CARTESIAN_POINT('Ctrl Pts',(11.8370887041422,637.542652870694,53.9552968708841));
#101764=CARTESIAN_POINT('Ctrl Pts',(11.6829923400669,637.438237648866,53.7815611779533));
#101765=CARTESIAN_POINT('Ctrl Pts',(11.5255012613247,637.332705058659,53.6117252605926));
#101766=CARTESIAN_POINT('Ctrl Pts',(11.3711873179765,637.229301422869,53.445315516375));
#101767=CARTESIAN_POINT('Ctrl Pts',(11.2140552717419,637.125076575966,53.2829927429756));
#101768=CARTESIAN_POINT('Ctrl Pts',(11.0542019754068,637.020337990515,53.1247785161058));
#101769=CARTESIAN_POINT('Ctrl Pts',(10.5698058923565,636.702953477967,52.6453492297812));
#101770=CARTESIAN_POINT('Ctrl Pts',(10.0592926792999,636.38008853675,52.2024986100953));
#101771=CARTESIAN_POINT('Ctrl Pts',(9.52149128320355,636.057785926617,51.7931946715343));
#101772=CARTESIAN_POINT('Ctrl Pts',(9.4607314186001,636.021372739342,51.7469522257744));
#101773=CARTESIAN_POINT('Ctrl Pts',(9.39962327575445,635.984966737236,51.7011379284146));
#101774=CARTESIAN_POINT('Ctrl Pts',(9.33816519001716,635.948576638187,51.6557473746706));
#101775=CARTESIAN_POINT('Ctrl Pts',(9.21814549218717,635.877511478259,51.5671054900537));
#101776=CARTESIAN_POINT('Ctrl Pts',(9.09677553395677,635.806510933312,51.4800960735065));
#101777=CARTESIAN_POINT('Ctrl Pts',(8.97400639050294,635.735660278011,51.3947159850713));
#101778=CARTESIAN_POINT('Ctrl Pts',(8.6952662635268,635.57479802794,51.200865510741));
#101779=CARTESIAN_POINT('Ctrl Pts',(8.40931705214077,635.414676812656,51.0154168364813));
#101780=CARTESIAN_POINT('Ctrl Pts',(8.11558835298555,635.256319777099,50.8383307562355));
#101781=CARTESIAN_POINT('Ctrl Pts',(7.6923917485449,635.028163114403,50.5831897772666));
#101782=CARTESIAN_POINT('Ctrl Pts',(7.2533699333788,634.803988668472,50.3458922881572));
#101783=CARTESIAN_POINT('Ctrl Pts',(6.8038425239994,634.591170154752,50.1300393648259));
#101784=CARTESIAN_POINT('Ctrl Pts',(6.73473828265152,634.558454325575,50.0968570667095));
#101785=CARTESIAN_POINT('Ctrl Pts',(6.66535065282463,634.525974001608,50.0641473617017));
#101786=CARTESIAN_POINT('Ctrl Pts',(6.59567017408014,634.493749398169,50.0319141884441));
#101787=CARTESIAN_POINT('Ctrl Pts',(6.0329269890491,634.233501818042,49.7715973980109));
#101788=CARTESIAN_POINT('Ctrl Pts',(5.45113667983874,633.989769248135,49.5423875083977));
#101789=CARTESIAN_POINT('Ctrl Pts',(4.84525727421132,633.772994795064,49.3462933887937));
#101790=CARTESIAN_POINT('Ctrl Pts',(4.54937241807388,633.667131685566,49.2505296446731));
#101791=CARTESIAN_POINT('Ctrl Pts',(4.24774282927289,633.567697202977,49.1626636005312));
#101792=CARTESIAN_POINT('Ctrl Pts',(3.93978362444749,633.475903764133,49.082928510463));
#101793=CARTESIAN_POINT('',(-3.91253447320281,633.467807133627,79.5230488432747));
#101794=CARTESIAN_POINT('Ctrl Pts',(-3.91253447320281,633.467807133627,
79.5230488432747));
#101795=CARTESIAN_POINT('Ctrl Pts',(-3.28597810505974,633.282223705224,
79.6840769479877));
#101796=CARTESIAN_POINT('Ctrl Pts',(-2.64771851246926,633.133689622239,
79.807103090937));
#101797=CARTESIAN_POINT('Ctrl Pts',(-1.67000646568519,632.980744450827,
79.9322661229594));
#101798=CARTESIAN_POINT('Ctrl Pts',(-1.34070899812117,632.941409107268,
79.9640509087433));
#101799=CARTESIAN_POINT('Ctrl Pts',(-0.674809016948164,632.888311307288,
80.0068322484697));
#101800=CARTESIAN_POINT('Ctrl Pts',(-0.336249102370441,632.874615496751,
80.0177804323122));
#101801=CARTESIAN_POINT('Ctrl Pts',(0.,632.874615496751,80.0177804323122));
#101802=CARTESIAN_POINT('Origin',(-3.85030552837329,633.467807133627,79.2809175598242));
#101803=CARTESIAN_POINT('Ctrl Pts',(1.86306288877797,634.816577773823,79.840079036097));
#101804=CARTESIAN_POINT('Ctrl Pts',(1.88043236474458,634.745314120185,79.9049255377571));
#101805=CARTESIAN_POINT('Ctrl Pts',(1.89318255568148,634.648256234279,79.9033522554387));
#101806=CARTESIAN_POINT('Ctrl Pts',(0.807589904959711,634.674153210188,
79.96967854764));
#101807=CARTESIAN_POINT('Ctrl Pts',(0.818743950698479,634.603422866382,
80.0328500715449));
#101808=CARTESIAN_POINT('Ctrl Pts',(0.820646498012554,634.507527220826,
80.0334805824724));
#101809=CARTESIAN_POINT('Ctrl Pts',(-0.24578162409436,634.652430501916,
79.9884448322078));
#101810=CARTESIAN_POINT('Ctrl Pts',(-0.250591804105093,634.58145862555,
80.0516667261813));
#101811=CARTESIAN_POINT('Ctrl Pts',(-0.249753392942155,634.486062895163,
80.0523236519829));
#101812=CARTESIAN_POINT('Ctrl Pts',(-1.82283398292192,634.801279095755,
79.8541299127167));
#101813=CARTESIAN_POINT('Ctrl Pts',(-1.84045202787124,634.730077912528,
79.9187905906115));
#101814=CARTESIAN_POINT('Ctrl Pts',(-1.85230285694165,634.633139639668,
79.9174605062689));
#101815=CARTESIAN_POINT('Ctrl Pts',(-2.35132258925576,634.881814269216,
79.7811312873554));
#101816=CARTESIAN_POINT('Ctrl Pts',(-2.37466264357766,634.810809328746,
79.8462807686186));
#101817=CARTESIAN_POINT('Ctrl Pts',(-2.38933484362825,634.712715932409,
79.8441641306276));
#101818=CARTESIAN_POINT('Ctrl Pts',(-3.37688542676327,635.092028016582,
79.5855704382192));
#101819=CARTESIAN_POINT('Ctrl Pts',(-3.41016272286989,635.021031352354,
79.6525292086393));
#101820=CARTESIAN_POINT('Ctrl Pts',(-3.43147735551063,634.920427161253,
79.6478052879441));
#101821=CARTESIAN_POINT('Ctrl Pts',(-3.87715892282217,635.221574909017,
79.4630988338053));
#101822=CARTESIAN_POINT('Ctrl Pts',(-3.91596185111128,635.150913347198,
79.5308660063145));
#101823=CARTESIAN_POINT('Ctrl Pts',(-3.93983799323763,635.048431634461,
79.524834163758));
#101824=CARTESIAN_POINT('Ctrl Pts',(-4.85600136127738,635.519479195749,
79.1715962336162));
#101825=CARTESIAN_POINT('Ctrl Pts',(-4.90487000526279,635.449018256018,
79.2419298822336));
#101826=CARTESIAN_POINT('Ctrl Pts',(-4.93450429122365,635.342789420971,
79.2321422141563));
#101827=CARTESIAN_POINT('Ctrl Pts',(-5.33696096117466,635.688816137699,
79.0015116750124));
#101828=CARTESIAN_POINT('Ctrl Pts',(-5.39138050124868,635.618861104025,
79.0729171785271));
#101829=CARTESIAN_POINT('Ctrl Pts',(-5.42323859046884,635.51011019859,79.0613640029475));
#101830=CARTESIAN_POINT('Ctrl Pts',(-6.26683249734681,636.052464199552,
78.6207327915938));
#101831=CARTESIAN_POINT('Ctrl Pts',(-6.33161473347313,635.983087692133,
78.6952414948338));
#101832=CARTESIAN_POINT('Ctrl Pts',(-6.36814164931804,635.869428991425,
78.6790317667906));
#101833=CARTESIAN_POINT('Ctrl Pts',(-6.71485606394656,636.246122485711,
78.4107691833072));
#101834=CARTESIAN_POINT('Ctrl Pts',(-6.78508370064264,636.177428409817,
78.4865227570079));
#101835=CARTESIAN_POINT('Ctrl Pts',(-6.82340725268958,636.060781547509,
78.4682119648795));
#101836=CARTESIAN_POINT('Ctrl Pts',(-8.01567130514643,636.849983611819,
77.7247225905372));
#101837=CARTESIAN_POINT('Ctrl Pts',(-8.10998737994435,636.786710672416,
77.80127117446));
#101838=CARTESIAN_POINT('Ctrl Pts',(-8.1452439447473,636.65745105782,77.7793700065673));
#101839=CARTESIAN_POINT('Ctrl Pts',(-8.82586458852353,637.282584832603,
77.1932211322336));
#101840=CARTESIAN_POINT('Ctrl Pts',(-8.9322668123389,637.222864399076,77.2695206334129));
#101841=CARTESIAN_POINT('Ctrl Pts',(-8.96853196172092,637.084900724076,
77.2457034968301));
#101842=CARTESIAN_POINT('Ctrl Pts',(-9.96920498164766,637.941263310567,
76.2792128579425));
#101843=CARTESIAN_POINT('Ctrl Pts',(-10.0844043143261,637.880534079776,
76.3668461206141));
#101844=CARTESIAN_POINT('Ctrl Pts',(-10.1303565945194,637.735739871643,
76.3279647989551));
#101845=CARTESIAN_POINT('Ctrl Pts',(-10.3376554216138,638.162400261368,
75.9549308895933));
#101846=CARTESIAN_POINT('Ctrl Pts',(-10.4588442149254,638.103340264843,
76.0434598022962));
#101847=CARTESIAN_POINT('Ctrl Pts',(-10.5047617063462,637.95424377021,76.0023613348043));
#101848=CARTESIAN_POINT('Ctrl Pts',(-11.0382031181792,638.595577836314,
75.2772723636161));
#101849=CARTESIAN_POINT('Ctrl Pts',(-11.1717706789499,638.540193855464,
75.367843846083));
#101850=CARTESIAN_POINT('Ctrl Pts',(-11.2166306018809,638.382263478537,
75.3219412047776));
#101851=CARTESIAN_POINT('Ctrl Pts',(-11.3720692100036,638.808639459202,
74.9225466233422));
#101852=CARTESIAN_POINT('Ctrl Pts',(-11.5117299914058,638.755294583093,
75.0135259579074));
#101853=CARTESIAN_POINT('Ctrl Pts',(-11.5558920129995,638.592788120577,
74.9657703096301));
#101854=CARTESIAN_POINT('Ctrl Pts',(-12.3258306637108,639.431272311957,
73.8086323110397));
#101855=CARTESIAN_POINT('Ctrl Pts',(-12.4934838485425,639.390510009471,
73.890709901465));
#101856=CARTESIAN_POINT('Ctrl Pts',(-12.5250601941573,639.208003600421,
73.8473239435239));
#101857=CARTESIAN_POINT('Ctrl Pts',(-12.8992879967844,639.824973080161,
72.9992994563982));
#101858=CARTESIAN_POINT('Ctrl Pts',(-13.077744970774,639.788629846106,73.078286707878));
#101859=CARTESIAN_POINT('Ctrl Pts',(-13.1077845770232,639.597016725675,
73.0346961932179));
#101860=CARTESIAN_POINT('Ctrl Pts',(-13.9074241048782,640.534546099924,
71.2282105920088));
#101861=CARTESIAN_POINT('Ctrl Pts',(-14.1129332121864,640.511006048043,
71.2991153875746));
#101862=CARTESIAN_POINT('Ctrl Pts',(-14.1322077025265,640.298139145848,
71.2563976137341));
#101863=CARTESIAN_POINT('Ctrl Pts',(-14.3263939594619,640.839310439365,
70.2940353094581));
#101864=CARTESIAN_POINT('Ctrl Pts',(-14.5401918741479,640.819432608961,
70.3605898861845));
#101865=CARTESIAN_POINT('Ctrl Pts',(-14.5579479788688,640.599275304904,
70.3184194820128));
#101866=CARTESIAN_POINT('Ctrl Pts',(-14.8207085214835,641.20293089409,68.8119251561665));
#101867=CARTESIAN_POINT('Ctrl Pts',(-15.0476696916695,641.189657317405,
68.873414318539));
#101868=CARTESIAN_POINT('Ctrl Pts',(-15.0602487335032,640.958565966149,
68.8302748068456));
#101869=CARTESIAN_POINT('Ctrl Pts',(-14.9632961223424,641.308768600142,
68.3027032249751));
#101870=CARTESIAN_POINT('Ctrl Pts',(-15.1947954692114,641.297980576062,
68.3589101018559));
#101871=CARTESIAN_POINT('Ctrl Pts',(-15.2051396204071,641.063143179964,
68.3189814008671));
#101872=CARTESIAN_POINT('Ctrl Pts',(-15.1980890660801,641.483791241123,
67.2613296018157));
#101873=CARTESIAN_POINT('Ctrl Pts',(-15.4382600058939,641.477993541957,
67.3038920930527));
#101874=CARTESIAN_POINT('Ctrl Pts',(-15.443724690614,641.23608096797,67.273372933676));
#101875=CARTESIAN_POINT('Ctrl Pts',(-15.2886130183545,641.551710847139,
66.7373033136078));
#101876=CARTESIAN_POINT('Ctrl Pts',(-15.5318361040901,641.54764077895,66.7735722504368));
#101877=CARTESIAN_POINT('Ctrl Pts',(-15.535710856414,641.303191662114,66.7472152886529));
#101878=CARTESIAN_POINT('Ctrl Pts',(-15.416753347311,641.648007675455,65.6826183891459));
#101879=CARTESIAN_POINT('Ctrl Pts',(-15.6650029770328,641.646911132633,
65.702986948441));
#101880=CARTESIAN_POINT('Ctrl Pts',(-15.6659206532499,641.398341361037,
65.6882422743292));
#101881=CARTESIAN_POINT('Ctrl Pts',(-15.4543691947642,641.676387664944,
65.1519598739898));
#101882=CARTESIAN_POINT('Ctrl Pts',(-15.7039435893065,641.67605647301,65.1652840040138));
#101883=CARTESIAN_POINT('Ctrl Pts',(-15.7041440786651,641.426383341139,
65.1554257032332));
#101884=CARTESIAN_POINT('Ctrl Pts',(-15.4758420566949,641.692577105787,
64.0838805525614));
#101885=CARTESIAN_POINT('Ctrl Pts',(-15.7262805762301,641.692762772545,
64.0801660974848));
#101886=CARTESIAN_POINT('Ctrl Pts',(-15.725963719193,641.442379922507,64.0830042219837));
#101887=CARTESIAN_POINT('Ctrl Pts',(-15.4595256835684,641.680254533958,
63.5443861522047));
#101888=CARTESIAN_POINT('Ctrl Pts',(-15.7093899474742,641.680108047155,
63.533432145575));
#101889=CARTESIAN_POINT('Ctrl Pts',(-15.7093838004202,641.430204112855,
63.5413158590829));
#101890=CARTESIAN_POINT('Ctrl Pts',(-15.3271559384047,641.580597626596,
61.9287880982582));
#101891=CARTESIAN_POINT('Ctrl Pts',(-15.5720423635035,641.577531969054,
61.8961392504176));
#101892=CARTESIAN_POINT('Ctrl Pts',(-15.5748761636817,641.331734267035,
61.9191477303746));
#101893=CARTESIAN_POINT('Ctrl Pts',(-15.1321164848615,641.43365154733,60.8870337307209));
#101894=CARTESIAN_POINT('Ctrl Pts',(-15.3728291173235,641.428596909895,
60.8481294183498));
#101895=CARTESIAN_POINT('Ctrl Pts',(-15.3766850183768,641.186537362943,
60.8731529828927));
#101896=CARTESIAN_POINT('Ctrl Pts',(-14.6914127541727,641.107583316918,
59.3724502436072));
#101897=CARTESIAN_POINT('Ctrl Pts',(-14.9137106754241,641.091687521186,
59.3061798598269));
#101898=CARTESIAN_POINT('Ctrl Pts',(-14.9288646952281,640.864354185543,
59.352414428403));
#101899=CARTESIAN_POINT('Ctrl Pts',(-14.5183989336226,640.980317513494,
58.8731518928978));
#101900=CARTESIAN_POINT('Ctrl Pts',(-14.7354925923479,640.961660459604,
58.8024640384097));
#101901=CARTESIAN_POINT('Ctrl Pts',(-14.7530559724391,640.738604035086,
58.8510846321663));
#101902=CARTESIAN_POINT('Ctrl Pts',(-14.1306968197733,640.698218654891,
57.9103117242868));
#101903=CARTESIAN_POINT('Ctrl Pts',(-14.3355486906423,640.673080740323,
57.831412861111));
#101904=CARTESIAN_POINT('Ctrl Pts',(-14.359091214726,640.459865155437,57.8843269848985));
#101905=CARTESIAN_POINT('Ctrl Pts',(-13.9157951809153,640.543213567675,
57.4449987770471));
#101906=CARTESIAN_POINT('Ctrl Pts',(-14.1147768511431,640.515153086481,
57.36307554632));
#101907=CARTESIAN_POINT('Ctrl Pts',(-14.1407177531073,640.306706015409,
57.4171203625588));
#101908=CARTESIAN_POINT('Ctrl Pts',(-13.4461019523439,640.2091391353,56.5440307949745));
#101909=CARTESIAN_POINT('Ctrl Pts',(-13.6319576862834,640.174660971835,
56.4571863827656));
#101910=CARTESIAN_POINT('Ctrl Pts',(-13.6634366702206,639.976610327696,
56.5124852728988));
#101911=CARTESIAN_POINT('Ctrl Pts',(-13.1913037235795,640.030055873436,
56.1083842943529));
#101912=CARTESIAN_POINT('Ctrl Pts',(-13.3709792891118,639.992762314905,
56.0198511196711));
#101913=CARTESIAN_POINT('Ctrl Pts',(-13.4045217018065,639.79965965408,56.0750652474453));
#101914=CARTESIAN_POINT('Ctrl Pts',(-12.64240759359,639.651151524472,55.2652320085852));
#101915=CARTESIAN_POINT('Ctrl Pts',(-12.8086534652092,639.607949925527,
55.1745452490493));
#101916=CARTESIAN_POINT('Ctrl Pts',(-12.8467572513285,639.42526762927,55.228479858422));
#101917=CARTESIAN_POINT('Ctrl Pts',(-12.3483069071172,639.451372577967,
54.8582156625017));
#101918=CARTESIAN_POINT('Ctrl Pts',(-12.5081763747874,639.405559223045,
54.7668256888036));
#101919=CARTESIAN_POINT('Ctrl Pts',(-12.5479044351808,639.22786764373,54.8198060554334));
#101920=CARTESIAN_POINT('Ctrl Pts',(-11.4236939741492,638.837407783853,
53.6980435355989));
#101921=CARTESIAN_POINT('Ctrl Pts',(-11.5721545818984,638.789502601269,
53.6169046527624));
#101922=CARTESIAN_POINT('Ctrl Pts',(-11.6083463397431,638.621210776527,
53.6549020913344));
#101923=CARTESIAN_POINT('Ctrl Pts',(-10.7466675601512,638.404972777793,
52.9971756449448));
#101924=CARTESIAN_POINT('Ctrl Pts',(-10.8838506687482,638.353029612216,
52.9147405141668));
#101925=CARTESIAN_POINT('Ctrl Pts',(-10.9203783533487,638.193924822611,
52.9511800330592));
#101926=CARTESIAN_POINT('Ctrl Pts',(-9.63611348815389,637.746715461555,
52.043761533861));
#101927=CARTESIAN_POINT('Ctrl Pts',(-9.74600809350944,637.684740757834,
51.957512201222));
#101928=CARTESIAN_POINT('Ctrl Pts',(-9.79188180091537,637.543508391082,
51.9938845551591));
#101929=CARTESIAN_POINT('Ctrl Pts',(-9.24839501364177,637.524950639754,
51.7415264001437));
#101930=CARTESIAN_POINT('Ctrl Pts',(-9.3523814388582,637.46152901563,51.6563518525185));
#101931=CARTESIAN_POINT('Ctrl Pts',(-9.39789698724149,637.324384062376,
51.6904175829392));
#101932=CARTESIAN_POINT('Ctrl Pts',(-8.45164641908639,637.090734943436,
51.1790240815796));
#101933=CARTESIAN_POINT('Ctrl Pts',(-8.5442188058991,637.02515789963,51.0970442175137));
#101934=CARTESIAN_POINT('Ctrl Pts',(-8.58827076396017,636.895338174316,
51.1256218197328));
#101935=CARTESIAN_POINT('Ctrl Pts',(-8.04152694278709,636.87756046477,50.9176054756285));
#101936=CARTESIAN_POINT('Ctrl Pts',(-8.12841996224353,636.810886545792,
50.8368346325361));
#101937=CARTESIAN_POINT('Ctrl Pts',(-8.17152248677754,636.684701860634,
50.863137499133));
#101938=CARTESIAN_POINT('Ctrl Pts',(-6.77296527985932,636.258719991593,
50.1910295542293));
#101939=CARTESIAN_POINT('Ctrl Pts',(-6.85180078127632,636.193927906267,
50.1198420410442));
#101940=CARTESIAN_POINT('Ctrl Pts',(-6.88245059777448,636.073226521136,
50.1335953878553));
#101941=CARTESIAN_POINT('Ctrl Pts',(-5.87736007948177,635.872567289871,
49.7825065974709));
#101942=CARTESIAN_POINT('Ctrl Pts',(-5.9437815426704,635.804781945381,49.7114424968018));
#101943=CARTESIAN_POINT('Ctrl Pts',(-5.97236940852386,635.691672509095,
49.7234080275098));
#101944=CARTESIAN_POINT('Ctrl Pts',(-4.43240690450128,635.383525832075,
49.2925569652473));
#101945=CARTESIAN_POINT('Ctrl Pts',(-4.47704379275697,635.313078576597,
49.2235345335549));
#101946=CARTESIAN_POINT('Ctrl Pts',(-4.50406198106327,635.208454481341,
49.2314609330919));
#101947=CARTESIAN_POINT('Ctrl Pts',(-3.93312549027658,635.236185446456,
49.1503705419181));
#101948=CARTESIAN_POINT('Ctrl Pts',(-3.97216443006433,635.165338459273,
49.0822732722215));
#101949=CARTESIAN_POINT('Ctrl Pts',(-3.99670954179863,635.062868366633,
49.088694597554));
#101950=CARTESIAN_POINT('Ctrl Pts',(-2.80721571948024,634.962333725774,
48.8913556172268));
#101951=CARTESIAN_POINT('Ctrl Pts',(-2.83595961882426,634.891619931837,
48.8258047037574));
#101952=CARTESIAN_POINT('Ctrl Pts',(-2.85259747105698,634.79227663453,48.828622663863));
#101953=CARTESIAN_POINT('Ctrl Pts',(-2.17289772786691,634.846757938817,
48.7861606117588));
#101954=CARTESIAN_POINT('Ctrl Pts',(-2.19436435124887,634.775581535024,
48.7211342965425));
#101955=CARTESIAN_POINT('Ctrl Pts',(-2.20802541255103,634.678077030975,
48.7229986861513));
#101956=CARTESIAN_POINT('Ctrl Pts',(-1.52385975751051,634.77491121819,48.7210323974546));
#101957=CARTESIAN_POINT('Ctrl Pts',(-1.53802701951984,634.703667729437,
48.6565547220431));
#101958=CARTESIAN_POINT('Ctrl Pts',(-1.54849576756905,634.607085709312,
48.6576047836707));
#101959=CARTESIAN_POINT('',(-1.8888840075986,634.820085762158,48.7620619651123));
#101960=CARTESIAN_POINT('',(1.86306288877797,634.816577773823,79.840079036097));
#101961=CARTESIAN_POINT('Ctrl Pts',(-1.88888400759861,634.820085762158,
48.7620619651124));
#101962=CARTESIAN_POINT('Ctrl Pts',(-2.41149695900854,634.891566330598,
48.8271353535257));
#101963=CARTESIAN_POINT('Ctrl Pts',(-2.92444502661294,634.990847088073,
48.9183242031726));
#101964=CARTESIAN_POINT('Ctrl Pts',(-3.42867105811381,635.113486538694,
49.0343192413469));
#101965=CARTESIAN_POINT('Ctrl Pts',(-3.43116315307004,635.114092673914,
49.0348925371141));
#101966=CARTESIAN_POINT('Ctrl Pts',(-3.43365511556905,635.114699409002,
49.0354664692822));
#101967=CARTESIAN_POINT('Ctrl Pts',(-3.43614694410229,635.115306742866,
49.0360410372357));
#101968=CARTESIAN_POINT('Ctrl Pts',(-3.82123395661622,635.209164076938,
49.1248347298047));
#101969=CARTESIAN_POINT('Ctrl Pts',(-4.20323008313647,635.317350603336,
49.2288408125806));
#101970=CARTESIAN_POINT('Ctrl Pts',(-4.57646776363458,635.435822811474,
49.3457763157678));
#101971=CARTESIAN_POINT('Ctrl Pts',(-4.68985979690286,635.471815438341,
49.3813020816818));
#101972=CARTESIAN_POINT('Ctrl Pts',(-4.80244368066391,635.508757271302,
49.4180209911173));
#101973=CARTESIAN_POINT('Ctrl Pts',(-4.91406129959471,635.546534671639,
49.4558685205457));
#101974=CARTESIAN_POINT('Ctrl Pts',(-4.91843568064348,635.548015197256,
49.4573517945759));
#101975=CARTESIAN_POINT('Ctrl Pts',(-4.92280863589928,635.549496953263,
49.4588367478035));
#101976=CARTESIAN_POINT('Ctrl Pts',(-4.92718016685644,635.550979936383,
49.4603233795273));
#101977=CARTESIAN_POINT('Ctrl Pts',(-5.42040916316384,635.718301243964,
49.6280563500103));
#101978=CARTESIAN_POINT('Ctrl Pts',(-5.89557048320261,635.901250262189,
49.8171650183551));
#101979=CARTESIAN_POINT('Ctrl Pts',(-6.35515504461554,636.095269123651,
50.026781157682));
#101980=CARTESIAN_POINT('Ctrl Pts',(-6.78955134192294,636.278654472296,
50.2249089505294));
#101981=CARTESIAN_POINT('Ctrl Pts',(-7.21003104621884,636.471930271108,
50.4413581652769));
#101982=CARTESIAN_POINT('Ctrl Pts',(-7.61867416252441,636.671279341153,
50.6754123677936));
#101983=CARTESIAN_POINT('Ctrl Pts',(-7.62456670988115,636.674153912604,
50.6787873799187));
#101984=CARTESIAN_POINT('Ctrl Pts',(-7.63045674519379,636.677029804123,
50.682166103682));
#101985=CARTESIAN_POINT('Ctrl Pts',(-7.63634427132602,636.679907007694,
50.6855485406359));
#101986=CARTESIAN_POINT('Ctrl Pts',(-8.05314726616503,636.883596475645,
50.9250056267778));
#101987=CARTESIAN_POINT('Ctrl Pts',(-8.45740792076498,637.093874893464,
51.1830917656922));
#101988=CARTESIAN_POINT('Ctrl Pts',(-8.85002243750459,637.30784159817,51.4602736948679));
#101989=CARTESIAN_POINT('Ctrl Pts',(-8.85593145106618,637.311061887044,
51.4644453994501));
#101990=CARTESIAN_POINT('Ctrl Pts',(-8.8618380665553,637.314283170744,51.4686216821428));
#101991=CARTESIAN_POINT('Ctrl Pts',(-8.86774226136733,637.317505426203,
51.4728025248131));
#101992=CARTESIAN_POINT('Ctrl Pts',(-9.23018926555088,637.515313404269,
51.7294563021797));
#101993=CARTESIAN_POINT('Ctrl Pts',(-9.583630223236,637.716848985045,52.0033825468534));
#101994=CARTESIAN_POINT('Ctrl Pts',(-9.92280720324511,637.916778287441,
52.2903964742841));
#101995=CARTESIAN_POINT('Ctrl Pts',(-9.95073667622084,637.933241433166,
52.314030589222));
#101996=CARTESIAN_POINT('Ctrl Pts',(-9.9785694564295,637.949693699854,52.3377534407296));
#101997=CARTESIAN_POINT('Ctrl Pts',(-10.0063026234585,637.966132117163,
52.3615626894152));
#101998=CARTESIAN_POINT('Ctrl Pts',(-10.0117904989738,637.969384972769,
52.3662740948152));
#101999=CARTESIAN_POINT('Ctrl Pts',(-10.0172748471287,637.972637449793,
52.3709890470134));
#102000=CARTESIAN_POINT('Ctrl Pts',(-10.0227556688065,637.975889541223,
52.375707548496));
#102001=CARTESIAN_POINT('Ctrl Pts',(-10.4844704327222,638.249851862,52.7732030201896));
#102002=CARTESIAN_POINT('Ctrl Pts',(-10.9212653120677,638.521129177495,
53.1959678507371));
#102003=CARTESIAN_POINT('Ctrl Pts',(-11.3338346748915,638.785642501227,
53.64564722763));
#102004=CARTESIAN_POINT('Ctrl Pts',(-11.5776710654221,638.941974938673,
53.9114163468082));
#102005=CARTESIAN_POINT('Ctrl Pts',(-11.8130457210345,639.095945236935,
54.1865861676));
#102006=CARTESIAN_POINT('Ctrl Pts',(-12.0401046610149,639.246716958051,
54.4714903191273));
#102007=CARTESIAN_POINT('Ctrl Pts',(-12.0438323006949,639.24919218607,54.476167606973));
#102008=CARTESIAN_POINT('Ctrl Pts',(-12.0475578528826,639.251666684543,
54.4808478324097));
#102009=CARTESIAN_POINT('Ctrl Pts',(-12.0512813078029,639.25414044383,54.4855309851298));
#102010=CARTESIAN_POINT('Ctrl Pts',(-12.3319606432928,639.440615942412,
54.8385537077483));
#102011=CARTESIAN_POINT('Ctrl Pts',(-12.6007933235743,639.622941327494,
55.2083103083306));
#102012=CARTESIAN_POINT('Ctrl Pts',(-12.853551064915,639.796961270491,55.5903491046588));
#102013=CARTESIAN_POINT('Ctrl Pts',(-12.8747668389634,639.811568015159,
55.622416366922));
#102014=CARTESIAN_POINT('Ctrl Pts',(-12.8958693834308,639.826116261523,
55.654570159216));
#102015=CARTESIAN_POINT('Ctrl Pts',(-12.9168562126465,639.840603562471,
55.6868078477632));
#102016=CARTESIAN_POINT('Ctrl Pts',(-12.9194398545994,639.842387061928,
55.6907765580309));
#102017=CARTESIAN_POINT('Ctrl Pts',(-12.922021743077,639.844169633993,55.6947464964152));
#102018=CARTESIAN_POINT('Ctrl Pts',(-12.9246018778219,639.845951277251,
55.6987176634258));
#102019=CARTESIAN_POINT('Ctrl Pts',(-13.1962036721651,640.033498655008,
56.1167485774522));
#102020=CARTESIAN_POINT('Ctrl Pts',(-13.4484034732778,640.210775408409,
56.5484436861926));
#102021=CARTESIAN_POINT('Ctrl Pts',(-13.680948979807,640.376176280427,56.9945145943681));
#102022=CARTESIAN_POINT('Ctrl Pts',(-13.6823423951751,640.377167364368,
56.9971874564156));
#102023=CARTESIAN_POINT('Ctrl Pts',(-13.6837351051094,640.378158022426,
56.9998608343006));
#102024=CARTESIAN_POINT('Ctrl Pts',(-13.6851271093879,640.379148254207,
57.0025347282827));
#102025=CARTESIAN_POINT('Ctrl Pts',(-13.9184371521736,640.545118303866,
57.4506988101028));
#102026=CARTESIAN_POINT('Ctrl Pts',(-14.1319267819666,640.699113596555,
57.9133662944617));
#102027=CARTESIAN_POINT('Ctrl Pts',(-14.3245484115035,640.839268025387,
58.3917316078811));
#102028=CARTESIAN_POINT('Ctrl Pts',(-14.3248720257519,640.839503492038,
58.3925352862205));
#102029=CARTESIAN_POINT('Ctrl Pts',(-14.3251955816966,640.839738920106,
58.3933390138011));
#102030=CARTESIAN_POINT('Ctrl Pts',(-14.3255190793133,640.839974309567,
58.3941427905653));
#102031=CARTESIAN_POINT('Ctrl Pts',(-14.5183947849969,640.980318182788,
58.8733704651745));
#102032=CARTESIAN_POINT('Ctrl Pts',(-14.6905438911395,641.106943614794,
59.370094559378));
#102033=CARTESIAN_POINT('Ctrl Pts',(-14.8368369280143,641.215178668622,
59.8722326143598));
#102034=CARTESIAN_POINT('Ctrl Pts',(-14.8373300871407,641.215543532909,
59.8739253399318));
#102035=CARTESIAN_POINT('Ctrl Pts',(-14.8378229525661,641.215908188285,
59.8756181274374));
#102036=CARTESIAN_POINT('Ctrl Pts',(-14.8383155240927,641.21627263457,59.8773109764116));
#102037=CARTESIAN_POINT('Ctrl Pts',(-15.0414396045849,641.366561095379,
60.575399218893));
#102038=CARTESIAN_POINT('Ctrl Pts',(-15.1973006597185,641.483141535664,
61.2886164427717));
#102039=CARTESIAN_POINT('Ctrl Pts',(-15.3033244731206,641.562742156357,
62.0179657600747));
#102040=CARTESIAN_POINT('Ctrl Pts',(-15.3495814982321,641.597471032749,
62.3361728552828));
#102041=CARTESIAN_POINT('Ctrl Pts',(-15.3863525773576,641.625161282438,
62.6574505114078));
#102042=CARTESIAN_POINT('Ctrl Pts',(-15.4134262294948,641.64554320332,62.9818812830931));
#102043=CARTESIAN_POINT('Ctrl Pts',(-15.4140928759569,641.646045076336,
62.989869884891));
#102044=CARTESIAN_POINT('Ctrl Pts',(-15.4147536449624,641.646542521192,
62.997860444859));
#102045=CARTESIAN_POINT('Ctrl Pts',(-15.4154085331436,641.647035533691,
63.0058529638405));
#102046=CARTESIAN_POINT('Ctrl Pts',(-15.4549862599015,641.676830412449,
63.4888754727554));
#102047=CARTESIAN_POINT('Ctrl Pts',(-15.4721900515041,641.689815398436,
63.9727246693793));
#102048=CARTESIAN_POINT('Ctrl Pts',(-15.4675657250194,641.68633387532,64.4526573526707));
#102049=CARTESIAN_POINT('Ctrl Pts',(-15.4671428394911,641.686015496904,
64.4965462491376));
#102050=CARTESIAN_POINT('Ctrl Pts',(-15.4665374395128,641.685559434798,
64.5404023977485));
#102051=CARTESIAN_POINT('Ctrl Pts',(-15.465749959502,641.684965964447,64.5842221752744));
#102052=CARTESIAN_POINT('Ctrl Pts',(-15.4655480571059,641.684813804285,
64.5954571500793));
#102053=CARTESIAN_POINT('Ctrl Pts',(-15.4653341842431,641.68465260963,64.6066898685709));
#102054=CARTESIAN_POINT('Ctrl Pts',(-15.4651083473515,641.684482384512,
64.6179202686375));
#102055=CARTESIAN_POINT('Ctrl Pts',(-15.4565102683661,641.678001561122,
65.0454848978451));
#102056=CARTESIAN_POINT('Ctrl Pts',(-15.4306782059191,641.658513233691,
65.4710177591547));
#102057=CARTESIAN_POINT('Ctrl Pts',(-15.3878202693293,641.62627564013,65.8944225395906));
#102058=CARTESIAN_POINT('Ctrl Pts',(-15.3786070250346,641.619345469231,
65.9854425930057));
#102059=CARTESIAN_POINT('Ctrl Pts',(-15.368607118984,641.611826233534,66.076364320098));
#102060=CARTESIAN_POINT('Ctrl Pts',(-15.3578228674146,641.603720685738,
66.1671867939494));
#102061=CARTESIAN_POINT('Ctrl Pts',(-15.3561295795732,641.602447994218,
66.1814472727328));
#102062=CARTESIAN_POINT('Ctrl Pts',(-15.3544169428895,641.601160842789,
66.1957053639419));
#102063=CARTESIAN_POINT('Ctrl Pts',(-15.3526849656753,641.599859241441,
66.209961068781));
#102064=CARTESIAN_POINT('Ctrl Pts',(-15.2907263898706,641.553296639394,
66.7199349654947));
#102065=CARTESIAN_POINT('Ctrl Pts',(-15.2040176992693,641.488239457045,
67.2268545417177));
#102066=CARTESIAN_POINT('Ctrl Pts',(-15.0921759771049,641.404839911851,
67.7306968564118));
#102067=CARTESIAN_POINT('Ctrl Pts',(-15.0883779410082,641.402007744419,
67.7478068513332));
#102068=CARTESIAN_POINT('Ctrl Pts',(-15.0845508622971,641.399154385515,
67.7649135318261));
#102069=CARTESIAN_POINT('Ctrl Pts',(-15.0806947254962,641.396279841134,
67.7820168863499));
#102070=CARTESIAN_POINT('Ctrl Pts',(-14.9906512622138,641.329157240253,
68.181392052377));
#102071=CARTESIAN_POINT('Ctrl Pts',(-14.8857494406163,641.251224978338,
68.5741722445334));
#102072=CARTESIAN_POINT('Ctrl Pts',(-14.7673626317222,641.163831168564,
68.9585381211271));
#102073=CARTESIAN_POINT('Ctrl Pts',(-14.7373499494998,641.14167563734,69.0559801505146));
#102074=CARTESIAN_POINT('Ctrl Pts',(-14.7064707999412,641.118912168443,
69.1528814797826));
#102075=CARTESIAN_POINT('Ctrl Pts',(-14.6747479525069,641.095563010779,
69.249212655916));
#102076=CARTESIAN_POINT('Ctrl Pts',(-14.6685113493146,641.090972646326,
69.2681510353233));
#102077=CARTESIAN_POINT('Ctrl Pts',(-14.6622419924248,641.086359534144,
69.2870678366535));
#102078=CARTESIAN_POINT('Ctrl Pts',(-14.6559400474473,641.081723837857,
69.3059628438942));
#102079=CARTESIAN_POINT('Ctrl Pts',(-14.4881365257321,640.958287951733,
69.8090850972834));
#102080=CARTESIAN_POINT('Ctrl Pts',(-14.2970453980756,640.818610280766,
70.2985271980189));
#102081=CARTESIAN_POINT('Ctrl Pts',(-14.0832076583259,640.664300850609,
70.774854665362));
#102082=CARTESIAN_POINT('Ctrl Pts',(-13.8873140841637,640.522940275832,
71.2112111764187));
#102083=CARTESIAN_POINT('Ctrl Pts',(-13.6723317916547,640.369301179495,
71.6365621257869));
#102084=CARTESIAN_POINT('Ctrl Pts',(-13.4387032223677,640.204642972739,
72.0513594656846));
#102085=CARTESIAN_POINT('Ctrl Pts',(-13.4269732670318,640.196375861329,
72.0721854900244));
#102086=CARTESIAN_POINT('Ctrl Pts',(-13.4151954394702,640.1880804198,72.0929863162258));
#102087=CARTESIAN_POINT('Ctrl Pts',(-13.4033698516022,640.179756844939,
72.1137618746436));
#102088=CARTESIAN_POINT('Ctrl Pts',(-13.2658603218293,640.082969194474,
72.3553428683921));
#102089=CARTESIAN_POINT('Ctrl Pts',(-13.1230592827466,639.983202596528,
72.5914514645084));
#102090=CARTESIAN_POINT('Ctrl Pts',(-12.9752216473832,639.880887422958,
72.8220741360128));
#102091=CARTESIAN_POINT('Ctrl Pts',(-12.865760869058,639.805132027481,72.9928299591849));
#102092=CARTESIAN_POINT('Ctrl Pts',(-12.7535396983477,639.727979956785,
73.1605791986305));
#102093=CARTESIAN_POINT('Ctrl Pts',(-12.6386729408158,639.649611717406,
73.3253295048863));
#102094=CARTESIAN_POINT('Ctrl Pts',(-12.4290296027194,639.506581830803,
73.6260153159772));
#102095=CARTESIAN_POINT('Ctrl Pts',(-12.2103932271219,639.359385521563,
73.9169651027286));
#102096=CARTESIAN_POINT('Ctrl Pts',(-11.9829905176729,639.208818948779,
74.1987899103335));
#102097=CARTESIAN_POINT('Ctrl Pts',(-11.903042823286,639.155884441644,74.2978707156751));
#102098=CARTESIAN_POINT('Ctrl Pts',(-11.8220112795529,639.102533255166,
74.3958233320781));
#102099=CARTESIAN_POINT('Ctrl Pts',(-11.7399047075142,639.048799693591,
74.4926732578092));
#102100=CARTESIAN_POINT('Ctrl Pts',(-11.723313317863,639.03794167778,74.512243857526));
#102101=CARTESIAN_POINT('Ctrl Pts',(-11.7066783200462,639.027068339378,
74.5317689045803));
#102102=CARTESIAN_POINT('Ctrl Pts',(-11.6899998492774,639.016179995548,
74.5512485570587));
#102103=CARTESIAN_POINT('Ctrl Pts',(-11.3893716288856,638.81991839135,74.9023678736655));
#102104=CARTESIAN_POINT('Ctrl Pts',(-11.0743064696377,638.618628706434,
75.2388277121095));
#102105=CARTESIAN_POINT('Ctrl Pts',(-10.7444640677327,638.414001617194,
75.5611408646034));
#102106=CARTESIAN_POINT('Ctrl Pts',(-10.7256680559147,638.402340978157,
75.5795078234553));
#102107=CARTESIAN_POINT('Ctrl Pts',(-10.706824102173,638.390669575054,75.5978287367273));
#102108=CARTESIAN_POINT('Ctrl Pts',(-10.687932101418,638.378987704478,75.6161037296601));
#102109=CARTESIAN_POINT('Ctrl Pts',(-10.3916439046371,638.195777868049,
75.9027152311344));
#102110=CARTESIAN_POINT('Ctrl Pts',(-10.0822730961469,638.009261624385,
76.1790010610358));
#102111=CARTESIAN_POINT('Ctrl Pts',(-9.76302160114976,637.823091051173,
76.4419445962466));
#102112=CARTESIAN_POINT('Ctrl Pts',(-9.72558983048289,637.801262823865,
76.472774341017));
#102113=CARTESIAN_POINT('Ctrl Pts',(-9.68802222038585,637.779439370458,
76.5034206111878));
#102114=CARTESIAN_POINT('Ctrl Pts',(-9.65032392871187,637.757626598003,
76.5338784979796));
#102115=CARTESIAN_POINT('Ctrl Pts',(-9.62962043291992,637.745647258285,
76.5506056413865));
#102116=CARTESIAN_POINT('Ctrl Pts',(-9.60887807747271,637.733671422695,
76.5672755719518));
#102117=CARTESIAN_POINT('Ctrl Pts',(-9.58809774349925,637.721700079099,
76.5838874705586));
#102118=CARTESIAN_POINT('Ctrl Pts',(-9.17209645664792,637.482045877798,
76.916440893729));
#102119=CARTESIAN_POINT('Ctrl Pts',(-8.7416773191496,637.244251929722,77.2259224192763));
#102120=CARTESIAN_POINT('Ctrl Pts',(-8.29525516687926,637.012110800027,
77.5129331902512));
#102121=CARTESIAN_POINT('Ctrl Pts',(-7.94596840718463,636.830480424898,
77.7374943185049));
#102122=CARTESIAN_POINT('Ctrl Pts',(-7.58688458986681,636.652310747268,
77.9482988748328));
#102123=CARTESIAN_POINT('Ctrl Pts',(-7.21723077844875,636.479431177125,
78.1456225473662));
#102124=CARTESIAN_POINT('Ctrl Pts',(-7.19435330607693,636.468731848544,
78.15783469486));
#102125=CARTESIAN_POINT('Ctrl Pts',(-7.17143531739337,636.458052904697,
78.1699950695052));
#102126=CARTESIAN_POINT('Ctrl Pts',(-7.14847664362299,636.447394775834,
78.182103743129));
#102127=CARTESIAN_POINT('Ctrl Pts',(-6.75967649899132,636.266901682683,
78.3871614961733));
#102128=CARTESIAN_POINT('Ctrl Pts',(-6.35908010376408,636.09247477315,78.5772453815688));
#102129=CARTESIAN_POINT('Ctrl Pts',(-5.94486173776335,635.927125347824,
78.7517442446595));
#102130=CARTESIAN_POINT('Ctrl Pts',(-5.9207510096408,635.917500726208,78.7619014346612));
#102131=CARTESIAN_POINT('Ctrl Pts',(-5.8965941154069,635.907906865483,78.7720058152168));
#102132=CARTESIAN_POINT('Ctrl Pts',(-5.87239069016908,635.898344361496,
78.7820572638862));
#102133=CARTESIAN_POINT('Ctrl Pts',(-5.8489383682211,635.889078610061,78.7917967866158));
#102134=CARTESIAN_POINT('Ctrl Pts',(-5.82544172188548,635.879842124891,
78.8014867950871));
#102135=CARTESIAN_POINT('Ctrl Pts',(-5.80190050955843,635.870635502112,
78.8111271194743));
#102136=CARTESIAN_POINT('Ctrl Pts',(-5.52092170777908,635.76074881485,78.9261903013297));
#102137=CARTESIAN_POINT('Ctrl Pts',(-5.23391572238355,635.655356125412,
79.033905907466));
#102138=CARTESIAN_POINT('Ctrl Pts',(-4.94271167504838,635.5562789377,79.1333013998953));
#102139=CARTESIAN_POINT('Ctrl Pts',(-4.77501441593533,635.499222818557,
79.1905408229085));
#102140=CARTESIAN_POINT('Ctrl Pts',(-4.60592561275295,635.444260856133,
79.2450216198842));
#102141=CARTESIAN_POINT('Ctrl Pts',(-4.43579829675245,635.391736888662,
79.296563818299));
#102142=CARTESIAN_POINT('Ctrl Pts',(-4.41274763656986,635.384620382307,
79.3035473041298));
#102143=CARTESIAN_POINT('Ctrl Pts',(-4.38967592729238,635.377547954362,
79.3104775101188));
#102144=CARTESIAN_POINT('Ctrl Pts',(-4.3665840167845,635.370520469936,79.3173539744283));
#102145=CARTESIAN_POINT('Ctrl Pts',(-4.04882336542099,635.273817426323,
79.4119788768291));
#102146=CARTESIAN_POINT('Ctrl Pts',(-3.72622839310077,635.185213899862,
79.4968684248799));
#102147=CARTESIAN_POINT('Ctrl Pts',(-3.39848998472152,635.106166302133,
79.5715572830165));
#102148=CARTESIAN_POINT('Ctrl Pts',(-3.24344222812536,635.0687701582,79.6068913775282));
#102149=CARTESIAN_POINT('Ctrl Pts',(-3.0872435683127,635.033512344151,79.639943018132));
#102150=CARTESIAN_POINT('Ctrl Pts',(-2.92986272136949,635.000544637532,
79.6706660016241));
#102151=CARTESIAN_POINT('Ctrl Pts',(-2.90796583102349,634.995957737215,
79.6749405865796));
#102152=CARTESIAN_POINT('Ctrl Pts',(-2.88604686704024,634.991415266355,
79.6791700030138));
#102153=CARTESIAN_POINT('Ctrl Pts',(-2.86410536448456,634.986917552588,
79.6833542027662));
#102154=CARTESIAN_POINT('Ctrl Pts',(-2.67077137140562,634.947286676806,
79.7202226006317));
#102155=CARTESIAN_POINT('Ctrl Pts',(-2.47523365109657,634.911146502476,
79.7535703438631));
#102156=CARTESIAN_POINT('Ctrl Pts',(-2.27824761487356,634.878810798285,
79.783236645037));
#102157=CARTESIAN_POINT('Ctrl Pts',(-2.09244054752051,634.848310147165,
79.8112193819154));
#102158=CARTESIAN_POINT('Ctrl Pts',(-1.90534362430371,634.821194294132,
79.8359266171042));
#102159=CARTESIAN_POINT('Ctrl Pts',(-1.71759256272266,634.79775958441,79.8571931173366));
#102160=CARTESIAN_POINT('Ctrl Pts',(-1.59648021958737,634.782642585437,
79.8709114721185));
#102161=CARTESIAN_POINT('Ctrl Pts',(-1.47509576549149,634.769058026899,
79.8831974849578));
#102162=CARTESIAN_POINT('Ctrl Pts',(-1.35361376683639,634.757093789453,
79.8939995839849));
#102163=CARTESIAN_POINT('Ctrl Pts',(-1.33479741520131,634.755240648236,
79.8956727215356));
#102164=CARTESIAN_POINT('Ctrl Pts',(-1.31597645205385,634.753425996979,
79.8973106052341));
#102165=CARTESIAN_POINT('Ctrl Pts',(-1.29715200364572,634.751650247623,
79.8989129667661));
#102166=CARTESIAN_POINT('Ctrl Pts',(-1.11523121238339,634.734489281146,
79.9143983011279));
#102167=CARTESIAN_POINT('Ctrl Pts',(-0.932588982074347,634.720883278272,
79.9267009011113));
#102168=CARTESIAN_POINT('Ctrl Pts',(-0.749467854780609,634.710917091553,
79.9357300191259));
#102169=CARTESIAN_POINT('Ctrl Pts',(-0.68360717759574,634.707332689164,
79.9389773988008));
#102170=CARTESIAN_POINT('Ctrl Pts',(-0.617684568112042,634.704218742184,
79.9418016685007));
#102171=CARTESIAN_POINT('Ctrl Pts',(-0.551711358599846,634.701577963951,
79.9441997051945));
#102172=CARTESIAN_POINT('Ctrl Pts',(-0.345342966588289,634.693317441815,
79.9517009163701));
#102173=CARTESIAN_POINT('Ctrl Pts',(-0.13842335344143,634.689669307663,
79.9550471976343));
#102174=CARTESIAN_POINT('Ctrl Pts',(0.0688418019382751,634.69072047944,
79.9541394471176));
#102175=CARTESIAN_POINT('Ctrl Pts',(0.131131170306721,634.691036387948,
79.9538666409809));
#102176=CARTESIAN_POINT('Ctrl Pts',(0.193451665010501,634.69177647057,79.9532098508914));
#102177=CARTESIAN_POINT('Ctrl Pts',(0.255797490386204,634.692942419917,
79.9521669823772));
#102178=CARTESIAN_POINT('Ctrl Pts',(0.666136199024486,634.700616296175,
79.9453031816842));
#102179=CARTESIAN_POINT('Ctrl Pts',(1.07421972569375,634.726606258343,79.9218319778895));
#102180=CARTESIAN_POINT('Ctrl Pts',(1.48012296303281,634.770182961628,79.8822570048232));
#102181=CARTESIAN_POINT('Ctrl Pts',(1.6079847342995,634.783909864879,79.8697906687889));
#102182=CARTESIAN_POINT('Ctrl Pts',(1.73563038656575,634.799382147975,79.8557262296273));
#102183=CARTESIAN_POINT('Ctrl Pts',(1.86306288877797,634.816577773823,79.840079036097));
#102184=CARTESIAN_POINT('',(-1.91941230150446,634.6517886719,48.698800681464));
#102185=CARTESIAN_POINT('Origin',(-1.88888400761935,634.651788671899,48.9469297270682));
#102186=CARTESIAN_POINT('',(1.49247666926852E-9,634.523620405604,80.0178253754844));
#102187=CARTESIAN_POINT('Ctrl Pts',(0.,634.523561041887,80.0177804323122));
#102188=CARTESIAN_POINT('Ctrl Pts',(-0.523838402099614,634.523561041886,
80.0177804323122));
#102189=CARTESIAN_POINT('Ctrl Pts',(-1.04370866617181,634.552420716909,
79.9916639229812));
#102190=CARTESIAN_POINT('Ctrl Pts',(-2.07588373512256,634.664326010256,
79.8887286024128));
#102191=CARTESIAN_POINT('Ctrl Pts',(-2.58884491618879,634.747802856386,
79.8114551737427));
#102192=CARTESIAN_POINT('Ctrl Pts',(-3.58593453053115,634.958082826433,
79.6117158816492));
#102193=CARTESIAN_POINT('Ctrl Pts',(-4.0730770151066,635.085061620392,79.4890655970438));
#102194=CARTESIAN_POINT('Ctrl Pts',(-5.02736864376844,635.373997049357,
79.2004542940851));
#102195=CARTESIAN_POINT('Ctrl Pts',(-5.49684127598253,635.536898097831,
79.0334559601684));
#102196=CARTESIAN_POINT('Ctrl Pts',(-6.85808462896243,636.058637569066,
78.4766795782573));
#102197=CARTESIAN_POINT('Ctrl Pts',(-7.70355359238228,636.448549836785,
78.0333468553696));
#102198=CARTESIAN_POINT('Ctrl Pts',(-8.89973254356871,637.057230951149,
77.2642195998673));
#102199=CARTESIAN_POINT('Ctrl Pts',(-9.28623993692406,637.264306410741,
76.9902938266832));
#102200=CARTESIAN_POINT('Ctrl Pts',(-10.0362291980326,637.68204941874,76.4058881437883));
#102201=CARTESIAN_POINT('Ctrl Pts',(-10.4000435824971,637.892995650452,
76.0948005375614));
#102202=CARTESIAN_POINT('Ctrl Pts',(-11.4396209671232,638.513918977268,
75.1208482803277));
#102203=CARTESIAN_POINT('Ctrl Pts',(-12.0708675035256,638.915587641525,
74.4129443846916));
#102204=CARTESIAN_POINT('Ctrl Pts',(-12.9272407039081,639.478792555837,
73.2539335615611));
#102205=CARTESIAN_POINT('Ctrl Pts',(-13.1974645163444,639.660006071349,
72.8512918153461));
#102206=CARTESIAN_POINT('Ctrl Pts',(-13.705907162251,640.005749387722,72.0101656887144));
#102207=CARTESIAN_POINT('Ctrl Pts',(-13.9424367491172,640.169145509004,
71.5740025956755));
#102208=CARTESIAN_POINT('Ctrl Pts',(-14.5877396657579,640.61954466326,70.2361076880824));
#102209=CARTESIAN_POINT('Ctrl Pts',(-14.9374786600809,640.870144794768,
69.2981314957323));
#102210=CARTESIAN_POINT('Ctrl Pts',(-15.2640367599687,641.105956087144,
68.0597854794833));
#102211=CARTESIAN_POINT('Ctrl Pts',(-15.3238781708752,641.149308553529,
67.8080648198323));
#102212=CARTESIAN_POINT('Ctrl Pts',(-15.4305740793169,641.22676859308,67.3042760285323));
#102213=CARTESIAN_POINT('Ctrl Pts',(-15.4776212824142,641.26101472037,67.0516154405275));
#102214=CARTESIAN_POINT('Ctrl Pts',(-15.6000369014761,641.350256255448,
66.2913465819385));
#102215=CARTESIAN_POINT('Ctrl Pts',(-15.6567243462522,641.391772923005,
65.7814558786312));
#102216=CARTESIAN_POINT('Ctrl Pts',(-15.7200921410461,641.438194610325,
64.7555336881403));
#102217=CARTESIAN_POINT('Ctrl Pts',(-15.7267764511932,641.443102869943,
64.2395027071171));
#102218=CARTESIAN_POINT('Ctrl Pts',(-15.6884879697056,641.41503836218,63.2010937639321));
#102219=CARTESIAN_POINT('Ctrl Pts',(-15.6429785458214,641.381673100163,
62.6781815568624));
#102220=CARTESIAN_POINT('Ctrl Pts',(-15.4329805623442,641.228341491889,
61.1446179884831));
#102221=CARTESIAN_POINT('Ctrl Pts',(-15.1957463219534,641.055416837413,
60.1535682172885));
#102222=CARTESIAN_POINT('Ctrl Pts',(-14.7000874693409,640.701185096577,
58.7109944575794));
#102223=CARTESIAN_POINT('Ctrl Pts',(-14.5127468230508,640.568220140849,
58.242003763886));
#102224=CARTESIAN_POINT('Ctrl Pts',(-14.1005377299408,640.279018469053,
57.3361700731209));
#102225=CARTESIAN_POINT('Ctrl Pts',(-13.8750752636248,640.122351198019,
56.8975962595972));
#102226=CARTESIAN_POINT('Ctrl Pts',(-13.1426912261625,639.620891692776,
55.6221334704683));
#102227=CARTESIAN_POINT('Ctrl Pts',(-12.5757171471258,639.241825375141,
54.8214953487566));
#102228=CARTESIAN_POINT('Ctrl Pts',(-11.3331559325469,638.450142176263,
53.3660245246631));
#102229=CARTESIAN_POINT('Ctrl Pts',(-10.6547752361309,638.035107392668,
52.7042730339687));
#102230=CARTESIAN_POINT('Ctrl Pts',(-9.54585906942516,637.406533531398,
51.8027276685537));
#102231=CARTESIAN_POINT('Ctrl Pts',(-9.16098839272779,637.196240615232,
51.5179512580578));
#102232=CARTESIAN_POINT('Ctrl Pts',(-8.37201911995265,636.785698604155,
50.9878126575492));
#102233=CARTESIAN_POINT('Ctrl Pts',(-7.96635410967427,636.58452539553,50.7411093620899));
#102234=CARTESIAN_POINT('Ctrl Pts',(-6.71291294709257,636.001439692389,
50.0548419703803));
#102235=CARTESIAN_POINT('Ctrl Pts',(-5.82961165971477,635.638936240212,
49.6681929464691));
#102236=CARTESIAN_POINT('Ctrl Pts',(-4.40836677555933,635.180500942699,
49.2037840375558));
#102237=CARTESIAN_POINT('Ctrl Pts',(-3.91938654325121,635.042911076968,
49.0692534214259));
#102238=CARTESIAN_POINT('Ctrl Pts',(-2.93166846065344,634.813010109247,
48.8486963579089));
#102239=CARTESIAN_POINT('Ctrl Pts',(-2.42992069874045,634.719685488227,
48.7616105405085));
#102240=CARTESIAN_POINT('Ctrl Pts',(-1.91941230150446,634.6517886719,48.698800681464));
#102241=CARTESIAN_POINT('',(1.89317385967765,634.648322422428,79.9033533194805));
#102242=CARTESIAN_POINT('Ctrl Pts',(1.89317385967764,634.648322422428,79.9033533194805));
#102243=CARTESIAN_POINT('Ctrl Pts',(1.58012448505219,634.607246312445,79.9413347011642));
#102244=CARTESIAN_POINT('Ctrl Pts',(1.26585353386948,634.576145886255,79.9700061023909));
#102245=CARTESIAN_POINT('Ctrl Pts',(0.950335111694906,634.555301997871,
79.9891761306859));
#102246=CARTESIAN_POINT('Ctrl Pts',(0.788177405142235,634.544589478733,
79.9990283852752));
#102247=CARTESIAN_POINT('Ctrl Pts',(0.625503300950952,634.536577108366,
80.0063792748622));
#102248=CARTESIAN_POINT('Ctrl Pts',(0.462595958332864,634.531322615861,
80.0111851918327));
#102249=CARTESIAN_POINT('Ctrl Pts',(0.308526274103216,634.526353177478,
80.0157303897235));
#102250=CARTESIAN_POINT('Ctrl Pts',(0.154247965605474,634.523850225432,
80.0179995314596));
#102251=CARTESIAN_POINT('Ctrl Pts',(6.79067047038018E-9,634.5238311429,
80.0179849207937));
#102252=CARTESIAN_POINT('Origin',(1.86306288877797,634.648322422428,79.6551732851678));
#102253=CARTESIAN_POINT('Ctrl Pts',(-0.252645464510396,637.415474030314,
76.9980210944396));
#102254=CARTESIAN_POINT('Ctrl Pts',(-0.239928764978578,637.71957350873,
76.5971361934352));
#102255=CARTESIAN_POINT('Ctrl Pts',(-0.247612686332898,637.216296403659,
76.5969814761947));
#102256=CARTESIAN_POINT('Ctrl Pts',(0.599346104179954,637.402304042614,
77.0153826803362));
#102257=CARTESIAN_POINT('Ctrl Pts',(0.570806075610007,637.708243376892,
76.6129375177081));
#102258=CARTESIAN_POINT('Ctrl Pts',(0.587407127222553,637.203283112552,
76.613794761412));
#102259=CARTESIAN_POINT('Ctrl Pts',(1.43522748368769,637.456242191975,76.9455084004709));
#102260=CARTESIAN_POINT('Ctrl Pts',(1.3489476199593,637.752521117499,76.5522413898123));
#102261=CARTESIAN_POINT('Ctrl Pts',(1.40663729476956,637.256579496553,76.5461272140149));
#102262=CARTESIAN_POINT('Ctrl Pts',(2.66678387891633,637.624714906102,76.7177190065359));
#102263=CARTESIAN_POINT('Ctrl Pts',(2.53731328870643,637.900219491323,76.3416431735781));
#102264=CARTESIAN_POINT('Ctrl Pts',(2.61366069407739,637.423047682413,76.3255317586155));
#102265=CARTESIAN_POINT('Ctrl Pts',(3.07572538189221,637.695889939016,76.6204570030234));
#102266=CARTESIAN_POINT('Ctrl Pts',(2.92857212557764,637.961901314834,76.2529152101653));
#102267=CARTESIAN_POINT('Ctrl Pts',(3.01445595206078,637.493375858542,76.2313414391483));
#102268=CARTESIAN_POINT('Ctrl Pts',(3.8755985784546,637.862370610506,76.3871426082101));
#102269=CARTESIAN_POINT('Ctrl Pts',(3.70006557576271,638.108664391703,76.0368396544836));
#102270=CARTESIAN_POINT('Ctrl Pts',(3.7983954194345,637.657875703638,76.0053954703534));
#102271=CARTESIAN_POINT('Ctrl Pts',(4.26480616625281,637.957101329594,76.2518851665813));
#102272=CARTESIAN_POINT('Ctrl Pts',(4.07641784659729,638.192281742605,75.9117507781356));
#102273=CARTESIAN_POINT('Ctrl Pts',(4.17984986817795,637.751479294978,75.874409667253));
#102274=CARTESIAN_POINT('Ctrl Pts',(5.02377713750492,638.164761246445,75.9459140475635));
#102275=CARTESIAN_POINT('Ctrl Pts',(4.81486847221986,638.378208854777,75.6252072189681));
#102276=CARTESIAN_POINT('Ctrl Pts',(4.92370189566428,637.956668425041,75.5781015854782));
#102277=CARTESIAN_POINT('Ctrl Pts',(5.39353601298289,638.277696548749,75.7751934044062));
#102278=CARTESIAN_POINT('Ctrl Pts',(5.17578544904304,638.479637284875,75.4653304964425));
#102279=CARTESIAN_POINT('Ctrl Pts',(5.28609505655054,638.068259997294,75.4127725629522));
#102280=CARTESIAN_POINT('Ctrl Pts',(6.11485814111501,638.517575135291,75.398561954746));
#102281=CARTESIAN_POINT('Ctrl Pts',(5.88314832657038,638.697574974731,75.1089592769933));
#102282=CARTESIAN_POINT('Ctrl Pts',(5.99304821798366,638.305284451723,75.0480357125633));
#102283=CARTESIAN_POINT('Ctrl Pts',(6.46756038601705,638.645018194642,75.1917528950879));
#102284=CARTESIAN_POINT('Ctrl Pts',(6.23031283838703,638.813863825324,74.9130743719703));
#102285=CARTESIAN_POINT('Ctrl Pts',(6.33872452185387,638.431211164344,74.8477580011569));
#102286=CARTESIAN_POINT('Ctrl Pts',(7.48242996358273,639.035870261262,74.5288163772505));
#102287=CARTESIAN_POINT('Ctrl Pts',(7.21704842590842,639.168144716683,74.2897410752272));
#102288=CARTESIAN_POINT('Ctrl Pts',(7.33337757366972,638.817412780853,74.2057580358069));
#102289=CARTESIAN_POINT('Ctrl Pts',(8.10709315029709,639.309087260829,74.028620906189));
#102290=CARTESIAN_POINT('Ctrl Pts',(7.84051708959433,639.422143423535,73.8120742692735));
#102291=CARTESIAN_POINT('Ctrl Pts',(7.94559727067024,639.087378981886,73.721359506763));
#102292=CARTESIAN_POINT('Ctrl Pts',(8.97315991273498,639.716567245409,73.188449545123));
#102293=CARTESIAN_POINT('Ctrl Pts',(8.71531793774959,639.809772891231,72.9883352789045));
#102294=CARTESIAN_POINT('Ctrl Pts',(8.79441170737145,639.490010673385,72.9077220474778));
#102295=CARTESIAN_POINT('Ctrl Pts',(9.25113112703224,639.852690149644,72.8917703602215));
#102296=CARTESIAN_POINT('Ctrl Pts',(8.99305377021651,639.938008123952,72.7011730151351));
#102297=CARTESIAN_POINT('Ctrl Pts',(9.06684564649771,639.624513956044,72.6204124471552));
#102298=CARTESIAN_POINT('Ctrl Pts',(9.77628595094184,640.117696108027,72.2740035948496));
#102299=CARTESIAN_POINT('Ctrl Pts',(9.51738335439514,640.188181759637,72.1016116954675));
#102300=CARTESIAN_POINT('Ctrl Pts',(9.58153921876773,639.886366811092,72.0221557047211));
#102301=CARTESIAN_POINT('Ctrl Pts',(10.0229859433045,640.246276120254,71.9538219181877));
#102302=CARTESIAN_POINT('Ctrl Pts',(9.76463235697413,640.310160688117,71.7902694724233));
#102303=CARTESIAN_POINT('Ctrl Pts',(9.82332486871901,640.013416948774,71.7120858574342));
#102304=CARTESIAN_POINT('Ctrl Pts',(10.7167107520177,640.616230378276,70.9588372302021));
#102305=CARTESIAN_POINT('Ctrl Pts',(10.4508934408169,640.657319512709,70.8323532494638));
#102306=CARTESIAN_POINT('Ctrl Pts',(10.5032304581882,640.378969403766,70.7485243138466));
#102307=CARTESIAN_POINT('Ctrl Pts',(11.1179466017888,640.841950027329,70.250007157043));
#102308=CARTESIAN_POINT('Ctrl Pts',(10.8576198832383,640.874656679083,70.138628472291));
#102309=CARTESIAN_POINT('Ctrl Pts',(10.8964735613622,640.602003388908,70.0620801831889));
#102310=CARTESIAN_POINT('Ctrl Pts',(11.6224782615555,641.132665168508,69.109586211324));
#102311=CARTESIAN_POINT('Ctrl Pts',(11.3677587268443,641.154807136228,69.014472786789));
#102312=CARTESIAN_POINT('Ctrl Pts',(11.390954790485,640.88925953228,68.957675482628));
#102313=CARTESIAN_POINT('Ctrl Pts',(11.7745701409246,641.221747318877,68.714791080186));
#102314=CARTESIAN_POINT('Ctrl Pts',(11.520855565674,641.240337307385,68.6277463485386));
#102315=CARTESIAN_POINT('Ctrl Pts',(11.5400169509314,640.977281762863,68.5753485881025));
#102316=CARTESIAN_POINT('Ctrl Pts',(12.036826018648,641.376809486983,67.9187349800865));
#102317=CARTESIAN_POINT('Ctrl Pts',(11.7840009883711,641.38886168525,67.8485756225846));
#102318=CARTESIAN_POINT('Ctrl Pts',(11.7970486078528,641.130498964837,67.804433162233));
#102319=CARTESIAN_POINT('Ctrl Pts',(12.1481605517107,641.4434586933,67.5152272280643));
#102320=CARTESIAN_POINT('Ctrl Pts',(11.8961680044815,641.453002536285,67.4527537325953));
#102321=CARTESIAN_POINT('Ctrl Pts',(11.906165321538,641.19635516356,67.4136688048127));
#102322=CARTESIAN_POINT('Ctrl Pts',(12.3313243194805,641.553729512778,66.6971148274926));
#102323=CARTESIAN_POINT('Ctrl Pts',(12.0800305729695,641.558788506436,66.6513216880366));
#102324=CARTESIAN_POINT('Ctrl Pts',(12.0856804087928,641.305313954761,66.6213936503897));
#102325=CARTESIAN_POINT('Ctrl Pts',(12.4031554959512,641.597355242453,66.2825110894363));
#102326=CARTESIAN_POINT('Ctrl Pts',(12.1524261846195,641.600829236324,66.2443008543885));
#102327=CARTESIAN_POINT('Ctrl Pts',(12.1560806850811,641.348420615636,66.2198837351635));
#102328=CARTESIAN_POINT('Ctrl Pts',(12.5061462176465,641.660056061986,65.4417759684511));
#102329=CARTESIAN_POINT('Ctrl Pts',(12.2558350970482,641.661037104903,65.4202915379704));
#102330=CARTESIAN_POINT('Ctrl Pts',(12.257019799162,641.410375405783,65.405700320617));
#102331=CARTESIAN_POINT('Ctrl Pts',(12.5373399906064,641.679151832955,65.0141778683388));
#102332=CARTESIAN_POINT('Ctrl Pts',(12.2872829443278,641.679454203773,65.0003000739761));
#102333=CARTESIAN_POINT('Ctrl Pts',(12.2875921822733,641.429243970851,64.9916064252471));
#102334=CARTESIAN_POINT('Ctrl Pts',(12.5658991754142,641.696620496606,63.7224078328247));
#102335=CARTESIAN_POINT('Ctrl Pts',(12.3159477798069,641.696227274136,63.7345453497792));
#102336=CARTESIAN_POINT('Ctrl Pts',(12.3155824582831,641.446504788682,63.7406324714832));
#102337=CARTESIAN_POINT('Ctrl Pts',(12.4989259854136,641.655343862422,62.8753544483646));
#102338=CARTESIAN_POINT('Ctrl Pts',(12.2476351021315,641.655943343438,62.8975114326958));
#102339=CARTESIAN_POINT('Ctrl Pts',(12.2499433960128,641.405719273125,62.9203303339275));
#102340=CARTESIAN_POINT('Ctrl Pts',(12.2757039450297,641.520177357917,61.6247744041512));
#102341=CARTESIAN_POINT('Ctrl Pts',(12.02433270669,641.526673421497,61.6764817660471));
#102342=CARTESIAN_POINT('Ctrl Pts',(12.0311680098947,641.272161011494,61.7092455282533));
#102343=CARTESIAN_POINT('Ctrl Pts',(12.1802763920905,641.462634802374,61.2099033326353));
#102344=CARTESIAN_POINT('Ctrl Pts',(11.9281609256542,641.471251810815,61.269319855613));
#102345=CARTESIAN_POINT('Ctrl Pts',(11.9376414045012,641.215303110347,61.3074767223547));
#102346=CARTESIAN_POINT('Ctrl Pts',(11.9490055759325,641.324698711005,60.3929349339052));
#102347=CARTESIAN_POINT('Ctrl Pts',(11.6960573690714,641.339031872542,60.4693531862596));
#102348=CARTESIAN_POINT('Ctrl Pts',(11.710977576111,641.079008215471,60.5163094405145));
#102349=CARTESIAN_POINT('Ctrl Pts',(11.8146027265403,641.245168037968,59.9953322208473));
#102350=CARTESIAN_POINT('Ctrl Pts',(11.5607302358161,641.262599583117,60.0796799798351));
#102351=CARTESIAN_POINT('Ctrl Pts',(11.5792520747703,641.000423816397,60.1312636317803));
#102352=CARTESIAN_POINT('Ctrl Pts',(11.5102203665223,641.067645854497,59.220368588735));
#102353=CARTESIAN_POINT('Ctrl Pts',(11.2554200175323,641.092765637189,59.3216529465386));
#102354=CARTESIAN_POINT('Ctrl Pts',(11.280933108072,640.825013833895,59.3807745414427));
#102355=CARTESIAN_POINT('Ctrl Pts',(11.340234579966,640.969646468321,58.8430123811434));
#102356=CARTESIAN_POINT('Ctrl Pts',(11.0844074462808,640.998826285913,58.9523736714234));
#102357=CARTESIAN_POINT('Ctrl Pts',(11.1143334927416,640.728180466839,59.0153358225178));
#102358=CARTESIAN_POINT('Ctrl Pts',(10.9653218879177,640.757511556913,58.1076875427682));
#102359=CARTESIAN_POINT('Ctrl Pts',(10.7086606118733,640.796424777516,58.2342052329224));
#102360=CARTESIAN_POINT('Ctrl Pts',(10.7468891809611,640.518569586652,58.3032336718348));
#102361=CARTESIAN_POINT('Ctrl Pts',(10.7594229698032,640.642843732934,57.748247707264));
#102362=CARTESIAN_POINT('Ctrl Pts',(10.5017718495429,640.686893603715,57.8832035358986));
#102363=CARTESIAN_POINT('Ctrl Pts',(10.5450918351581,640.405266106664,57.9551454984287));
#102364=CARTESIAN_POINT('Ctrl Pts',(10.0956130835857,640.281843896905,56.7094894932663));
#102365=CARTESIAN_POINT('Ctrl Pts',(9.82988413289725,640.339878780936,56.8595245434182));
#102366=CARTESIAN_POINT('Ctrl Pts',(9.89450525281217,640.04856153217,56.9491928643266));
#102367=CARTESIAN_POINT('Ctrl Pts',(9.5965007327143,640.020836388794,56.0745184163995));
#102368=CARTESIAN_POINT('Ctrl Pts',(9.32615145971497,640.091117978275,56.2424874391652));
#102369=CARTESIAN_POINT('Ctrl Pts',(9.40533537943261,639.790659551114,56.3342751495656));
#102370=CARTESIAN_POINT('Ctrl Pts',(8.48692376686844,639.482176762763,54.9079363581114));
#102371=CARTESIAN_POINT('Ctrl Pts',(8.21935109391615,639.584201598171,55.1122541884108));
#102372=CARTESIAN_POINT('Ctrl Pts',(8.31786154047716,639.258409024392,55.2045355438743));
#102373=CARTESIAN_POINT('Ctrl Pts',(7.87102737898878,639.202422841643,54.3737954611148));
#102374=CARTESIAN_POINT('Ctrl Pts',(7.60328278950778,639.322779690413,54.6002522073219));
#102375=CARTESIAN_POINT('Ctrl Pts',(7.71423400494031,638.98198367962,54.687263637379));
#102376=CARTESIAN_POINT('Ctrl Pts',(6.56285306515126,638.672930315504,53.4432039225965));
#102377=CARTESIAN_POINT('Ctrl Pts',(6.30828894600969,638.832969696623,53.7086110751252));
#102378=CARTESIAN_POINT('Ctrl Pts',(6.43211894031247,638.458791180624,53.786061608348));
#102379=CARTESIAN_POINT('Ctrl Pts',(5.86710297479519,638.420941785181,53.0415050222643));
#102380=CARTESIAN_POINT('Ctrl Pts',(5.62291561811055,638.604759063604,53.3322766970217));
#102381=CARTESIAN_POINT('Ctrl Pts',(5.75022841332413,638.209800867581,53.3970489773778));
#102382=CARTESIAN_POINT('Ctrl Pts',(4.75112300194525,638.086758847639,52.5364612008833));
#102383=CARTESIAN_POINT('Ctrl Pts',(4.54890972975399,638.307939687588,52.8639499834371));
#102384=CARTESIAN_POINT('Ctrl Pts',(4.65647911755443,637.87959411755,52.9079552143514));
#102385=CARTESIAN_POINT('Ctrl Pts',(4.36447646411708,637.982211773197,52.3837883044384));
#102386=CARTESIAN_POINT('Ctrl Pts',(4.17347758256706,638.214957381859,52.7219730108443));
#102387=CARTESIAN_POINT('Ctrl Pts',(4.27753470189083,637.776290968105,52.760103963041));
#102388=CARTESIAN_POINT('Ctrl Pts',(3.57968505656083,637.796737097994,52.118787442565));
#102389=CARTESIAN_POINT('Ctrl Pts',(3.41373149403426,638.050384043215,52.4753963396111));
#102390=CARTESIAN_POINT('Ctrl Pts',(3.5083765892915,637.593023114497,52.503472235072));
#102391=CARTESIAN_POINT('Ctrl Pts',(3.18116850106493,637.715539157465,52.005977374802));
#102392=CARTESIAN_POINT('Ctrl Pts',(3.0308328190885,637.979497306057,52.3719224428149));
#102393=CARTESIAN_POINT('Ctrl Pts',(3.11779861057926,637.512791285563,52.3942248829386));
#102394=CARTESIAN_POINT('Ctrl Pts',(1.96629699390316,637.512004536896,51.7270877774893));
#102395=CARTESIAN_POINT('Ctrl Pts',(1.85276789715343,637.799756796079,52.1125876973074));
#102396=CARTESIAN_POINT('Ctrl Pts',(1.92712773112881,637.311678368128,52.1241430466814));
#102397=CARTESIAN_POINT('Ctrl Pts',(1.1273257642139,637.429925082731,51.6199783226107));
#102398=CARTESIAN_POINT('Ctrl Pts',(1.06865977295132,637.731952156895,52.0190762779579));
#102399=CARTESIAN_POINT('Ctrl Pts',(1.10486896435859,637.23057551233,52.0204162706371));
#102400=CARTESIAN_POINT('Ctrl Pts',(0.270210553101147,637.415754985731,
51.6012974652903));
#102401=CARTESIAN_POINT('Ctrl Pts',(0.256610940649088,637.719814747952,
52.0021484287645));
#102402=CARTESIAN_POINT('Ctrl Pts',(0.264827872760487,637.216574016203,
52.0023253862613));
#102403=CARTESIAN_POINT('',(0.270210553101167,637.415754985731,51.6012974652903));
#102404=CARTESIAN_POINT('',(-0.252645464510396,637.415474030314,76.9980210944396));
#102405=CARTESIAN_POINT('Ctrl Pts',(0.270210553101167,637.415754985731,
51.6012974652903));
#102406=CARTESIAN_POINT('Ctrl Pts',(0.416188845712236,637.418168344564,
51.6044790675076));
#102407=CARTESIAN_POINT('Ctrl Pts',(0.562179672062563,637.422563160715,
51.6102408737133));
#102408=CARTESIAN_POINT('Ctrl Pts',(0.707836668902967,637.428891368953,
51.6185654510171));
#102409=CARTESIAN_POINT('Ctrl Pts',(0.855734314323139,637.435316924322,
51.6270180856934));
#102410=CARTESIAN_POINT('Ctrl Pts',(1.00328760572369,637.443735718904,51.6381129450356));
#102411=CARTESIAN_POINT('Ctrl Pts',(1.1501423060896,637.454064618708,51.651789297983));
#102412=CARTESIAN_POINT('Ctrl Pts',(1.28385901362555,637.463469469019,51.6642421298138));
#102413=CARTESIAN_POINT('Ctrl Pts',(1.4169965503748,637.474457442842,51.678834639128));
#102414=CARTESIAN_POINT('Ctrl Pts',(1.54929519817636,637.486943941046,51.6954914009046));
#102415=CARTESIAN_POINT('Ctrl Pts',(1.75719362309161,637.506565632971,51.7216663814889));
#102416=CARTESIAN_POINT('Ctrl Pts',(1.96334804814262,637.529911630287,51.7529703760962));
#102417=CARTESIAN_POINT('Ctrl Pts',(2.1678167060391,637.556769095995,51.7892635905837));
#102418=CARTESIAN_POINT('Ctrl Pts',(2.37228536393557,637.583626561702,51.8255568050713));
#102419=CARTESIAN_POINT('Ctrl Pts',(2.57506848853288,637.613995807679,51.8668394514028));
#102420=CARTESIAN_POINT('Ctrl Pts',(2.77621117828721,637.64769460665,51.913014617884));
#102421=CARTESIAN_POINT('Ctrl Pts',(2.780947277973,637.648488077551,51.9141018569566));
#102422=CARTESIAN_POINT('Ctrl Pts',(2.78568258013031,637.649283388912,51.9151918299073));
#102423=CARTESIAN_POINT('Ctrl Pts',(2.79041708794957,637.650080538493,51.9162845374166));
#102424=CARTESIAN_POINT('Ctrl Pts',(3.19062783311624,637.71746406392,52.0086517492298));
#102425=CARTESIAN_POINT('Ctrl Pts',(3.58441626783845,637.79786112867,52.1203933631369));
#102426=CARTESIAN_POINT('Ctrl Pts',(3.97207884850314,637.889477127378,52.2512917195333));
#102427=CARTESIAN_POINT('Ctrl Pts',(3.9785435235221,637.89100491904,52.2534745851923));
#102428=CARTESIAN_POINT('Ctrl Pts',(3.98500659612944,637.892535904034,52.2556629087786));
#102429=CARTESIAN_POINT('Ctrl Pts',(3.99146802647607,637.894070059965,52.2578566698448));
#102430=CARTESIAN_POINT('Ctrl Pts',(4.32723754954278,637.973792780423,52.371855903358));
#102431=CARTESIAN_POINT('Ctrl Pts',(4.65860664868912,638.062095960474,52.5005649822514));
#102432=CARTESIAN_POINT('Ctrl Pts',(4.97989942399088,638.155824072753,52.6410924030451));
#102433=CARTESIAN_POINT('Ctrl Pts',(5.02786800056233,638.169817553081,52.6620729568045));
#102434=CARTESIAN_POINT('Ctrl Pts',(5.07561206228213,638.183931950536,52.6833169044677));
#102435=CARTESIAN_POINT('Ctrl Pts',(5.12311282356784,638.198156764768,52.7048145891233));
#102436=CARTESIAN_POINT('Ctrl Pts',(5.13072165517588,638.200435343325,52.708258160512));
#102437=CARTESIAN_POINT('Ctrl Pts',(5.13832532939628,638.202716944462,52.7117084833211));
#102438=CARTESIAN_POINT('Ctrl Pts',(5.14592385222657,638.205001549891,52.7151655548058));
#102439=CARTESIAN_POINT('Ctrl Pts',(5.6540545374847,638.357778365596,52.9463478703353));
#102440=CARTESIAN_POINT('Ctrl Pts',(6.13932327119867,638.524027475389,53.2077731234659));
#102441=CARTESIAN_POINT('Ctrl Pts',(6.60384272768677,638.698424725211,53.4988133237996));
#102442=CARTESIAN_POINT('Ctrl Pts',(6.81232117456394,638.776695004905,53.6294334907203));
#102443=CARTESIAN_POINT('Ctrl Pts',(7.01662033272776,638.856606954161,53.7660183723263));
#102444=CARTESIAN_POINT('Ctrl Pts',(7.21693171141826,638.937681782581,53.9085088387218));
#102445=CARTESIAN_POINT('Ctrl Pts',(7.22513947055269,638.941003823834,53.9143473858616));
#102446=CARTESIAN_POINT('Ctrl Pts',(7.23334108115382,638.944328172037,53.9201966743797));
#102447=CARTESIAN_POINT('Ctrl Pts',(7.24153649808195,638.947654776522,53.92605666394));
#102448=CARTESIAN_POINT('Ctrl Pts',(7.60433131784438,639.09491694573,54.1854667555743));
#102449=CARTESIAN_POINT('Ctrl Pts',(7.95512168437114,639.246660216953,54.4659556720753));
#102450=CARTESIAN_POINT('Ctrl Pts',(8.28995998193701,639.398498406753,54.7640522820467));
#102451=CARTESIAN_POINT('Ctrl Pts',(8.55084003077369,639.51679895558,54.9963060556824));
#102452=CARTESIAN_POINT('Ctrl Pts',(8.80203719278185,639.635157211398,55.2392478412932));
#102453=CARTESIAN_POINT('Ctrl Pts',(9.04170368382722,639.75150971375,55.4912341838178));
#102454=CARTESIAN_POINT('Ctrl Pts',(9.04882604992424,639.754967456693,55.4987226690669));
#102455=CARTESIAN_POINT('Ctrl Pts',(9.05593912941169,639.7584237756,55.5062195590408));
#102456=CARTESIAN_POINT('Ctrl Pts',(9.06304292057168,639.761878644838,55.51372486464));
#102457=CARTESIAN_POINT('Ctrl Pts',(9.41782794429989,639.934425364931,55.8885627455857));
#102458=CARTESIAN_POINT('Ctrl Pts',(9.74946630676366,640.103354072031,56.2843874740499));
#102459=CARTESIAN_POINT('Ctrl Pts',(10.0578808157674,640.265564551166,56.7027531624886));
#102460=CARTESIAN_POINT('Ctrl Pts',(10.2247778709026,640.353343985951,56.9291497791573));
#102461=CARTESIAN_POINT('Ctrl Pts',(10.3848733586231,640.439156313795,57.1621477031083));
#102462=CARTESIAN_POINT('Ctrl Pts',(10.5381498361278,640.522511090264,57.4019967994255));
#102463=CARTESIAN_POINT('Ctrl Pts',(10.5430825010644,640.525193570903,57.4097154999511));
#102464=CARTESIAN_POINT('Ctrl Pts',(10.5480074933753,640.527873218049,57.4174407015242));
#102465=CARTESIAN_POINT('Ctrl Pts',(10.552924779657,640.5305499995,57.4251723494433));
#102466=CARTESIAN_POINT('Ctrl Pts',(10.7311538823148,640.627571065319,57.7054091694609));
#102467=CARTESIAN_POINT('Ctrl Pts',(10.8991800314946,640.720784301005,57.9939850693816));
#102468=CARTESIAN_POINT('Ctrl Pts',(11.055494941017,640.808699365534,58.2883985364575));
#102469=CARTESIAN_POINT('Ctrl Pts',(11.0884477683194,640.827232785971,58.3504639924381));
#102470=CARTESIAN_POINT('Ctrl Pts',(11.1208800201698,640.845530717851,58.412789017301));
#102471=CARTESIAN_POINT('Ctrl Pts',(11.1527773651984,640.863579132001,58.4753503757855));
#102472=CARTESIAN_POINT('Ctrl Pts',(11.1563744083562,640.865614440099,58.48240538009));
#102473=CARTESIAN_POINT('Ctrl Pts',(11.1599650069621,640.86764677106,58.4894639315986));
#102474=CARTESIAN_POINT('Ctrl Pts',(11.1635491598044,640.869676117202,58.4965260351483));
#102475=CARTESIAN_POINT('Ctrl Pts',(11.3468191789592,640.973443540843,58.8576355943088));
#102476=CARTESIAN_POINT('Ctrl Pts',(11.5131975113051,641.069382235403,59.2279486399778));
#102477=CARTESIAN_POINT('Ctrl Pts',(11.6624107054815,641.156407018995,59.6078507224401));
#102478=CARTESIAN_POINT('Ctrl Pts',(11.6647417380394,641.157766534184,59.613785613975));
#102479=CARTESIAN_POINT('Ctrl Pts',(11.6670685829227,641.159123875855,59.6197228445413));
#102480=CARTESIAN_POINT('Ctrl Pts',(11.6693912367388,641.160479039298,59.6256624167821));
#102481=CARTESIAN_POINT('Ctrl Pts',(11.791461484725,641.231701507476,59.9378247594141));
#102482=CARTESIAN_POINT('Ctrl Pts',(11.9019377577645,641.296895212091,60.2563928914153));
#102483=CARTESIAN_POINT('Ctrl Pts',(12.0003794520937,641.355405979746,60.5818958374238));
#102484=CARTESIAN_POINT('Ctrl Pts',(12.0224039614789,641.368496682422,60.6547211045843));
#102485=CARTESIAN_POINT('Ctrl Pts',(12.0438259072343,641.381252781993,60.7278935919235));
#102486=CARTESIAN_POINT('Ctrl Pts',(12.0646400666275,641.393666799833,60.80141938881));
#102487=CARTESIAN_POINT('Ctrl Pts',(12.0658734024639,641.394402388178,60.8057761345467));
#102488=CARTESIAN_POINT('Ctrl Pts',(12.0671044404052,641.395136677262,60.8101336095226));
#102489=CARTESIAN_POINT('Ctrl Pts',(12.0683331795544,641.395869665849,60.8144918087508));
#102490=CARTESIAN_POINT('Ctrl Pts',(12.1541174147233,641.447043151603,61.1187588191497));
#102491=CARTESIAN_POINT('Ctrl Pts',(12.228649207192,641.49184978824,61.4263757001361));
#102492=CARTESIAN_POINT('Ctrl Pts',(12.2916497337314,641.529885155632,61.7356739632629));
#102493=CARTESIAN_POINT('Ctrl Pts',(12.312390183329,641.542406806856,61.8374982715564));
#102494=CARTESIAN_POINT('Ctrl Pts',(12.3318805284049,641.554194394784,61.9395049355668));
#102495=CARTESIAN_POINT('Ctrl Pts',(12.3501097718202,641.565232888749,62.0416346902988));
#102496=CARTESIAN_POINT('Ctrl Pts',(12.3505132822593,641.565477229528,62.0438953667977));
#102497=CARTESIAN_POINT('Ctrl Pts',(12.3509161912353,641.565721211449,62.0461561431484));
#102498=CARTESIAN_POINT('Ctrl Pts',(12.3513184986724,641.565964834433,62.048417019426));
#102499=CARTESIAN_POINT('Ctrl Pts',(12.4988878701167,641.655327563793,62.8777233171341));
#102500=CARTESIAN_POINT('Ctrl Pts',(12.5654436335101,641.696343276042,63.719998294979));
#102501=CARTESIAN_POINT('Ctrl Pts',(12.547023784357,641.685076145265,64.5759864683422));
#102502=CARTESIAN_POINT('Ctrl Pts',(12.5469692630458,641.68504279544,64.5785201263097));
#102503=CARTESIAN_POINT('Ctrl Pts',(12.5469139970635,641.685008987506,64.5810539094377));
#102504=CARTESIAN_POINT('Ctrl Pts',(12.5468579862992,641.684974721356,64.5835878177417));
#102505=CARTESIAN_POINT('Ctrl Pts',(12.5374524690111,641.679220633378,65.0090902838063));
#102506=CARTESIAN_POINT('Ctrl Pts',(12.5068775203495,641.660503714393,65.4317526596763));
#102507=CARTESIAN_POINT('Ctrl Pts',(12.4564407748525,641.629795989302,65.8474537330173));
#102508=CARTESIAN_POINT('Ctrl Pts',(12.4558465628446,641.62943421142,65.8523512450805));
#102509=CARTESIAN_POINT('Ctrl Pts',(12.4552495926927,641.629070768235,65.8572478053186));
#102510=CARTESIAN_POINT('Ctrl Pts',(12.4546498665094,641.628705661322,65.8621434068506));
#102511=CARTESIAN_POINT('Ctrl Pts',(12.4040416607679,641.597895924734,66.2752612870232));
#102512=CARTESIAN_POINT('Ctrl Pts',(12.3337717584624,641.55521695327,66.6829679693347));
#102513=CARTESIAN_POINT('Ctrl Pts',(12.2443814590765,641.50138783171,67.0853656096814));
#102514=CARTESIAN_POINT('Ctrl Pts',(12.2428405235091,641.500459909904,67.0923022553853));
#102515=CARTESIAN_POINT('Ctrl Pts',(12.2412939039662,641.499528674119,67.0992373326653));
#102516=CARTESIAN_POINT('Ctrl Pts',(12.2397416031979,641.498594128006,67.1061708425375));
#102517=CARTESIAN_POINT('Ctrl Pts',(12.150177183183,641.444672824668,67.5062194691017));
#102518=CARTESIAN_POINT('Ctrl Pts',(12.0416978792334,641.379727280723,67.9010490570524));
#102519=CARTESIAN_POINT('Ctrl Pts',(11.914246482633,641.30433460348,68.2907180385381));
#102520=CARTESIAN_POINT('Ctrl Pts',(11.9114061210395,641.302654414243,68.2994021396051));
#102521=CARTESIAN_POINT('Ctrl Pts',(11.9085563276577,641.300969032295,68.3080836988315));
#102522=CARTESIAN_POINT('Ctrl Pts',(11.9056971018176,641.29927846412,68.3167627159898));
#102523=CARTESIAN_POINT('Ctrl Pts',(11.7780348473212,641.223795883638,68.7042742170754));
#102524=CARTESIAN_POINT('Ctrl Pts',(11.63045559295,641.13733782012,69.0888496165626));
#102525=CARTESIAN_POINT('Ctrl Pts',(11.4674585767456,641.043351164257,69.4598550915683));
#102526=CARTESIAN_POINT('Ctrl Pts',(11.4630803893133,641.040826632183,69.4698204979656));
#102527=CARTESIAN_POINT('Ctrl Pts',(11.458691033693,641.038296635479,69.4797762480409));
#102528=CARTESIAN_POINT('Ctrl Pts',(11.4542905965529,641.035761240617,69.4897221352274));
#102529=CARTESIAN_POINT('Ctrl Pts',(11.2649214349003,640.926652626114,69.9177351390396));
#102530=CARTESIAN_POINT('Ctrl Pts',(11.0548558465911,640.807348643409,70.3297521125393));
#102531=CARTESIAN_POINT('Ctrl Pts',(10.8247037221897,640.679801375466,70.7266992259515));
#102532=CARTESIAN_POINT('Ctrl Pts',(10.6530709447778,640.584684756816,71.0227170695312));
#102533=CARTESIAN_POINT('Ctrl Pts',(10.470268352681,640.484984565181,71.3103549097642));
#102534=CARTESIAN_POINT('Ctrl Pts',(10.2765612833766,640.381519680905,71.5900073533417));
#102535=CARTESIAN_POINT('Ctrl Pts',(10.26913038327,640.377550609346,71.6007352497487));
#102536=CARTESIAN_POINT('Ctrl Pts',(10.2616833989456,640.373575989167,71.6114514209664));
#102537=CARTESIAN_POINT('Ctrl Pts',(10.2542203448061,640.369595866016,71.6221558912206));
#102538=CARTESIAN_POINT('Ctrl Pts',(10.0309413485718,640.250518892223,71.9424112891989));
#102539=CARTESIAN_POINT('Ctrl Pts',(9.79314227964304,640.126485515932,72.2520967897448));
#102540=CARTESIAN_POINT('Ctrl Pts',(9.54042013959494,639.998687759293,72.5513581119671));
#102541=CARTESIAN_POINT('Ctrl Pts',(9.53153439293211,639.994194371855,72.5618801829449));
#102542=CARTESIAN_POINT('Ctrl Pts',(9.52263008694159,639.989696280727,72.5723894853929));
#102543=CARTESIAN_POINT('Ctrl Pts',(9.51370721162859,639.985193542565,72.5828860130588));
#102544=CARTESIAN_POINT('Ctrl Pts',(9.3115180637735,639.883163114011,72.8207335576842));
#102545=CARTESIAN_POINT('Ctrl Pts',(9.10007725182296,639.778925091646,73.0514824787519));
#102546=CARTESIAN_POINT('Ctrl Pts',(8.8816208225359,639.674324548391,73.2729706357969));
#102547=CARTESIAN_POINT('Ctrl Pts',(8.82635703926505,639.647863337012,73.3290013671786));
#102548=CARTESIAN_POINT('Ctrl Pts',(8.77064449616043,639.621378982489,73.3844395960483));
#102549=CARTESIAN_POINT('Ctrl Pts',(8.71451977111152,639.594901428748,73.4392506659581));
#102550=CARTESIAN_POINT('Ctrl Pts',(8.70451527424171,639.590181679951,73.4490209976055));
#102551=CARTESIAN_POINT('Ctrl Pts',(8.69449736220672,639.585461993116,73.4587717209558));
#102552=CARTESIAN_POINT('Ctrl Pts',(8.68446623164618,639.580742533684,73.4685026450421));
#102553=CARTESIAN_POINT('Ctrl Pts',(8.35856609470834,639.427412610826,73.7846494116626));
#102554=CARTESIAN_POINT('Ctrl Pts',(8.01730513116886,639.273445263822,74.081986796801));
#102555=CARTESIAN_POINT('Ctrl Pts',(7.65987184773939,639.121443315517,74.3606572776207));
#102556=CARTESIAN_POINT('Ctrl Pts',(7.39538695995618,639.008968568188,74.5668611603172));
#102557=CARTESIAN_POINT('Ctrl Pts',(7.12204759184878,638.897570561306,74.7628452062894));
#102558=CARTESIAN_POINT('Ctrl Pts',(6.83953361923845,638.788308851806,74.9486824712654));
#102559=CARTESIAN_POINT('Ctrl Pts',(6.8283183754522,638.783971378876,74.9560598417084));
#102560=CARTESIAN_POINT('Ctrl Pts',(6.81708850557552,638.77963722266,74.9634213086029));
#102561=CARTESIAN_POINT('Ctrl Pts',(6.80584399584154,638.775306452619,74.9707668709571));
#102562=CARTESIAN_POINT('Ctrl Pts',(6.53600531050182,638.671379352018,75.1470410648213));
#102563=CARTESIAN_POINT('Ctrl Pts',(6.25682003400716,638.569197778981,75.3144018558145));
#102564=CARTESIAN_POINT('Ctrl Pts',(5.97168962520577,638.471187254382,75.4705491677874));
#102565=CARTESIAN_POINT('Ctrl Pts',(5.91058146393213,638.450181978343,75.5040141186588));
#102566=CARTESIAN_POINT('Ctrl Pts',(5.84920038485744,638.429368272628,75.5369641331853));
#102567=CARTESIAN_POINT('Ctrl Pts',(5.78758008341291,638.408769967278,75.5693767842875));
#102568=CARTESIAN_POINT('Ctrl Pts',(5.77645936187983,638.405052555768,75.5752263510472));
#102569=CARTESIAN_POINT('Ctrl Pts',(5.76533057667264,638.401342057466,75.5810585770746));
#102570=CARTESIAN_POINT('Ctrl Pts',(5.75419392195765,638.39763861286,75.5868733289663));
#102571=CARTESIAN_POINT('Ctrl Pts',(5.43563539119555,638.291703401373,75.7532014469483));
#102572=CARTESIAN_POINT('Ctrl Pts',(5.10974723267518,638.191150407059,75.9059290152506));
#102573=CARTESIAN_POINT('Ctrl Pts',(4.77620299466647,638.097497832909,76.0448419303968));
#102574=CARTESIAN_POINT('Ctrl Pts',(4.74275640441732,638.088106696992,76.0587716069547));
#102575=CARTESIAN_POINT('Ctrl Pts',(4.70923285125379,638.078784938588,76.0725624092196));
#102576=CARTESIAN_POINT('Ctrl Pts',(4.67563202082697,638.069534081832,76.0862141459991));
#102577=CARTESIAN_POINT('Ctrl Pts',(4.66519251392584,638.06665991528,76.0904556304658));
#102578=CARTESIAN_POINT('Ctrl Pts',(4.65474549323414,638.063792577535,76.0946837135968));
#102579=CARTESIAN_POINT('Ctrl Pts',(4.64429094472362,638.060932112898,76.0988983916671));
#102580=CARTESIAN_POINT('Ctrl Pts',(4.27379986217441,637.959562203058,76.2482592788739));
#102581=CARTESIAN_POINT('Ctrl Pts',(3.89386018446253,637.86681693476,76.3807926409731));
#102582=CARTESIAN_POINT('Ctrl Pts',(3.50348924748349,637.784945316901,76.4956462456033));
#102583=CARTESIAN_POINT('Ctrl Pts',(3.49421925398876,637.783001142033,76.4983736314482));
#102584=CARTESIAN_POINT('Ctrl Pts',(3.4849433167112,637.781063089165,76.5010910617607));
#102585=CARTESIAN_POINT('Ctrl Pts',(3.47566142285349,637.779131189023,76.5037985243145));
#102586=CARTESIAN_POINT('Ctrl Pts',(3.1135796752967,637.703768790973,76.6094151999565));
#102587=CARTESIAN_POINT('Ctrl Pts',(2.74384243019707,637.638239420645,76.6992121831809));
#102588=CARTESIAN_POINT('Ctrl Pts',(2.3719816618457,637.5847920319,76.7716691688675));
#102589=CARTESIAN_POINT('Ctrl Pts',(2.34061880023512,637.580284261252,76.7777802152811));
#102590=CARTESIAN_POINT('Ctrl Pts',(2.30924086293913,637.575862440254,76.7837679159765));
#102591=CARTESIAN_POINT('Ctrl Pts',(2.27785118480889,637.571527921841,76.7896313582787));
#102592=CARTESIAN_POINT('Ctrl Pts',(2.27065610270346,637.570534371804,76.7909753653312));
#102593=CARTESIAN_POINT('Ctrl Pts',(2.26346025582311,637.569545385811,76.7923128747317));
#102594=CARTESIAN_POINT('Ctrl Pts',(2.25626368658222,637.568560981047,76.7936438742463));
#102595=CARTESIAN_POINT('Ctrl Pts',(1.96925816375727,637.529302051626,76.8467253077398));
#102596=CARTESIAN_POINT('Ctrl Pts',(1.68006019104803,637.497124903821,76.8898579427876));
#102597=CARTESIAN_POINT('Ctrl Pts',(1.38876410941254,637.472468422105,76.9227278834574));
#102598=CARTESIAN_POINT('Ctrl Pts',(1.10512361178556,637.448459940066,76.9547339656408));
#102599=CARTESIAN_POINT('Ctrl Pts',(0.819493826338199,637.431582163689,
76.9770097040753));
#102600=CARTESIAN_POINT('Ctrl Pts',(0.531969592107279,637.422213051343,
76.989304983325));
#102601=CARTESIAN_POINT('Ctrl Pts',(0.271955131226084,637.413740357895,
77.000423873578));
#102602=CARTESIAN_POINT('Ctrl Pts',(0.0103914694409467,637.411408035635,
77.003381168988));
#102603=CARTESIAN_POINT('Ctrl Pts',(-0.252645464510395,637.415474030314,
76.9980210944396));
#102604=CARTESIAN_POINT('',(0.264827872760508,637.216574016203,52.0023253862613));
#102605=CARTESIAN_POINT('Origin',(0.270210553101161,637.216574016203,51.7523833394738));
#102606=CARTESIAN_POINT('',(-3.86212967253593E-9,637.214372791556,76.5994959777072));
#102607=CARTESIAN_POINT('Ctrl Pts',(-3.25135893208817E-9,637.214372791556,
76.5994959777073));
#102608=CARTESIAN_POINT('Ctrl Pts',(0.310528165472536,637.214386003673,
76.5995448311342));
#102609=CARTESIAN_POINT('Ctrl Pts',(0.618777498408002,637.223529415885,
76.5878893241728));
#102610=CARTESIAN_POINT('Ctrl Pts',(0.92467364940843,637.241314282396,76.564836683329));
#102611=CARTESIAN_POINT('Ctrl Pts',(1.23978245630703,637.259634774658,76.5410897674936));
#102612=CARTESIAN_POINT('Ctrl Pts',(1.55239421536144,637.287124882276,76.5052488949338));
#102613=CARTESIAN_POINT('Ctrl Pts',(1.86243766898481,637.323219022104,76.4576945787577));
#102614=CARTESIAN_POINT('Ctrl Pts',(1.97909517691913,637.336799868124,76.4398017061562));
#102615=CARTESIAN_POINT('Ctrl Pts',(2.09538918047889,637.351598516929,76.4202509684407));
#102616=CARTESIAN_POINT('Ctrl Pts',(2.21131621964626,637.367583834262,76.3990641890932));
#102617=CARTESIAN_POINT('Ctrl Pts',(2.28847278600611,637.37822304498,76.3849630858612));
#102618=CARTESIAN_POINT('Ctrl Pts',(2.36554368200416,637.389403280499,76.3701075120779));
#102619=CARTESIAN_POINT('Ctrl Pts',(2.44247543406213,637.401102268236,76.354512897056));
#102620=CARTESIAN_POINT('Ctrl Pts',(2.64351074550122,637.431673645855,76.3137616051143));
#102621=CARTESIAN_POINT('Ctrl Pts',(2.8440260578588,637.465865757867,76.2678728545131));
#102622=CARTESIAN_POINT('Ctrl Pts',(3.04288942630178,637.503285001264,76.2171146986249));
#102623=CARTESIAN_POINT('Ctrl Pts',(3.16477478014477,637.526219630993,76.1860045155917));
#102624=CARTESIAN_POINT('Ctrl Pts',(3.28603954227595,637.550365906112,76.1530659810039));
#102625=CARTESIAN_POINT('Ctrl Pts',(3.40642527297713,637.57562795491,76.1183685737292));
#102626=CARTESIAN_POINT('Ctrl Pts',(3.47943076865769,637.590947614339,76.0973270316614));
#102627=CARTESIAN_POINT('Ctrl Pts',(3.55205443377299,637.606657828165,76.0756654689925));
#102628=CARTESIAN_POINT('Ctrl Pts',(3.624292679273,637.622740245025,76.0533936492376));
#102629=CARTESIAN_POINT('Ctrl Pts',(3.94018000276088,637.693066310974,75.9560022261365));
#102630=CARTESIAN_POINT('Ctrl Pts',(4.24915881614502,637.770600446213,75.8468009339012));
#102631=CARTESIAN_POINT('Ctrl Pts',(4.55177540581521,637.854075900525,75.7262558160285));
#102632=CARTESIAN_POINT('Ctrl Pts',(4.61866590223142,637.872527349547,75.6996104732076));
#102633=CARTESIAN_POINT('Ctrl Pts',(4.68524538832333,637.891269293644,75.6724106564061));
#102634=CARTESIAN_POINT('Ctrl Pts',(4.75151758316339,637.910289739806,75.6446572600295));
#102635=CARTESIAN_POINT('Ctrl Pts',(5.00694798017803,637.983599521175,75.537688401188));
#102636=CARTESIAN_POINT('Ctrl Pts',(5.25788462119999,638.061063217152,75.4224616809293));
#102637=CARTESIAN_POINT('Ctrl Pts',(5.50437127896534,638.141932884419,75.2991083225993));
#102638=CARTESIAN_POINT('Ctrl Pts',(5.54958725702918,638.156767768929,75.2764801495578));
#102639=CARTESIAN_POINT('Ctrl Pts',(5.59465355083892,638.171717219499,75.2535786253479));
#102640=CARTESIAN_POINT('Ctrl Pts',(5.63957051211808,638.18677656011,75.2304047182994));
#102641=CARTESIAN_POINT('Ctrl Pts',(5.70073378556493,638.207282813015,75.1988488878676));
#102642=CARTESIAN_POINT('Ctrl Pts',(5.76165357779709,638.228007610847,75.1667619524568));
#102643=CARTESIAN_POINT('Ctrl Pts',(5.82229488838819,638.248925991892,75.1341674982549));
#102644=CARTESIAN_POINT('Ctrl Pts',(6.03771053817337,638.323234192051,75.0183824754239));
#102645=CARTESIAN_POINT('Ctrl Pts',(6.24993868377269,638.400103047963,74.8960130814583));
#102646=CARTESIAN_POINT('Ctrl Pts',(6.45731962006765,638.478404326221,74.768123123848));
#102647=CARTESIAN_POINT('Ctrl Pts',(6.52890397505861,638.505432589277,74.7239776961683));
#102648=CARTESIAN_POINT('Ctrl Pts',(6.59991097229038,638.532631370786,74.6791748810446));
#102649=CARTESIAN_POINT('Ctrl Pts',(6.67027315473924,638.559953912966,74.6337595519187));
#102650=CARTESIAN_POINT('Ctrl Pts',(6.72531600416889,638.581327760719,74.598232099019));
#102651=CARTESIAN_POINT('Ctrl Pts',(6.78000298293607,638.602786093397,74.5623194192597));
#102652=CARTESIAN_POINT('Ctrl Pts',(6.83433353593326,638.624319539508,74.526023120994));
#102653=CARTESIAN_POINT('Ctrl Pts',(7.10822454753777,638.732873879809,74.3430463371942));
#102654=CARTESIAN_POINT('Ctrl Pts',(7.37336538639476,638.843433750453,74.1501101955193));
#102655=CARTESIAN_POINT('Ctrl Pts',(7.62995416450792,638.954928099765,73.9471842046907));
#102656=CARTESIAN_POINT('Ctrl Pts',(7.8884435207344,639.0672482986,73.7427551212498));
#102657=CARTESIAN_POINT('Ctrl Pts',(8.13825378256586,639.180516194487,73.5281875575904));
#102658=CARTESIAN_POINT('Ctrl Pts',(8.37962080003936,639.293634261351,73.3034909566159));
#102659=CARTESIAN_POINT('Ctrl Pts',(8.42385440908566,639.314364601387,73.2623124157134));
#102660=CARTESIAN_POINT('Ctrl Pts',(8.46780453567413,639.335089918768,73.2207937995264));
#102661=CARTESIAN_POINT('Ctrl Pts',(8.5114727458354,639.355803477485,73.1789353160944));
#102662=CARTESIAN_POINT('Ctrl Pts',(8.55430052500404,639.376118386551,73.1378824339602));
#102663=CARTESIAN_POINT('Ctrl Pts',(8.59688191547822,639.396437541293,73.0964662008016));
#102664=CARTESIAN_POINT('Ctrl Pts',(8.63920055811426,639.416747258165,73.0547024182158));
#102665=CARTESIAN_POINT('Ctrl Pts',(8.79391013170621,639.490996039346,72.902021316154));
#102666=CARTESIAN_POINT('Ctrl Pts',(8.94539579188608,639.565251675653,72.7444053092197));
#102667=CARTESIAN_POINT('Ctrl Pts',(9.09269306745744,639.638775141591,72.5827363034081));
#102668=CARTESIAN_POINT('Ctrl Pts',(9.17109278887125,639.677908378947,72.4966871557392));
#102669=CARTESIAN_POINT('Ctrl Pts',(9.24830637544962,639.716834119649,72.4094906238483));
#102670=CARTESIAN_POINT('Ctrl Pts',(9.32419224683953,639.755441259617,72.3212842918984));
#102671=CARTESIAN_POINT('Ctrl Pts',(9.36129694465004,639.774318373836,72.2781554560291));
#102672=CARTESIAN_POINT('Ctrl Pts',(9.39807441423151,639.793113104251,72.2348034790566));
#102673=CARTESIAN_POINT('Ctrl Pts',(9.43452337359978,639.811820175665,72.1912312995811));
#102674=CARTESIAN_POINT('Ctrl Pts',(9.65091478739477,639.922880949451,71.9325505119194));
#102675=CARTESIAN_POINT('Ctrl Pts',(9.85597586740215,640.030976085533,71.665812843898));
#102676=CARTESIAN_POINT('Ctrl Pts',(10.0499594594973,640.135271225398,71.3908995346973));
#102677=CARTESIAN_POINT('Ctrl Pts',(10.0810275633506,640.151974969265,71.3468698559567));
#102678=CARTESIAN_POINT('Ctrl Pts',(10.1118142187007,640.168581847187,71.3026323420182));
#102679=CARTESIAN_POINT('Ctrl Pts',(10.1423182570292,640.18508833926,71.2581851032761));
#102680=CARTESIAN_POINT('Ctrl Pts',(10.368697236347,640.307587622379,70.9283297434193));
#102681=CARTESIAN_POINT('Ctrl Pts',(10.5795594554243,640.424590868755,70.5868461102142));
#102682=CARTESIAN_POINT('Ctrl Pts',(10.7743498376389,640.534625593794,70.233068626278));
#102683=CARTESIAN_POINT('Ctrl Pts',(10.9361257815805,640.62601086296,69.9392518281467));
#102684=CARTESIAN_POINT('Ctrl Pts',(11.0868167655308,640.712589548309,69.6369556978497));
#102685=CARTESIAN_POINT('Ctrl Pts',(11.2261259025389,640.793526545651,69.325814430765));
#102686=CARTESIAN_POINT('Ctrl Pts',(11.2465333475455,640.805383035166,69.2802352359348));
#102687=CARTESIAN_POINT('Ctrl Pts',(11.2666986076393,640.817120814722,69.2344396511952));
#102688=CARTESIAN_POINT('Ctrl Pts',(11.2866125566538,640.82873286362,69.1884489145415));
#102689=CARTESIAN_POINT('Ctrl Pts',(11.3880924823146,640.887906956016,68.954083719907));
#102690=CARTESIAN_POINT('Ctrl Pts',(11.4831444008195,640.943852057169,68.7144140723365));
#102691=CARTESIAN_POINT('Ctrl Pts',(11.5704748159164,640.995610908571,68.4723906692549));
#102692=CARTESIAN_POINT('Ctrl Pts',(11.6043465274191,641.015685940625,68.3785202018239));
#102693=CARTESIAN_POINT('Ctrl Pts',(11.6370570638028,641.035131394244,68.2842960263096));
#102694=CARTESIAN_POINT('Ctrl Pts',(11.668532669455,641.053892244932,68.1898912049256));
#102695=CARTESIAN_POINT('Ctrl Pts',(11.683669793509,641.062914639206,68.1444904107873));
#102696=CARTESIAN_POINT('Ctrl Pts',(11.698537234685,641.071787880423,68.0990176527924));
#102697=CARTESIAN_POINT('Ctrl Pts',(11.7131347554859,641.080510894475,68.0534740137289));
#102698=CARTESIAN_POINT('Ctrl Pts',(11.8224706417623,641.1458465419,67.7123507360731));
#102699=CARTESIAN_POINT('Ctrl Pts',(11.9167276342155,641.202767414028,67.3670528841897));
#102700=CARTESIAN_POINT('Ctrl Pts',(11.9959228357299,641.25083557254,67.0175313575219));
#102701=CARTESIAN_POINT('Ctrl Pts',(12.0059728443566,641.256935505345,66.973176468702));
#102702=CARTESIAN_POINT('Ctrl Pts',(12.0157803206307,641.262892923904,66.9287535733242));
#102703=CARTESIAN_POINT('Ctrl Pts',(12.0253444381023,641.268706747125,66.8842623710702));
#102704=CARTESIAN_POINT('Ctrl Pts',(12.0802141521749,641.302060877155,66.6290146125976));
#102705=CARTESIAN_POINT('Ctrl Pts',(12.1270883150579,641.330698896874,66.3714346350773));
#102706=CARTESIAN_POINT('Ctrl Pts',(12.1657799000475,641.354400361684,66.1116378612346));
#102707=CARTESIAN_POINT('Ctrl Pts',(12.1805677414234,641.363459011054,66.012344087599));
#102708=CARTESIAN_POINT('Ctrl Pts',(12.1941607596463,641.37179681849,65.9127266173964));
#102709=CARTESIAN_POINT('Ctrl Pts',(12.2065502013075,641.379402497237,65.812792357429));
#102710=CARTESIAN_POINT('Ctrl Pts',(12.2119202405116,641.382699077838,65.769477177574));
#102711=CARTESIAN_POINT('Ctrl Pts',(12.2170645586533,641.385858354091,65.7260864061383));
#102712=CARTESIAN_POINT('Ctrl Pts',(12.2219815693876,641.388879140903,65.6826258242829));
#102713=CARTESIAN_POINT('Ctrl Pts',(12.2489552484072,641.405450537277,65.4442102811187));
#102714=CARTESIAN_POINT('Ctrl Pts',(12.2691246111521,641.417870627053,65.2033421763435));
#102715=CARTESIAN_POINT('Ctrl Pts',(12.2821848003886,641.425918961536,64.9610218376528));
#102716=CARTESIAN_POINT('Ctrl Pts',(12.2891074986869,641.430185070581,64.8325772519037));
#102717=CARTESIAN_POINT('Ctrl Pts',(12.2940334684438,641.433223291306,64.7037249406801));
#102718=CARTESIAN_POINT('Ctrl Pts',(12.2969222724657,641.435003822481,64.5746151917459));
#102719=CARTESIAN_POINT('Ctrl Pts',(12.297866127023,641.435585572732,64.5324313592704));
#102720=CARTESIAN_POINT('Ctrl Pts',(12.2985942535798,641.436033507889,64.4902847021331));
#102721=CARTESIAN_POINT('Ctrl Pts',(12.2991072457852,641.43634820398,64.4481760965921));
#102722=CARTESIAN_POINT('Ctrl Pts',(12.3039230418204,641.439302463655,64.0528748551926));
#102723=CARTESIAN_POINT('Ctrl Pts',(12.2897795816084,641.430514251088,63.6605870250526));
#102724=CARTESIAN_POINT('Ctrl Pts',(12.2571208090154,641.410420092158,63.2713649049953));
#102725=CARTESIAN_POINT('Ctrl Pts',(12.2244620364223,641.390325933228,62.8821427849379));
#102726=CARTESIAN_POINT('Ctrl Pts',(12.1732881572924,641.358926028386,62.4959863338011));
#102727=CARTESIAN_POINT('Ctrl Pts',(12.1040930127778,641.316687091337,62.1129397664499));
#102728=CARTESIAN_POINT('Ctrl Pts',(12.097501651259,641.312663512714,62.076451680159));
#102729=CARTESIAN_POINT('Ctrl Pts',(12.0907423182806,641.308539354126,62.0399811711845));
#102730=CARTESIAN_POINT('Ctrl Pts',(12.083815675173,641.304315434519,62.0035314922614));
#102731=CARTESIAN_POINT('Ctrl Pts',(12.0363940815464,641.275397386341,61.7539875450918));
#102732=CARTESIAN_POINT('Ctrl Pts',(11.9810777244786,641.241765390489,61.5051624947921));
#102733=CARTESIAN_POINT('Ctrl Pts',(11.9180804827761,641.203688800903,61.2582463139588));
#102734=CARTESIAN_POINT('Ctrl Pts',(11.8885070000971,641.185814091913,61.1423337565242));
#102735=CARTESIAN_POINT('Ctrl Pts',(11.8572414900855,641.166960298106,61.0268418090731));
#102736=CARTESIAN_POINT('Ctrl Pts',(11.824309419125,641.147157255363,60.9118928329591));
#102737=CARTESIAN_POINT('Ctrl Pts',(11.8147012792868,641.141379592485,60.8783557426836));
#102738=CARTESIAN_POINT('Ctrl Pts',(11.8049614391109,641.135527263631,60.8448961507762));
#102739=CARTESIAN_POINT('Ctrl Pts',(11.7950906598908,641.129601189148,60.8115140280203));
#102740=CARTESIAN_POINT('Ctrl Pts',(11.6884979670894,641.065606622677,60.4510267476747));
#102741=CARTESIAN_POINT('Ctrl Pts',(11.5665815949929,640.992974536206,60.0993881528899));
#102742=CARTESIAN_POINT('Ctrl Pts',(11.4300925444937,640.912719421956,59.7560189685529));
#102743=CARTESIAN_POINT('Ctrl Pts',(11.4183382568568,640.905807939359,59.7264483902275));
#102744=CARTESIAN_POINT('Ctrl Pts',(11.4064758513312,640.89883987044,59.6969391717302));
#102745=CARTESIAN_POINT('Ctrl Pts',(11.3945054923629,640.891815783686,59.6674910998064));
#102746=CARTESIAN_POINT('Ctrl Pts',(11.2921850121202,640.831775150665,59.4157742657978));
#102747=CARTESIAN_POINT('Ctrl Pts',(11.1819396277238,640.767620977233,59.1684441713329));
#102748=CARTESIAN_POINT('Ctrl Pts',(11.0639479787746,640.699754720745,58.9255372140161));
#102749=CARTESIAN_POINT('Ctrl Pts',(11.020546532114,640.674791142921,58.8361875571092));
#102750=CARTESIAN_POINT('Ctrl Pts',(10.9760974099167,640.649325512844,58.7474361315046));
#102751=CARTESIAN_POINT('Ctrl Pts',(10.9306109324387,640.623378466979,58.6592839633751));
#102752=CARTESIAN_POINT('Ctrl Pts',(10.9173036742458,640.615787550781,58.6334946799086));
#102753=CARTESIAN_POINT('Ctrl Pts',(10.9039026380964,640.608152673949,58.6077492085214));
#102754=CARTESIAN_POINT('Ctrl Pts',(10.8904091198925,640.600475021888,58.5820495569515));
#102755=CARTESIAN_POINT('Ctrl Pts',(10.7698070167312,640.53185385342,58.3523517136592));
#102756=CARTESIAN_POINT('Ctrl Pts',(10.6416424932156,640.459709701766,58.1259903442911));
#102757=CARTESIAN_POINT('Ctrl Pts',(10.5068163413095,640.384883069019,57.9044450451186));
#102758=CARTESIAN_POINT('Ctrl Pts',(10.4485076621598,640.352522565815,57.8086326705612));
#102759=CARTESIAN_POINT('Ctrl Pts',(10.3889536073115,640.319660622561,57.713720804039));
#102760=CARTESIAN_POINT('Ctrl Pts',(10.3282293807528,640.286366224327,57.6198275512506));
#102761=CARTESIAN_POINT('Ctrl Pts',(10.3139692496735,640.27854755771,57.597778195201));
#102762=CARTESIAN_POINT('Ctrl Pts',(10.2996497960813,640.270707523277,57.5757900176145));
#102763=CARTESIAN_POINT('Ctrl Pts',(10.2852711775002,640.262846614506,57.5538629682177));
#102764=CARTESIAN_POINT('Ctrl Pts',(10.0352430737247,640.126154198402,57.1725760906817));
#102765=CARTESIAN_POINT('Ctrl Pts',(9.76709513330229,639.983017170431,56.8094299412362));
#102766=CARTESIAN_POINT('Ctrl Pts',(9.48107593712361,639.835696654845,56.4634525360726));
#102767=CARTESIAN_POINT('Ctrl Pts',(9.28311236321487,639.733731135868,56.2239898547808));
#102768=CARTESIAN_POINT('Ctrl Pts',(9.07658839348234,639.629761831818,55.9927510172857));
#102769=CARTESIAN_POINT('Ctrl Pts',(8.86159725045972,639.524539530591,55.7694040901285));
#102770=CARTESIAN_POINT('Ctrl Pts',(8.84757081570353,639.517674625729,55.75483250798));
#102771=CARTESIAN_POINT('Ctrl Pts',(8.83350480090612,639.510803005305,55.7402928849304));
#102772=CARTESIAN_POINT('Ctrl Pts',(8.81939960411072,639.503925105357,55.7257855526291));
#102773=CARTESIAN_POINT('Ctrl Pts',(8.49324152366855,639.344885662151,55.3903287898225));
#102774=CARTESIAN_POINT('Ctrl Pts',(8.14587360450725,639.182353336129,55.0718764699218));
#102775=CARTESIAN_POINT('Ctrl Pts',(7.78212530166576,639.02170993629,54.7745772655406));
#102776=CARTESIAN_POINT('Ctrl Pts',(7.55195563852923,638.920059325312,54.5864547170954));
#102777=CARTESIAN_POINT('Ctrl Pts',(7.31522835413135,638.819165518536,54.4068014680504));
#102778=CARTESIAN_POINT('Ctrl Pts',(7.07317494872264,638.720393123171,54.2366615516199));
#102779=CARTESIAN_POINT('Ctrl Pts',(7.06129788050288,638.715546562653,54.2283131320183));
#102780=CARTESIAN_POINT('Ctrl Pts',(7.04940682153739,638.710704346424,54.219985871321));
#102781=CARTESIAN_POINT('Ctrl Pts',(7.03750173377691,638.705866579126,54.2116797798133));
#102782=CARTESIAN_POINT('Ctrl Pts',(6.64028634979692,638.544453607337,53.9345455499819));
#102783=CARTESIAN_POINT('Ctrl Pts',(6.22730832298175,638.387924142036,53.6808812320082));
#102784=CARTESIAN_POINT('Ctrl Pts',(5.79712163884134,638.2401609909,53.45108975874));
#102785=CARTESIAN_POINT('Ctrl Pts',(5.54446643548225,638.153377437676,53.3161297203447));
#102786=CARTESIAN_POINT('Ctrl Pts',(5.28587575783202,638.069617723393,53.1894035722665));
#102787=CARTESIAN_POINT('Ctrl Pts',(5.02106131531316,637.989666687543,53.0709860658359));
#102788=CARTESIAN_POINT('Ctrl Pts',(5.01259930724038,637.987111893687,53.0672020958763));
#102789=CARTESIAN_POINT('Ctrl Pts',(5.00412957485698,637.984560747639,53.0634263089924));
#102790=CARTESIAN_POINT('Ctrl Pts',(4.9956522280165,637.982013310887,53.0596587598676));
#102791=CARTESIAN_POINT('Ctrl Pts',(4.72092237015458,637.899457182191,52.9375618048865));
#102792=CARTESIAN_POINT('Ctrl Pts',(4.43801237504386,637.820746463645,52.8240393805747));
#102793=CARTESIAN_POINT('Ctrl Pts',(4.15077506061875,637.748019723362,52.7210258524583));
#102794=CARTESIAN_POINT('Ctrl Pts',(4.06518506628605,637.726348857579,52.6903302330353));
#102795=CARTESIAN_POINT('Ctrl Pts',(3.97921111129791,637.705209220218,52.660567473289));
#102796=CARTESIAN_POINT('Ctrl Pts',(3.89295563852527,637.684657074927,52.631788096699));
#102797=CARTESIAN_POINT('Ctrl Pts',(3.88647932075825,637.683113958654,52.6296272553988));
#102798=CARTESIAN_POINT('Ctrl Pts',(3.88000131269557,637.681574078487,52.6274718253079));
#102799=CARTESIAN_POINT('Ctrl Pts',(3.87352161455212,637.680037443336,52.6253218076544));
#102800=CARTESIAN_POINT('Ctrl Pts',(3.49528738953933,637.590340671551,52.4998205508172));
#102801=CARTESIAN_POINT('Ctrl Pts',(3.11117130680274,637.511675562861,52.3927215905075));
#102802=CARTESIAN_POINT('Ctrl Pts',(2.72090801980653,637.445755536795,52.3041975366685));
#102803=CARTESIAN_POINT('Ctrl Pts',(2.71660777482107,637.445029175205,52.3032221051296));
#102804=CARTESIAN_POINT('Ctrl Pts',(2.71230668873312,637.444304366729,52.3022489124891));
#102805=CARTESIAN_POINT('Ctrl Pts',(2.70800476328749,637.44358111362,52.3012779602549));
#102806=CARTESIAN_POINT('Ctrl Pts',(2.51064590304966,637.410400527148,52.2567337140315));
#102807=CARTESIAN_POINT('Ctrl Pts',(2.31170028173491,637.380523021655,52.2169417014671));
#102808=CARTESIAN_POINT('Ctrl Pts',(2.11111770838934,637.35412628928,52.1819925296957));
#102809=CARTESIAN_POINT('Ctrl Pts',(1.91053513504378,637.327729556906,52.1470433579242));
#102810=CARTESIAN_POINT('Ctrl Pts',(1.70831537286292,637.304813279245,52.116936815071));
#102811=CARTESIAN_POINT('Ctrl Pts',(1.50439479076096,637.285586274148,52.0918063490636));
#102812=CARTESIAN_POINT('Ctrl Pts',(1.36067001764642,637.272034935108,52.0740942059933));
#102813=CARTESIAN_POINT('Ctrl Pts',(1.21594950307129,637.260306033537,52.0588407343316));
#102814=CARTESIAN_POINT('Ctrl Pts',(1.07058065255011,637.250510636707,52.0461417320882));
#102815=CARTESIAN_POINT('Ctrl Pts',(0.927490453078941,637.24086878234,52.0336417862087));
#102816=CARTESIAN_POINT('Ctrl Pts',(0.783772258610834,637.233100409219,
52.0236168794799));
#102817=CARTESIAN_POINT('Ctrl Pts',(0.639767420114975,637.227281790098,
52.0161192211438));
#102818=CARTESIAN_POINT('Ctrl Pts',(0.514927066398998,637.222237525774,
52.0096193678855));
#102819=CARTESIAN_POINT('Ctrl Pts',(0.389871499267673,637.218658197405,
52.0050182899915));
#102820=CARTESIAN_POINT('Ctrl Pts',(0.264827872760508,637.216574016203,
52.0023253862613));
#102821=CARTESIAN_POINT('',(-0.247612686332903,637.216296403659,76.5969814761947));
#102822=CARTESIAN_POINT('Origin',(0.00102225664371531,643.230913064776,
68.9078455093003));
#102823=CARTESIAN_POINT('Origin',(-0.252645464510396,637.216296403659,76.8469308133488));
#102824=CARTESIAN_POINT('Origin',(0.,22.7782939407039,64.2994740882088));
#102825=CARTESIAN_POINT('',(-3.417213350044E-14,635.742307759052,51.9994740882088));
#102826=CARTESIAN_POINT('Ctrl Pts',(-4.02455846426619E-15,635.742307759052,
51.9994740882088));
#102827=CARTESIAN_POINT('Ctrl Pts',(-0.803517342471636,635.742307759052,
51.9994740882088));
#102828=CARTESIAN_POINT('Ctrl Pts',(-1.62216512710203,635.808561272943,
52.0793396645949));
#102829=CARTESIAN_POINT('Ctrl Pts',(-3.23077935439454,636.064326910425,
52.4030388996346));
#102830=CARTESIAN_POINT('Ctrl Pts',(-4.02089381669516,636.253138677506,
52.6466899325635));
#102831=CARTESIAN_POINT('Ctrl Pts',(-6.27564182199435,636.933990415857,
53.5959081295421));
#102832=CARTESIAN_POINT('Ctrl Pts',(-7.62604171070064,637.536810853389,
54.5306889817204));
#102833=CARTESIAN_POINT('Ctrl Pts',(-9.75980156458901,638.60355417627,56.6644488356087));
#102834=CARTESIAN_POINT('Ctrl Pts',(-10.7006947361121,639.148581736175,
58.017090947518));
#102835=CARTESIAN_POINT('Ctrl Pts',(-11.654095320228,639.721789350985,60.2816553316396));
#102836=CARTESIAN_POINT('Ctrl Pts',(-11.8983125166469,639.873458090211,
61.0753972970467));
#102837=CARTESIAN_POINT('Ctrl Pts',(-12.2213288811781,640.075308832797,
62.6858966089289));
#102838=CARTESIAN_POINT('Ctrl Pts',(-12.3,640.125373764374,63.5026943063123));
#102839=CARTESIAN_POINT('Ctrl Pts',(-12.3,640.125373764374,65.0962538701053));
#102840=CARTESIAN_POINT('Ctrl Pts',(-12.2213288811781,640.075308832797,
65.9130515674887));
#102841=CARTESIAN_POINT('Ctrl Pts',(-11.8983125166469,639.873458090211,
67.5235508793709));
#102842=CARTESIAN_POINT('Ctrl Pts',(-11.654095320228,639.721789350985,68.317292844778));
#102843=CARTESIAN_POINT('Ctrl Pts',(-10.7006947361121,639.148581736175,
70.5818572288996));
#102844=CARTESIAN_POINT('Ctrl Pts',(-9.75980156458901,638.60355417627,71.9344993408089));
#102845=CARTESIAN_POINT('Ctrl Pts',(-7.62604171070064,637.536810853389,
74.0682591946972));
#102846=CARTESIAN_POINT('Ctrl Pts',(-6.27564182199435,636.933990415857,
75.0030400468755));
#102847=CARTESIAN_POINT('Ctrl Pts',(-4.02089381669516,636.253138677506,
75.952258243854));
#102848=CARTESIAN_POINT('Ctrl Pts',(-3.23077935439454,636.064326910425,
76.195909276783));
#102849=CARTESIAN_POINT('Ctrl Pts',(-1.62216512710202,635.808561272943,
76.5196085118227));
#102850=CARTESIAN_POINT('Ctrl Pts',(-0.80351734247163,635.742307759052,
76.5994740882088));
#102851=CARTESIAN_POINT('Ctrl Pts',(0.803517342471631,635.742307759052,
76.5994740882088));
#102852=CARTESIAN_POINT('Ctrl Pts',(1.62216512710202,635.808561272943,76.5196085118227));
#102853=CARTESIAN_POINT('Ctrl Pts',(3.23077935439454,636.064326910425,76.195909276783));
#102854=CARTESIAN_POINT('Ctrl Pts',(4.02089381669516,636.253138677506,75.952258243854));
#102855=CARTESIAN_POINT('Ctrl Pts',(6.27564182199435,636.933990415857,75.0030400468755));
#102856=CARTESIAN_POINT('Ctrl Pts',(7.62604171070065,637.536810853389,74.0682591946972));
#102857=CARTESIAN_POINT('Ctrl Pts',(9.75980156458901,638.60355417627,71.9344993408089));
#102858=CARTESIAN_POINT('Ctrl Pts',(10.7006947361121,639.148581736175,70.5818572288996));
#102859=CARTESIAN_POINT('Ctrl Pts',(11.654095320228,639.721789350985,68.317292844778));
#102860=CARTESIAN_POINT('Ctrl Pts',(11.8983125166469,639.873458090211,67.5235508793709));
#102861=CARTESIAN_POINT('Ctrl Pts',(12.2213288811781,640.075308832797,65.9130515674887));
#102862=CARTESIAN_POINT('Ctrl Pts',(12.3,640.125373764374,65.0962538701053));
#102863=CARTESIAN_POINT('Ctrl Pts',(12.3,640.125373764374,63.5026943063123));
#102864=CARTESIAN_POINT('Ctrl Pts',(12.2213288811781,640.075308832797,62.6858966089289));
#102865=CARTESIAN_POINT('Ctrl Pts',(11.8983125166469,639.873458090211,61.0753972970467));
#102866=CARTESIAN_POINT('Ctrl Pts',(11.654095320228,639.721789350985,60.2816553316396));
#102867=CARTESIAN_POINT('Ctrl Pts',(10.7006947361121,639.148581736175,58.017090947518));
#102868=CARTESIAN_POINT('Ctrl Pts',(9.75980156458901,638.60355417627,56.6644488356087));
#102869=CARTESIAN_POINT('Ctrl Pts',(7.62604171070065,637.536810853389,54.5306889817204));
#102870=CARTESIAN_POINT('Ctrl Pts',(6.27564182199435,636.933990415857,53.5959081295421));
#102871=CARTESIAN_POINT('Ctrl Pts',(4.02089381669516,636.253138677506,52.6466899325635));
#102872=CARTESIAN_POINT('Ctrl Pts',(3.23077935439455,636.064326910425,52.4030388996346));
#102873=CARTESIAN_POINT('Ctrl Pts',(1.62216512710203,635.808561272943,52.0793396645949));
#102874=CARTESIAN_POINT('Ctrl Pts',(0.803517342471631,635.742307759052,
51.9994740882088));
#102875=CARTESIAN_POINT('Ctrl Pts',(-1.11022302462516E-15,635.742307759052,
51.9994740882088));
#102876=CARTESIAN_POINT('',(3.02331010654657E-11,637.214366842191,51.9994740882088));
#102877=CARTESIAN_POINT('',(-1.50631556295125E-15,22.7782939407039,51.9994740882088));
#102878=CARTESIAN_POINT('Ctrl Pts',(3.02331010654653E-11,637.214366842191,
51.9994740882088));
#102879=CARTESIAN_POINT('Ctrl Pts',(-0.830412355286513,637.21436684219,
51.9994740882068));
#102880=CARTESIAN_POINT('Ctrl Pts',(-1.64231938504929,637.2796645682,52.0826407378937));
#102881=CARTESIAN_POINT('Ctrl Pts',(-2.83515367978352,637.460650458936,
52.3238128901797));
#102882=CARTESIAN_POINT('Ctrl Pts',(-3.22987045737859,637.535077177222,
52.4241819097058));
#102883=CARTESIAN_POINT('Ctrl Pts',(-4.00546366489188,637.707452625756,
52.6628556650804));
#102884=CARTESIAN_POINT('Ctrl Pts',(-4.3819730375247,637.804289924468,52.7996457417074));
#102885=CARTESIAN_POINT('Ctrl Pts',(-5.11472586367998,638.014469814955,
53.106292277839));
#102886=CARTESIAN_POINT('Ctrl Pts',(-5.4709631470815,638.127820070073,53.2761570601927));
#102887=CARTESIAN_POINT('Ctrl Pts',(-6.16461781174502,638.366908005775,
53.648537824575));
#102888=CARTESIAN_POINT('Ctrl Pts',(-6.50301550229225,638.493045789728,
53.8517225300024));
#102889=CARTESIAN_POINT('Ctrl Pts',(-7.48440400047611,638.881866601756,
54.5069979081057));
#102890=CARTESIAN_POINT('Ctrl Pts',(-8.08540127787933,639.150990068374,
54.9978561404126));
#102891=CARTESIAN_POINT('Ctrl Pts',(-8.91512989825012,639.549152457839,
55.8164668699459));
#102892=CARTESIAN_POINT('Ctrl Pts',(-9.17960981986667,639.681011055625,
56.1031778705361));
#102893=CARTESIAN_POINT('Ctrl Pts',(-9.68420831857607,639.939946757686,
56.7060152336913));
#102894=CARTESIAN_POINT('Ctrl Pts',(-9.92291043223669,640.06632247763,57.0207475962688));
#102895=CARTESIAN_POINT('Ctrl Pts',(-10.588630748229,640.426678872799,57.9917849677541));
#102896=CARTESIAN_POINT('Ctrl Pts',(-10.9702548417394,640.644251182824,
58.6797638066909));
#102897=CARTESIAN_POINT('Ctrl Pts',(-11.4461458407818,640.921726794252,
59.7789482198191));
#102898=CARTESIAN_POINT('Ctrl Pts',(-11.5888532985381,641.006239015841,
60.157572983035));
#102899=CARTESIAN_POINT('Ctrl Pts',(-11.8381254652856,641.155207113641,
60.9355996838596));
#102900=CARTESIAN_POINT('Ctrl Pts',(-11.9427242536689,641.218473448575,
61.328594326499));
#102901=CARTESIAN_POINT('Ctrl Pts',(-12.1975694083928,641.373418861391,
62.5194580325877));
#102902=CARTESIAN_POINT('Ctrl Pts',(-12.2894856073328,641.430410984453,
63.329099770875));
#102903=CARTESIAN_POINT('Ctrl Pts',(-12.3039937693077,641.439358792849,
64.5687472338827));
#102904=CARTESIAN_POINT('Ctrl Pts',(-12.2877001556332,641.429290464151,
64.9861606719414));
#102905=CARTESIAN_POINT('Ctrl Pts',(-12.2143945388442,641.384192208162,
65.8053557663228));
#102906=CARTESIAN_POINT('Ctrl Pts',(-12.1575137190371,641.349243906771,
66.2102226898452));
#102907=CARTESIAN_POINT('Ctrl Pts',(-12.0043633846739,641.255863449383,
67.0108131994104));
#102908=CARTESIAN_POINT('Ctrl Pts',(-11.9080923355556,641.197427827018,
67.4065361653013));
#102909=CARTESIAN_POINT('Ctrl Pts',(-11.6759895729683,641.058111400096,
68.1889168908426));
#102910=CARTESIAN_POINT('Ctrl Pts',(-11.5401719162782,640.977255570532,
68.5745577010913));
#102911=CARTESIAN_POINT('Ctrl Pts',(-11.084049328587,640.709716701086,69.6921989559377));
#102912=CARTESIAN_POINT('Ctrl Pts',(-10.713120747878,640.496599747497,70.394448758527));
#102913=CARTESIAN_POINT('Ctrl Pts',(-10.0591458219439,640.13930168359,71.3889736072495));
#102914=CARTESIAN_POINT('Ctrl Pts',(-9.82548367484988,640.014353394576,
71.7091490640292));
#102915=CARTESIAN_POINT('Ctrl Pts',(-9.33415010122502,639.75928843652,72.3192655181552));
#102916=CARTESIAN_POINT('Ctrl Pts',(-9.07556749241562,639.628663169196,
72.6106271901288));
#102917=CARTESIAN_POINT('Ctrl Pts',(-8.53249912602467,639.364197433611,
73.167261290061));
#102918=CARTESIAN_POINT('Ctrl Pts',(-8.24801593829463,639.230348267547,
73.4325321421815));
#102919=CARTESIAN_POINT('Ctrl Pts',(-7.65202535438717,638.962573514797,
73.9373693102691));
#102920=CARTESIAN_POINT('Ctrl Pts',(-7.33917816046739,638.828145283974,
74.1777117225733));
#102921=CARTESIAN_POINT('Ctrl Pts',(-6.37510403592419,638.437326991065,
74.8474837516176));
#102922=CARTESIAN_POINT('Ctrl Pts',(-5.69483978905192,638.191200666448,
75.2303104565591));
#102923=CARTESIAN_POINT('Ctrl Pts',(-4.61072722039661,637.866819284235,
75.7094386141286));
#102924=CARTESIAN_POINT('Ctrl Pts',(-4.23864535083926,637.766213340969,
75.8531520209636));
#102925=CARTESIAN_POINT('Ctrl Pts',(-3.47047139791234,637.584888214298,
76.1066505694972));
#102926=CARTESIAN_POINT('Ctrl Pts',(-3.0763775345276,637.504868994145,76.2154608388605));
#102927=CARTESIAN_POINT('Ctrl Pts',(-1.88763310249882,637.307010047577,
76.4808614138365));
#102928=CARTESIAN_POINT('Ctrl Pts',(-1.07745358387097,637.229228985181,
76.5802724694516));
#102929=CARTESIAN_POINT('Ctrl Pts',(-0.247612686332903,637.216296403659,
76.5969814761947));
#102930=CARTESIAN_POINT('Origin',(-0.00103899059614113,643.228225309358,
59.690866538563));
#102931=CARTESIAN_POINT('Origin',(0.,22.7782939407039,64.2994740882088));
#102932=CARTESIAN_POINT('',(-1.09932974876048E-8,634.523606676254,48.5811983853019));
#102933=CARTESIAN_POINT('Ctrl Pts',(-1.91941230150446,634.6517886719,48.698800681464));
#102934=CARTESIAN_POINT('Ctrl Pts',(-1.77856148953381,634.63305573477,48.6814712512449));
#102935=CARTESIAN_POINT('Ctrl Pts',(-1.63703421268158,634.61630066659,48.6660258498621));
#102936=CARTESIAN_POINT('Ctrl Pts',(-1.49482298762889,634.601549979961,
48.6524629893774));
#102937=CARTESIAN_POINT('Ctrl Pts',(-1.47848330595685,634.599855166321,
48.65090465372));
#102938=CARTESIAN_POINT('Ctrl Pts',(-1.46213456918917,634.598186849375,
48.649371204989));
#102939=CARTESIAN_POINT('Ctrl Pts',(-1.44577674730117,634.596545097886,
48.6478626682891));
#102940=CARTESIAN_POINT('Ctrl Pts',(-1.30269956743721,634.582185168137,
48.634667930125));
#102941=CARTESIAN_POINT('Ctrl Pts',(-1.15892868452191,634.569854628533,
48.6233762927982));
#102942=CARTESIAN_POINT('Ctrl Pts',(-1.01444129744806,634.559620255549,
48.614023979145));
#102943=CARTESIAN_POINT('Ctrl Pts',(-0.998637300186558,634.558500822179,
48.6130010252225));
#102944=CARTESIAN_POINT('Ctrl Pts',(-0.982824721720789,634.557406504378,
48.6120013076365));
#102945=CARTESIAN_POINT('Ctrl Pts',(-0.967003526926908,634.556337417338,
48.6110248994056));
#102946=CARTESIAN_POINT('Ctrl Pts',(-0.806537717335257,634.545494246539,
48.6011217195698));
#102947=CARTESIAN_POINT('Ctrl Pts',(-0.645476066513774,634.537265715482,
48.5936338603989));
#102948=CARTESIAN_POINT('Ctrl Pts',(-0.484183920938914,634.531783080114,
48.588641220104));
#102949=CARTESIAN_POINT('Ctrl Pts',(-0.42261549034373,634.529690248787,
48.586735429674));
#102950=CARTESIAN_POINT('Ctrl Pts',(-0.361005641426023,634.527998080083,
48.58519312428));
#102951=CARTESIAN_POINT('Ctrl Pts',(-0.299397258432974,634.526706674014,
48.5840194145379));
#102952=CARTESIAN_POINT('Ctrl Pts',(-0.280307236559402,634.526306517917,
48.5836557279166));
#102953=CARTESIAN_POINT('Ctrl Pts',(-0.261214851172683,634.525944782025,
48.5833273536881));
#102954=CARTESIAN_POINT('Ctrl Pts',(-0.242121350637931,634.52562112443,
48.5830342121591));
#102955=CARTESIAN_POINT('Ctrl Pts',(-0.161408243682273,634.524252941048,
48.5817950279905));
#102956=CARTESIAN_POINT('Ctrl Pts',(-0.0806852921308739,634.523587621895,
48.5811855692694));
#102957=CARTESIAN_POINT('Ctrl Pts',(-1.56438910714485E-8,634.523606676253,
48.5811983853012));
#102958=CARTESIAN_POINT('',(-4.88526835490447E-16,632.874615496751,48.5811677441054));
#102959=CARTESIAN_POINT('',(-1.92493735523237E-15,22.7782939407039,48.5811677441054));
#102960=CARTESIAN_POINT('Ctrl Pts',(-4.88526835490447E-16,632.874615496751,
48.5811677441054));
#102961=CARTESIAN_POINT('Ctrl Pts',(-1.00038541833524,632.874615496751,
48.5811677441054));
#102962=CARTESIAN_POINT('Ctrl Pts',(-1.98186107540154,632.994943488914,
48.6756960232106));
#102963=CARTESIAN_POINT('Ctrl Pts',(-3.18805636841627,633.269464450547,
48.9059115645402));
#102964=CARTESIAN_POINT('Ctrl Pts',(-3.42854858272457,633.330642826548,
48.9577280742447));
#102965=CARTESIAN_POINT('Ctrl Pts',(-3.90080611161479,633.462396409217,
49.0709538770827));
#102966=CARTESIAN_POINT('Ctrl Pts',(-4.13345843873348,633.533150770153,
49.1325121211066));
#102967=CARTESIAN_POINT('Ctrl Pts',(-4.82191402968073,633.758076226497,
49.3314235132617));
#102968=CARTESIAN_POINT('Ctrl Pts',(-5.2682579819503,633.924846454147,49.4829579943546));
#102969=CARTESIAN_POINT('Ctrl Pts',(-6.13948585279376,634.283225661171,
49.8222366173663));
#102970=CARTESIAN_POINT('Ctrl Pts',(-6.56545659234337,634.475387114061,
50.0105449985554));
#102971=CARTESIAN_POINT('Ctrl Pts',(-7.39359379433367,634.875218035797,
50.4209480281591));
#102972=CARTESIAN_POINT('Ctrl Pts',(-7.79284032142571,635.081369451215,
50.6414529752954));
#102973=CARTESIAN_POINT('Ctrl Pts',(-8.95204291419481,635.709623472847,
51.3478306146848));
#102974=CARTESIAN_POINT('Ctrl Pts',(-9.6739937385886,636.141209625582,51.8780902826517));
#102975=CARTESIAN_POINT('Ctrl Pts',(-10.6909797044834,636.782704337244,
52.7681666459264));
#102976=CARTESIAN_POINT('Ctrl Pts',(-11.018834746685,636.99566173962,53.0807607042935));
#102977=CARTESIAN_POINT('Ctrl Pts',(-11.6523858512663,637.416398533235,
53.7403002029845));
#102978=CARTESIAN_POINT('Ctrl Pts',(-11.9552766171641,637.622331956755,
54.0845026139995));
#102979=CARTESIAN_POINT('Ctrl Pts',(-12.8157642528714,638.217349503897,
55.1530076404017));
#102980=CARTESIAN_POINT('Ctrl Pts',(-13.3290592983858,638.586009440671,
55.9162808887405));
#102981=CARTESIAN_POINT('Ctrl Pts',(-14.004746121757,639.080347468074,57.1474541420455));
#102982=CARTESIAN_POINT('Ctrl Pts',(-14.2141395881851,639.235335259904,
57.5723098240839));
#102983=CARTESIAN_POINT('Ctrl Pts',(-14.5988681163382,639.522324200276,
58.4540012253265));
#102984=CARTESIAN_POINT('Ctrl Pts',(-14.774314469106,639.654423764541,58.9121779826557));
#102985=CARTESIAN_POINT('Ctrl Pts',(-15.2329469259702,640.001641631537,
60.3025784912361));
#102986=CARTESIAN_POINT('Ctrl Pts',(-15.4543798168271,640.171936383211,
61.2611681259983));
#102987=CARTESIAN_POINT('Ctrl Pts',(-15.6499076381601,640.322525407937,
62.7513958204655));
#102988=CARTESIAN_POINT('Ctrl Pts',(-15.6916676668363,640.354793810631,
63.2567226635694));
#102989=CARTESIAN_POINT('Ctrl Pts',(-15.7262198238666,640.381486323066,
64.2573462892223));
#102990=CARTESIAN_POINT('Ctrl Pts',(-15.7195678789232,640.376339938052,
64.7561248933746));
#102991=CARTESIAN_POINT('Ctrl Pts',(-15.6590995589811,640.329648865433,
65.7506616225585));
#102992=CARTESIAN_POINT('Ctrl Pts',(-15.6052831790191,640.288103150951,
66.2464197156399));
#102993=CARTESIAN_POINT('Ctrl Pts',(-15.4498800061554,640.168587449424,
67.2348902714699));
#102994=CARTESIAN_POINT('Ctrl Pts',(-15.3482435235833,640.090585479368,
67.7257307925787));
#102995=CARTESIAN_POINT('Ctrl Pts',(-14.9812478047689,639.81051358526,69.1572522104259));
#102996=CARTESIAN_POINT('Ctrl Pts',(-14.6526793160863,639.561289321234,
70.0696014607015));
#102997=CARTESIAN_POINT('Ctrl Pts',(-13.8372960983329,638.955981993477,
71.8177596455625));
#102998=CARTESIAN_POINT('Ctrl Pts',(-13.3616578586644,638.608220356701,
72.6296038086576));
#102999=CARTESIAN_POINT('Ctrl Pts',(-12.2895634342419,637.849607134678,
74.1428267938299));
#103000=CARTESIAN_POINT('Ctrl Pts',(-11.6877930740782,637.435132345469,
74.8486713035806));
#103001=CARTESIAN_POINT('Ctrl Pts',(-10.3949373649157,636.588911121083,
76.1246737064291));
#103002=CARTESIAN_POINT('Ctrl Pts',(-9.70188800092167,636.155193164691,
76.6994753988773));
#103003=CARTESIAN_POINT('Ctrl Pts',(-8.58467388731213,635.511284076344,
77.4742190882293));
#103004=CARTESIAN_POINT('Ctrl Pts',(-8.19773601749983,635.297061722008,
77.7185803584321));
#103005=CARTESIAN_POINT('Ctrl Pts',(-7.40176600282271,634.879910318627,
78.1735199632814));
#103006=CARTESIAN_POINT('Ctrl Pts',(-6.99390219741844,634.677513014684,
78.3836222033658));
#103007=CARTESIAN_POINT('Ctrl Pts',(-5.73705816174996,634.097967889989,
78.9624303035972));
#103008=CARTESIAN_POINT('Ctrl Pts',(-4.8557807881079,633.747192826359,79.2806298462149));
#103009=CARTESIAN_POINT('Ctrl Pts',(-3.91253447320281,633.467807133627,
79.5230488432747));
#103010=CARTESIAN_POINT('Ctrl Pts',(3.93978362444746,633.475903764133,49.082928510463));
#103011=CARTESIAN_POINT('Ctrl Pts',(3.62591964374305,633.382350288002,49.0016645885587));
#103012=CARTESIAN_POINT('Ctrl Pts',(3.3057992406009,633.297177229342,48.9292260493855));
#103013=CARTESIAN_POINT('Ctrl Pts',(2.66144129984969,633.148794387986,48.8046503202028));
#103014=CARTESIAN_POINT('Ctrl Pts',(2.3359974548026,633.085210702006,48.7521822712622));
#103015=CARTESIAN_POINT('Ctrl Pts',(1.67806442767431,632.981730278595,48.6674791187011));
#103016=CARTESIAN_POINT('Ctrl Pts',(1.34557472886657,632.941837524538,48.6352427984729));
#103017=CARTESIAN_POINT('Ctrl Pts',(0.672995467599795,632.88812644915,48.5919666363597));
#103018=CARTESIAN_POINT('Ctrl Pts',(0.334567964264241,632.874615496751,
48.5811677441054));
#103019=CARTESIAN_POINT('Ctrl Pts',(-4.88526835490447E-16,632.874615496751,
48.5811677441054));
#103020=CARTESIAN_POINT('Ctrl Pts',(-6.34270402866122E-9,634.523606676255,
48.5811983853026));
#103021=CARTESIAN_POINT('Ctrl Pts',(0.131183067920692,634.523637656084,
48.5812192224713));
#103022=CARTESIAN_POINT('Ctrl Pts',(0.262263850660877,634.525477231112,
48.5828845405628));
#103023=CARTESIAN_POINT('Ctrl Pts',(0.393087042492144,634.529084138707,
48.5861654542112));
#103024=CARTESIAN_POINT('Ctrl Pts',(0.62595673992944,634.535504555978,48.5920055912538));
#103025=CARTESIAN_POINT('Ctrl Pts',(0.858266994437316,634.547536978571,
48.6029757350669));
#103026=CARTESIAN_POINT('Ctrl Pts',(1.08860828168253,634.564969308388,48.6189321330415));
#103027=CARTESIAN_POINT('Ctrl Pts',(1.16869635359341,634.571030408856,48.6244800622196));
#103028=CARTESIAN_POINT('Ctrl Pts',(1.24854641185876,634.577743962404,48.6306304686975));
#103029=CARTESIAN_POINT('Ctrl Pts',(1.32809942293835,634.585099981992,48.637376328015));
#103030=CARTESIAN_POINT('Ctrl Pts',(1.40535872090963,634.592243909061,48.6439276872661));
#103031=CARTESIAN_POINT('Ctrl Pts',(1.48241468364269,634.599987046874,48.6510297053401));
#103032=CARTESIAN_POINT('Ctrl Pts',(1.55926269747949,634.608315807309,48.6586783314213));
#103033=CARTESIAN_POINT('Ctrl Pts',(2.07067858640156,634.66374287964,48.7095791772737));
#103034=CARTESIAN_POINT('Ctrl Pts',(2.57353940461454,634.745183949427,48.7847527919497));
#103035=CARTESIAN_POINT('Ctrl Pts',(3.0686126658422,634.848983739582,48.8833382201712));
#103036=CARTESIAN_POINT('Ctrl Pts',(3.5280360180697,634.945308973214,48.9748245747402));
#103037=CARTESIAN_POINT('Ctrl Pts',(3.98077413585814,635.060900537147,49.0864791016381));
#103038=CARTESIAN_POINT('Ctrl Pts',(4.42735940791138,635.192792800213,49.2175762302821));
#103039=CARTESIAN_POINT('Ctrl Pts',(4.46201311942238,635.203027254237,49.2277489842));
#103040=CARTESIAN_POINT('Ctrl Pts',(4.49663613259052,635.213362895059,49.2380436267645));
#103041=CARTESIAN_POINT('Ctrl Pts',(4.53121896438336,635.223794826727,49.2484565026335));
#103042=CARTESIAN_POINT('Ctrl Pts',(4.74601947947587,635.288589529171,49.3131328459027));
#103043=CARTESIAN_POINT('Ctrl Pts',(4.95932213084446,635.357118326411,49.3823865525656));
#103044=CARTESIAN_POINT('Ctrl Pts',(5.16884411272974,635.428209929197,49.4553437713038));
#103045=CARTESIAN_POINT('Ctrl Pts',(5.41200740793916,635.510716157134,49.5400151626208));
#103046=CARTESIAN_POINT('Ctrl Pts',(5.65093526308688,635.596907367806,49.6299024007825));
#103047=CARTESIAN_POINT('Ctrl Pts',(5.88596567871249,635.68616027303,49.7248192945151));
#103048=CARTESIAN_POINT('Ctrl Pts',(5.9012058732883,635.691947743721,49.7309740380412));
#103049=CARTESIAN_POINT('Ctrl Pts',(5.91642974293561,635.697748021797,49.7371498648016));
#103050=CARTESIAN_POINT('Ctrl Pts',(5.93163735194624,635.703560967641,49.7433467521698));
#103051=CARTESIAN_POINT('Ctrl Pts',(6.38532277407427,635.876977366458,49.9282171982447));
#103052=CARTESIAN_POINT('Ctrl Pts',(6.82458941528542,636.061682510158,50.1318546390623));
#103053=CARTESIAN_POINT('Ctrl Pts',(7.25129724309772,636.254031066571,50.3537276895692));
#103054=CARTESIAN_POINT('Ctrl Pts',(7.67449000072657,636.444795122697,50.5737730273099));
#103055=CARTESIAN_POINT('Ctrl Pts',(8.08531522162718,636.643099353163,50.8117642540156));
#103056=CARTESIAN_POINT('Ctrl Pts',(8.48485213004565,636.846125285092,51.0679794092165));
#103057=CARTESIAN_POINT('Ctrl Pts',(8.50152150271618,636.854595879047,51.0786691498034));
#103058=CARTESIAN_POINT('Ctrl Pts',(8.51817133864072,636.863074757022,51.0893906828856));
#103059=CARTESIAN_POINT('Ctrl Pts',(8.53480170293738,636.871561707065,51.1001440211828));
#103060=CARTESIAN_POINT('Ctrl Pts',(8.88265589543402,637.04908163995,51.3250695696129));
#103061=CARTESIAN_POINT('Ctrl Pts',(9.22310591847262,637.230801572943,51.5648853840179));
#103062=CARTESIAN_POINT('Ctrl Pts',(9.55213627069025,637.412648744007,51.8166263298771));
#103063=CARTESIAN_POINT('Ctrl Pts',(9.58597325050769,637.431349629854,51.8425149849719));
#103064=CARTESIAN_POINT('Ctrl Pts',(9.61968948712715,637.45005185641,51.8685297223147));
#103065=CARTESIAN_POINT('Ctrl Pts',(9.65328063531741,637.468750993354,51.8946672948334));
#103066=CARTESIAN_POINT('Ctrl Pts',(9.68287665471881,637.485226167606,51.917696221948));
#103067=CARTESIAN_POINT('Ctrl Pts',(9.71237647083123,637.501699898547,51.940821203202));
#103068=CARTESIAN_POINT('Ctrl Pts',(9.74177715342259,637.518169132975,51.9640400780151));
#103069=CARTESIAN_POINT('Ctrl Pts',(10.0857430188191,637.710846784418,52.2356834435658));
#103070=CARTESIAN_POINT('Ctrl Pts',(10.4168996980707,637.903110177124,52.5202505899506));
#103071=CARTESIAN_POINT('Ctrl Pts',(10.7356021263374,638.093325829708,52.8182111751762));
#103072=CARTESIAN_POINT('Ctrl Pts',(11.1345671134278,638.331445714109,53.1912106583761));
#103073=CARTESIAN_POINT('Ctrl Pts',(11.5140262355694,638.566425706844,53.5852075140256));
#103074=CARTESIAN_POINT('Ctrl Pts',(11.8747642121883,638.795350794663,54.0011669855164));
#103075=CARTESIAN_POINT('Ctrl Pts',(12.1396201387599,638.963428929431,54.3065668557228));
#103076=CARTESIAN_POINT('Ctrl Pts',(12.3942600538462,639.128288972181,54.6238994674662));
#103077=CARTESIAN_POINT('Ctrl Pts',(12.6384027128533,639.288833991502,54.9540941874028));
#103078=CARTESIAN_POINT('Ctrl Pts',(12.6934199989364,639.325012639237,55.0285032130264));
#103079=CARTESIAN_POINT('Ctrl Pts',(12.7479128130092,639.360977370941,55.1035770627711));
#103080=CARTESIAN_POINT('Ctrl Pts',(12.8018733060316,639.396712358839,55.1793208996343));
#103081=CARTESIAN_POINT('Ctrl Pts',(12.9672617185343,639.506239766544,55.4114750597241));
#103082=CARTESIAN_POINT('Ctrl Pts',(13.1265971638525,639.61291400292,55.6485181832674));
#103083=CARTESIAN_POINT('Ctrl Pts',(13.2794577936759,639.71615893547,55.8898965897075));
#103084=CARTESIAN_POINT('Ctrl Pts',(13.3380989021436,639.755766238511,55.9824953009005));
#103085=CARTESIAN_POINT('Ctrl Pts',(13.395787529721,639.794869067689,56.0757317394399));
#103086=CARTESIAN_POINT('Ctrl Pts',(13.4525014240595,639.83343577007,56.1695736395204));
#103087=CARTESIAN_POINT('Ctrl Pts',(13.5103276838369,639.87275890555,56.265256120072));
#103088=CARTESIAN_POINT('Ctrl Pts',(13.5671707966639,639.911546279781,56.3616179364094));
#103089=CARTESIAN_POINT('Ctrl Pts',(13.6230077720489,639.949765308903,56.4586314313637));
#103090=CARTESIAN_POINT('Ctrl Pts',(13.7869220361162,640.061960569997,56.7434229251792));
#103091=CARTESIAN_POINT('Ctrl Pts',(13.9424991854698,640.169458563498,57.0341146385251));
#103092=CARTESIAN_POINT('Ctrl Pts',(14.0893519141752,640.271692823618,57.3308706562064));
#103093=CARTESIAN_POINT('Ctrl Pts',(14.111156236253,640.286872308227,57.3749322398425));
#103094=CARTESIAN_POINT('Ctrl Pts',(14.1327682926389,640.301935791542,57.4191274656104));
#103095=CARTESIAN_POINT('Ctrl Pts',(14.1541868887825,640.31688146356,57.4634568184052));
#103096=CARTESIAN_POINT('Ctrl Pts',(14.3690003859214,640.46677607158,57.9080491360309));
#103097=CARTESIAN_POINT('Ctrl Pts',(14.5644206321617,640.604866455008,58.3662732287448));
#103098=CARTESIAN_POINT('Ctrl Pts',(14.7394736989775,640.729507918388,58.8391490276349));
#103099=CARTESIAN_POINT('Ctrl Pts',(14.7930222736766,640.767635629223,58.9838013065174));
#103100=CARTESIAN_POINT('Ctrl Pts',(14.844665954123,640.804501637939,59.1298267006041));
#103101=CARTESIAN_POINT('Ctrl Pts',(14.8943779224113,640.840060847293,59.2772573842497));
#103102=CARTESIAN_POINT('Ctrl Pts',(14.9788181415358,640.900461341042,59.5276815710471));
#103103=CARTESIAN_POINT('Ctrl Pts',(15.0576110594056,640.957060717116,59.7824113765591));
#103104=CARTESIAN_POINT('Ctrl Pts',(15.1295263785222,641.008879049081,60.0377155440764));
#103105=CARTESIAN_POINT('Ctrl Pts',(15.1536787692919,641.026281969877,60.1234581382101));
#103106=CARTESIAN_POINT('Ctrl Pts',(15.1770912859024,641.043171234754,60.2093651695768));
#103107=CARTESIAN_POINT('Ctrl Pts',(15.1997652434983,641.059544776398,60.2954371488871));
#103108=CARTESIAN_POINT('Ctrl Pts',(15.2446133607517,641.091930940674,60.4656838384653));
#103109=CARTESIAN_POINT('Ctrl Pts',(15.2865717155591,641.122296729638,60.636574808298));
#103110=CARTESIAN_POINT('Ctrl Pts',(15.325649598072,641.150623333856,60.8081106404716));
#103111=CARTESIAN_POINT('Ctrl Pts',(15.4433396652835,641.235933994003,61.3247216316376));
#103112=CARTESIAN_POINT('Ctrl Pts',(15.5349555636936,641.302769846919,61.8471715921895));
#103113=CARTESIAN_POINT('Ctrl Pts',(15.600123128367,641.350389654829,62.3755944903987));
#103114=CARTESIAN_POINT('Ctrl Pts',(15.6386979344604,641.378577371611,62.688385231251));
#103115=CARTESIAN_POINT('Ctrl Pts',(15.6680084809615,641.400034585006,63.00326810169));
#103116=CARTESIAN_POINT('Ctrl Pts',(15.6877925284557,641.414528796385,63.3203069204358));
#103117=CARTESIAN_POINT('Ctrl Pts',(15.7005815679481,641.423898317046,63.525250927709));
#103118=CARTESIAN_POINT('Ctrl Pts',(15.7093924335219,641.430360162221,63.7311946738769));
#103119=CARTESIAN_POINT('Ctrl Pts',(15.7141470311169,641.433849188663,63.9378910948812));
#103120=CARTESIAN_POINT('Ctrl Pts',(15.7144659003347,641.434083181785,63.9517532829566));
#103121=CARTESIAN_POINT('Ctrl Pts',(15.7147665408602,641.434303815199,63.9656188529755));
#103122=CARTESIAN_POINT('Ctrl Pts',(15.7150489358492,641.434511074186,63.9794877289295));
#103123=CARTESIAN_POINT('Ctrl Pts',(15.7158488065306,641.435098125634,64.0187706754704));
#103124=CARTESIAN_POINT('Ctrl Pts',(15.7165007988266,641.435576865089,64.0581033421356));
#103125=CARTESIAN_POINT('Ctrl Pts',(15.7170049051664,641.435947313476,64.0974701301083));
#103126=CARTESIAN_POINT('Ctrl Pts',(15.7194694294045,641.437758397678,64.2899303224724));
#103127=CARTESIAN_POINT('Ctrl Pts',(15.7184018336159,641.436970322652,64.4836683248673));
#103128=CARTESIAN_POINT('Ctrl Pts',(15.7137735336007,641.433574471331,64.6767950132201));
#103129=CARTESIAN_POINT('Ctrl Pts',(15.7128333947127,641.432884677698,64.7160245163702));
#103130=CARTESIAN_POINT('Ctrl Pts',(15.7117464743582,641.432087384869,64.7552287682019));
#103131=CARTESIAN_POINT('Ctrl Pts',(15.7105127430939,641.431182674632,64.7943919360785));
#103132=CARTESIAN_POINT('Ctrl Pts',(15.7095991882977,641.430512753718,64.8233915252814));
#103133=CARTESIAN_POINT('Ctrl Pts',(15.708605979292,641.429784554329,64.8523701843884));
#103134=CARTESIAN_POINT('Ctrl Pts',(15.7075334205578,641.42899836347,64.8813270198615));
#103135=CARTESIAN_POINT('Ctrl Pts',(15.6985693797753,641.422427677226,65.1233373134135));
#103136=CARTESIAN_POINT('Ctrl Pts',(15.6840546075089,641.411790509973,65.3640472137197));
#103137=CARTESIAN_POINT('Ctrl Pts',(15.6641212610662,641.397197896467,65.6034907467274));
#103138=CARTESIAN_POINT('Ctrl Pts',(15.6411292069346,641.380366093507,65.8796761172173));
#103139=CARTESIAN_POINT('Ctrl Pts',(15.6110000935115,641.3583004588,66.1541909485691));
#103140=CARTESIAN_POINT('Ctrl Pts',(15.5737798644399,641.331104474615,66.4270558219922));
#103141=CARTESIAN_POINT('Ctrl Pts',(15.5042909343416,641.280330476413,66.9364854678731));
#103142=CARTESIAN_POINT('Ctrl Pts',(15.4100832406381,641.211672672658,67.4401695893287));
#103143=CARTESIAN_POINT('Ctrl Pts',(15.2914680739336,641.12581412946,67.9381923855767));
#103144=CARTESIAN_POINT('Ctrl Pts',(15.2270223963164,641.079165693603,68.2087768096833));
#103145=CARTESIAN_POINT('Ctrl Pts',(15.1553484481903,641.027422827044,68.4777850319379));
#103146=CARTESIAN_POINT('Ctrl Pts',(15.0765013223764,640.970699140689,68.7451756305374));
#103147=CARTESIAN_POINT('Ctrl Pts',(15.0102267686864,640.923020332387,68.969929448767));
#103148=CARTESIAN_POINT('Ctrl Pts',(14.9393986310139,640.872195863483,69.1917973879912));
#103149=CARTESIAN_POINT('Ctrl Pts',(14.8641408406389,640.818399206912,69.4108007082289));
#103150=CARTESIAN_POINT('Ctrl Pts',(14.638491776709,640.657098095927,70.0674489298011));
#103151=CARTESIAN_POINT('Ctrl Pts',(14.3730295175424,640.469084278575,70.6983179950207));
#103152=CARTESIAN_POINT('Ctrl Pts',(14.0709202550478,640.258910548728,71.3048669690282));
#103153=CARTESIAN_POINT('Ctrl Pts',(14.0153823305951,640.220273491944,71.4163712334691));
#103154=CARTESIAN_POINT('Ctrl Pts',(13.9586060318041,640.18088759514,71.5270536792873));
#103155=CARTESIAN_POINT('Ctrl Pts',(13.9006111685527,640.14078120424,71.6369234719542));
#103156=CARTESIAN_POINT('Ctrl Pts',(13.8132963508808,640.080398577011,71.8023391721822));
#103157=CARTESIAN_POINT('Ctrl Pts',(13.722999297798,640.018241840122,71.9661929969353));
#103158=CARTESIAN_POINT('Ctrl Pts',(13.6299592468021,639.954544488634,72.1281591912608));
#103159=CARTESIAN_POINT('Ctrl Pts',(13.5153701108086,639.876094139629,72.3276385130071));
#103160=CARTESIAN_POINT('Ctrl Pts',(13.3964238457193,639.795161400824,72.5245885124587));
#103161=CARTESIAN_POINT('Ctrl Pts',(13.2736785048361,639.712270183463,72.7181535822366));
#103162=CARTESIAN_POINT('Ctrl Pts',(13.2230467223056,639.678078009153,72.797998116033));
#103163=CARTESIAN_POINT('Ctrl Pts',(13.1717690142433,639.643552886662,72.8772669587132));
#103164=CARTESIAN_POINT('Ctrl Pts',(13.119886458028,639.608732640406,72.9559013911626));
#103165=CARTESIAN_POINT('Ctrl Pts',(13.028077430013,639.547116305414,73.0950493310163));
#103166=CARTESIAN_POINT('Ctrl Pts',(12.9344479627768,639.48462216792,73.232156163104));
#103167=CARTESIAN_POINT('Ctrl Pts',(12.8390792114001,639.421364130704,73.367197238578));
#103168=CARTESIAN_POINT('Ctrl Pts',(12.6440223006845,639.291982995488,73.643395622445));
#103169=CARTESIAN_POINT('Ctrl Pts',(12.4414058536515,639.15920090843,73.9113615973352));
#103170=CARTESIAN_POINT('Ctrl Pts',(12.2313971791556,639.023622204506,74.1715598542876));
#103171=CARTESIAN_POINT('Ctrl Pts',(12.1400319511015,638.964638073335,74.2847602882354));
#103172=CARTESIAN_POINT('Ctrl Pts',(12.0472674516941,638.90512335526,74.3964896998921));
#103173=CARTESIAN_POINT('Ctrl Pts',(11.9530990206169,638.845127013667,74.506770281284));
#103174=CARTESIAN_POINT('Ctrl Pts',(11.7624766227016,638.723678175987,74.7300080333411));
#103175=CARTESIAN_POINT('Ctrl Pts',(11.5660389794382,638.600215282207,74.9473754835452));
#103176=CARTESIAN_POINT('Ctrl Pts',(11.3639002899801,638.475242595692,75.1588940699884));
#103177=CARTESIAN_POINT('Ctrl Pts',(11.324185565883,638.450688880725,75.2004516873081));
#103178=CARTESIAN_POINT('Ctrl Pts',(11.2842508843236,638.42607691691,75.2417836420707));
#103179=CARTESIAN_POINT('Ctrl Pts',(11.244097275529,638.401410569611,75.2828902591882));
#103180=CARTESIAN_POINT('Ctrl Pts',(11.1555970541534,638.347044915761,75.373490950486));
#103181=CARTESIAN_POINT('Ctrl Pts',(11.0659447322039,638.292363220271,75.463070243372));
#103182=CARTESIAN_POINT('Ctrl Pts',(10.9752166475745,638.237454616551,75.5515588294561));
#103183=CARTESIAN_POINT('Ctrl Pts',(10.7995114119609,638.131117872056,75.722927021902));
#103184=CARTESIAN_POINT('Ctrl Pts',(10.6193973010404,638.023696042729,75.8905643475752));
#103185=CARTESIAN_POINT('Ctrl Pts',(10.4355011010581,637.915901197236,76.053840239258));
#103186=CARTESIAN_POINT('Ctrl Pts',(10.343703427894,637.862091950518,76.1353446256548));
#103187=CARTESIAN_POINT('Ctrl Pts',(10.2509639608639,637.808189937796,76.2157627203798));
#103188=CARTESIAN_POINT('Ctrl Pts',(10.1573640686073,637.75428427382,76.2950194899588));
#103189=CARTESIAN_POINT('Ctrl Pts',(10.0741297969102,637.706348335293,76.3654990528508));
#103190=CARTESIAN_POINT('Ctrl Pts',(9.99030988510562,637.658450897748,76.4350092280443));
#103191=CARTESIAN_POINT('Ctrl Pts',(9.90591360420892,637.610632366472,76.5035433110902));
#103192=CARTESIAN_POINT('Ctrl Pts',(9.40639551616552,637.327607794034,76.9091774665904));
#103193=CARTESIAN_POINT('Ctrl Pts',(8.88565058254247,637.046582516874,77.2814637959477));
#103194=CARTESIAN_POINT('Ctrl Pts',(8.34163289752633,636.773710266685,77.6218868333786));
#103195=CARTESIAN_POINT('Ctrl Pts',(8.14290238226259,636.674029604871,77.7462439039291));
#103196=CARTESIAN_POINT('Ctrl Pts',(7.94106647131428,636.57543655124,77.8663491091254));
#103197=CARTESIAN_POINT('Ctrl Pts',(7.73602658782707,636.478229722697,77.982275225029));
#103198=CARTESIAN_POINT('Ctrl Pts',(7.67213350385392,636.447938815615,78.0183993045599));
#103199=CARTESIAN_POINT('Ctrl Pts',(7.60792574479906,636.41778470578,78.0541135135407));
#103200=CARTESIAN_POINT('Ctrl Pts',(7.54339610210034,636.387779954009,78.0894159789354));
#103201=CARTESIAN_POINT('Ctrl Pts',(7.29105366480304,636.270446711865,78.227465870237));
#103202=CARTESIAN_POINT('Ctrl Pts',(7.03370074020654,636.155345245241,78.3592633253105));
#103203=CARTESIAN_POINT('Ctrl Pts',(6.77108651634947,636.043300256403,78.4846057105662));
#103204=CARTESIAN_POINT('Ctrl Pts',(6.64811138529507,635.99083262162,78.5433001560806));
#103205=CARTESIAN_POINT('Ctrl Pts',(6.52398298358298,635.93903498938,78.6005796581726));
#103206=CARTESIAN_POINT('Ctrl Pts',(6.39867799322467,635.887990551571,78.6564262110446));
#103207=CARTESIAN_POINT('Ctrl Pts',(6.3469937399708,635.866936372936,78.6794611067318));
#103208=CARTESIAN_POINT('Ctrl Pts',(6.29507802198154,635.846001728375,78.7022602318609));
#103209=CARTESIAN_POINT('Ctrl Pts',(6.242947083485,635.825199921756,78.7248152334023));
#103210=CARTESIAN_POINT('Ctrl Pts',(5.9934113591813,635.725627690158,78.8327795020041));
#103211=CARTESIAN_POINT('Ctrl Pts',(5.73853110387259,635.628941916558,78.9353252138458));
#103212=CARTESIAN_POINT('Ctrl Pts',(5.48010053989362,635.53663991684,79.0314825681284));
#103213=CARTESIAN_POINT('Ctrl Pts',(5.31038406678866,635.476023364326,79.0946310083929));
#103214=CARTESIAN_POINT('Ctrl Pts',(5.13913733643898,635.417297288755,79.1550248358553));
#103215=CARTESIAN_POINT('Ctrl Pts',(4.96687438959262,635.360879771099,79.2123984530303));
#103216=CARTESIAN_POINT('Ctrl Pts',(4.93007196624935,635.348826677809,79.2246558083506));
#103217=CARTESIAN_POINT('Ctrl Pts',(4.89321390536558,635.336873120223,79.2367829629027));
#103218=CARTESIAN_POINT('Ctrl Pts',(4.85630009928058,635.325021373308,79.2487791179174));
#103219=CARTESIAN_POINT('Ctrl Pts',(4.25499476163656,635.131963018284,79.4441898004406));
#103220=CARTESIAN_POINT('Ctrl Pts',(3.63825269208279,634.965644185472,79.605049820634));
#103221=CARTESIAN_POINT('Ctrl Pts',(3.00303825703234,634.835251784121,79.7285331850169));
#103222=CARTESIAN_POINT('Ctrl Pts',(2.63932772572501,634.760591815839,79.799237182894));
#103223=CARTESIAN_POINT('Ctrl Pts',(2.26956149096814,634.697709328596,79.8576872889952));
#103224=CARTESIAN_POINT('Ctrl Pts',(1.89317385967765,634.648322422428,79.9033533194805));
#103225=CARTESIAN_POINT('Ctrl Pts',(-29.2194381818547,646.39670912511,64.2994740882088));
#103226=CARTESIAN_POINT('Ctrl Pts',(-30.058537813032,646.39670912511,64.2994740882088));
#103227=CARTESIAN_POINT('Ctrl Pts',(-30.204245934867,645.570357302777,64.2994740882088));
#103228=CARTESIAN_POINT('Ctrl Pts',(-29.2194381818525,646.39670912511,63.6657417300129));
#103229=CARTESIAN_POINT('Ctrl Pts',(-30.058537813076,646.39670912511,63.5542259178429));
#103230=CARTESIAN_POINT('Ctrl Pts',(-30.2042459348789,645.570357302709,
63.5348184358982));
#103231=CARTESIAN_POINT('Ctrl Pts',(-29.0915097686744,646.39670912511,63.0324871423586));
#103232=CARTESIAN_POINT('Ctrl Pts',(-29.9111456379662,646.39670912511,62.8068138256533));
#103233=CARTESIAN_POINT('Ctrl Pts',(-30.0506856115286,645.565837705453,
62.7707392571429));
#103234=CARTESIAN_POINT('Ctrl Pts',(-28.5990783166314,646.39670912511,61.8617135225403));
#103235=CARTESIAN_POINT('Ctrl Pts',(-29.3454369712421,646.39670912511,61.4226444395839));
#103236=CARTESIAN_POINT('Ctrl Pts',(-29.45958992671,645.548440539176,61.3580945430258));
#103237=CARTESIAN_POINT('Ctrl Pts',(-28.234769018359,646.39670912511,61.3247693565845));
#103238=CARTESIAN_POINT('Ctrl Pts',(-28.9235388845874,646.39670912511,60.7826106946149));
#103239=CARTESIAN_POINT('Ctrl Pts',(-29.0222871239381,645.535569814948,
60.7102226359645));
#103240=CARTESIAN_POINT('Ctrl Pts',(-27.3248743388726,646.39670912511,60.4286980218046));
#103241=CARTESIAN_POINT('Ctrl Pts',(-27.8689763870026,646.39670912511,59.7035779132664));
#103242=CARTESIAN_POINT('Ctrl Pts',(-27.9300847139336,645.50342404321,59.6290311800515));
#103243=CARTESIAN_POINT('Ctrl Pts',(-26.7796469437582,646.39670912511,60.0699234004071));
#103244=CARTESIAN_POINT('Ctrl Pts',(-27.2309350653715,646.39670912511,59.2646547208034));
#103245=CARTESIAN_POINT('Ctrl Pts',(-27.275614819367,645.484161643149,59.1961370117062));
#103246=CARTESIAN_POINT('Ctrl Pts',(-25.590812253516,646.39670912511,59.584973088534));
#103247=CARTESIAN_POINT('Ctrl Pts',(-25.8325282144725,646.39670912511,58.6515832061606));
#103248=CARTESIAN_POINT('Ctrl Pts',(-25.8485836001921,645.442161168378,
58.6110004122124));
#103249=CARTESIAN_POINT('Ctrl Pts',(-24.9476726899769,646.39670912511,59.4589881954405));
#103250=CARTESIAN_POINT('Ctrl Pts',(-25.0679049368893,646.39670912511,58.4814632535357));
#103251=CARTESIAN_POINT('Ctrl Pts',(-25.0765837225069,645.419439618224,
58.4589881954405));
#103252=CARTESIAN_POINT('Ctrl Pts',(-23.6608872937837,646.39670912511,59.4589881954405));
#103253=CARTESIAN_POINT('Ctrl Pts',(-23.5230979344025,646.39670912511,58.4359963952912));
#103254=CARTESIAN_POINT('Ctrl Pts',(-23.5319762612537,645.373978631996,
58.4589881954405));
#103255=CARTESIAN_POINT('Ctrl Pts',(-23.0177477302446,646.39670912511,59.584973088534));
#103256=CARTESIAN_POINT('Ctrl Pts',(-22.7425774139614,646.39670912511,58.566978825107));
#103257=CARTESIAN_POINT('Ctrl Pts',(-22.7599763835685,645.351257081842,
58.6110004122124));
#103258=CARTESIAN_POINT('Ctrl Pts',(-21.8289130400024,646.39670912511,60.0699234004071));
#103259=CARTESIAN_POINT('Ctrl Pts',(-21.280243410082,646.39670912511,59.1147920019372));
#103260=CARTESIAN_POINT('Ctrl Pts',(-21.3329451643936,645.309256607071,
59.1961370117062));
#103261=CARTESIAN_POINT('Ctrl Pts',(-21.2836856448871,646.39670912511,60.4286980218043));
#103262=CARTESIAN_POINT('Ctrl Pts',(-20.6031006941262,646.39670912511,59.5367585763147));
#103263=CARTESIAN_POINT('Ctrl Pts',(-20.6784752698267,645.28999420701,59.6290311800517));
#103264=CARTESIAN_POINT('Ctrl Pts',(-20.3737909654025,646.39670912511,61.3247693565847));
#103265=CARTESIAN_POINT('Ctrl Pts',(-19.4561930076906,646.39670912511,60.6144134200796));
#103266=CARTESIAN_POINT('Ctrl Pts',(-19.5862728598228,645.257848435272,
60.7102226359643));
#103267=CARTESIAN_POINT('Ctrl Pts',(-20.0094816671295,646.39670912511,61.8617135225397));
#103268=CARTESIAN_POINT('Ctrl Pts',(-18.9941367827483,646.39670912511,61.2703174980295));
#103269=CARTESIAN_POINT('Ctrl Pts',(-19.1489700570509,645.244977711044,
61.358094543025));
#103270=CARTESIAN_POINT('Ctrl Pts',(-19.517050215086,646.39670912511,63.0324871423592));
#103271=CARTESIAN_POINT('Ctrl Pts',(-18.3617148294141,646.39670912511,62.7197742154602));
#103272=CARTESIAN_POINT('Ctrl Pts',(-18.5578743722317,645.227580544767,
62.7707392571437));
#103273=CARTESIAN_POINT('Ctrl Pts',(-19.3891218019081,646.39670912511,63.6657417300125));
#103274=CARTESIAN_POINT('Ctrl Pts',(-18.1973682094106,646.39670912511,63.5071737129916));
#103275=CARTESIAN_POINT('Ctrl Pts',(-18.4043140488817,645.223060947511,
63.5348184358976));
#103276=CARTESIAN_POINT('Ctrl Pts',(-19.3891218019059,646.39670912511,64.2994740882088));
#103277=CARTESIAN_POINT('Ctrl Pts',(-18.1973682093116,646.39670912511,64.2994740882088));
#103278=CARTESIAN_POINT('Ctrl Pts',(-18.4043140488937,645.223060947443,
64.2994740882088));
#103279=CARTESIAN_POINT('',(-19.3891218019059,646.39670912511,64.2994740882088));
#103280=CARTESIAN_POINT('',(-29.2194381818547,646.39670912511,64.2994740882088));
#103281=CARTESIAN_POINT('Ctrl Pts',(-19.3891218019059,646.39670912511,64.2994740882088));
#103282=CARTESIAN_POINT('Ctrl Pts',(-19.3891218019081,646.39670912511,63.6657417300125));
#103283=CARTESIAN_POINT('Ctrl Pts',(-19.517050215086,646.39670912511,63.0324871423592));
#103284=CARTESIAN_POINT('Ctrl Pts',(-19.7632659411077,646.39670912511,62.4471003324495));
#103285=CARTESIAN_POINT('Ctrl Pts',(-20.0094816671295,646.39670912511,61.8617135225397));
#103286=CARTESIAN_POINT('Ctrl Pts',(-20.3737909654025,646.39670912511,61.3247693565847));
#103287=CARTESIAN_POINT('Ctrl Pts',(-20.8287383051448,646.39670912511,60.8767336891945));
#103288=CARTESIAN_POINT('Ctrl Pts',(-21.2836856448871,646.39670912511,60.4286980218043));
#103289=CARTESIAN_POINT('Ctrl Pts',(-21.8289130400025,646.39670912511,60.0699234004071));
#103290=CARTESIAN_POINT('Ctrl Pts',(-22.4233303851235,646.39670912511,59.8274482444706));
#103291=CARTESIAN_POINT('Ctrl Pts',(-23.0177477302446,646.39670912511,59.584973088534));
#103292=CARTESIAN_POINT('Ctrl Pts',(-23.6608872937837,646.39670912511,59.4589881954405));
#103293=CARTESIAN_POINT('Ctrl Pts',(-24.3042799918803,646.39670912511,59.4589881954405));
#103294=CARTESIAN_POINT('Ctrl Pts',(-24.9476726899769,646.39670912511,59.4589881954405));
#103295=CARTESIAN_POINT('Ctrl Pts',(-25.590812253516,646.39670912511,59.584973088534));
#103296=CARTESIAN_POINT('Ctrl Pts',(-26.1852295986371,646.39670912511,59.8274482444706));
#103297=CARTESIAN_POINT('Ctrl Pts',(-26.7796469437582,646.39670912511,60.0699234004071));
#103298=CARTESIAN_POINT('Ctrl Pts',(-27.3248743388726,646.39670912511,60.4286980218046));
#103299=CARTESIAN_POINT('Ctrl Pts',(-27.7798216786158,646.39670912511,60.8767336891945));
#103300=CARTESIAN_POINT('Ctrl Pts',(-28.234769018359,646.39670912511,61.3247693565845));
#103301=CARTESIAN_POINT('Ctrl Pts',(-28.5990783166314,646.39670912511,61.8617135225403));
#103302=CARTESIAN_POINT('Ctrl Pts',(-28.8452940426529,646.39670912511,62.4471003324495));
#103303=CARTESIAN_POINT('Ctrl Pts',(-29.0915097686744,646.39670912511,63.0324871423586));
#103304=CARTESIAN_POINT('Ctrl Pts',(-29.2194381818525,646.39670912511,63.6657417300129));
#103305=CARTESIAN_POINT('Ctrl Pts',(-29.2194381818548,646.39670912511,64.2994740882088));
#103306=CARTESIAN_POINT('',(-18.4043140488937,645.223060947443,64.2994740882088));
#103307=CARTESIAN_POINT('Origin',(-19.3891218019059,645.39670912511,64.2994740882088));
#103308=CARTESIAN_POINT('',(-30.204245934867,645.570357302777,64.2994740882088));
#103309=CARTESIAN_POINT('Ctrl Pts',(-30.204245934867,645.570357302777,64.2994740882088));
#103310=CARTESIAN_POINT('Ctrl Pts',(-30.2042459348789,645.570357302709,
63.5348184358982));
#103311=CARTESIAN_POINT('Ctrl Pts',(-30.0506856115286,645.565837705453,
62.7707392571429));
#103312=CARTESIAN_POINT('Ctrl Pts',(-29.45958992671,645.548440539176,61.3580945430258));
#103313=CARTESIAN_POINT('Ctrl Pts',(-29.0222871239381,645.535569814948,
60.7102226359645));
#103314=CARTESIAN_POINT('Ctrl Pts',(-27.9300847139336,645.50342404321,59.6290311800515));
#103315=CARTESIAN_POINT('Ctrl Pts',(-27.275614819367,645.484161643149,59.1961370117062));
#103316=CARTESIAN_POINT('Ctrl Pts',(-25.8485836001921,645.442161168378,
58.6110004122124));
#103317=CARTESIAN_POINT('Ctrl Pts',(-25.0765837225069,645.419439618224,
58.4589881954405));
#103318=CARTESIAN_POINT('Ctrl Pts',(-23.5319762612537,645.373978631996,
58.4589881954405));
#103319=CARTESIAN_POINT('Ctrl Pts',(-22.7599763835685,645.351257081842,
58.6110004122124));
#103320=CARTESIAN_POINT('Ctrl Pts',(-21.3329451643936,645.309256607071,
59.1961370117062));
#103321=CARTESIAN_POINT('Ctrl Pts',(-20.6784752698267,645.28999420701,59.6290311800517));
#103322=CARTESIAN_POINT('Ctrl Pts',(-19.5862728598228,645.257848435272,
60.7102226359643));
#103323=CARTESIAN_POINT('Ctrl Pts',(-19.1489700570509,645.244977711044,
61.358094543025));
#103324=CARTESIAN_POINT('Ctrl Pts',(-18.5578743722317,645.227580544767,
62.7707392571437));
#103325=CARTESIAN_POINT('Ctrl Pts',(-18.4043140488817,645.223060947511,
63.5348184358976));
#103326=CARTESIAN_POINT('Ctrl Pts',(-18.4043140488937,645.223060947443,
64.2994740882088));
#103327=CARTESIAN_POINT('Origin',(-29.2194381818547,645.39670912511,64.2994740882088));
#103328=CARTESIAN_POINT('Origin',(-26.4620031331058,633.159653102509,64.2994740882088));
#103329=CARTESIAN_POINT('',(-31.2678407122057,639.538553970656,64.2994740877864));
#103330=CARTESIAN_POINT('Ctrl Pts',(-19.6604693917099,639.614613618721,
62.5660159449655));
#103331=CARTESIAN_POINT('Ctrl Pts',(-19.7556504099892,639.582567616465,
62.282332691133));
#103332=CARTESIAN_POINT('Ctrl Pts',(-19.8718432110569,639.544021407052,
62.0111775190741));
#103333=CARTESIAN_POINT('Ctrl Pts',(-20.0074654347315,639.500530839039,
61.7514240468761));
#103334=CARTESIAN_POINT('Ctrl Pts',(-20.032231644244,639.492588950976,61.7039900147554));
#103335=CARTESIAN_POINT('Ctrl Pts',(-20.057645885894,639.484482149599,61.6569362630971));
#103336=CARTESIAN_POINT('Ctrl Pts',(-20.0836986773465,639.476219869507,
61.6102560203614));
#103337=CARTESIAN_POINT('Ctrl Pts',(-20.101297793179,639.470638554942,61.5787227007747));
#103338=CARTESIAN_POINT('Ctrl Pts',(-20.1191895721033,639.464985737746,
61.5473576036808));
#103339=CARTESIAN_POINT('Ctrl Pts',(-20.1373704921135,639.459264520637,
61.516159925298));
#103340=CARTESIAN_POINT('Ctrl Pts',(-20.2253501924973,639.43157884979,61.3651905356716));
#103341=CARTESIAN_POINT('Ctrl Pts',(-20.3201686033712,639.402279383082,
61.2181734019715));
#103342=CARTESIAN_POINT('Ctrl Pts',(-20.4217102305742,639.371692235151,
61.0751674764617));
#103343=CARTESIAN_POINT('Ctrl Pts',(-20.4312396758219,639.368821702547,
61.0617467033779));
#103344=CARTESIAN_POINT('Ctrl Pts',(-20.4408283027393,639.365939834986,
61.0483612397612));
#103345=CARTESIAN_POINT('Ctrl Pts',(-20.4504759958362,639.363046905543,
61.0350111227245));
#103346=CARTESIAN_POINT('Ctrl Pts',(-20.5204449471276,639.342066217495,
60.9381907036576));
#103347=CARTESIAN_POINT('Ctrl Pts',(-20.5938065024781,639.320423943129,
60.8429238161653));
#103348=CARTESIAN_POINT('Ctrl Pts',(-20.6698874971932,639.298416870665,
60.7499994453728));
#103349=CARTESIAN_POINT('Ctrl Pts',(-20.7162781708621,639.284997975173,
60.6933384595712));
#103350=CARTESIAN_POINT('Ctrl Pts',(-20.7636535181521,639.271451210823,
60.6375798052197));
#103351=CARTESIAN_POINT('Ctrl Pts',(-20.8118752315682,639.257838908372,
60.5828777103897));
#103352=CARTESIAN_POINT('Ctrl Pts',(-20.9167303497794,639.228239802877,
60.4639314056347));
#103353=CARTESIAN_POINT('Ctrl Pts',(-21.0254306336414,639.198358602934,
60.3499372916202));
#103354=CARTESIAN_POINT('Ctrl Pts',(-21.1379837166309,639.168414488515,
60.2406077607254));
#103355=CARTESIAN_POINT('Ctrl Pts',(-21.252662669507,639.137904798375,60.129213245458));
#103356=CARTESIAN_POINT('Ctrl Pts',(-21.3713413391399,639.107329448174,
60.0226612620548));
#103357=CARTESIAN_POINT('Ctrl Pts',(-21.494062811382,639.076916809791,59.9206887222358));
#103358=CARTESIAN_POINT('Ctrl Pts',(-21.5446960815533,639.064368954002,
59.8786161894965));
#103359=CARTESIAN_POINT('Ctrl Pts',(-21.5960179561576,639.051848786154,
59.8373236768977));
#103360=CARTESIAN_POINT('Ctrl Pts',(-21.6480331481804,639.03937239533,59.7967946409827));
#103361=CARTESIAN_POINT('Ctrl Pts',(-21.7727113592165,639.009467015235,
59.6996482593893));
#103362=CARTESIAN_POINT('Ctrl Pts',(-21.9019771385064,638.979701094277,
59.6066175164186));
#103363=CARTESIAN_POINT('Ctrl Pts',(-22.0351170267143,638.950494813038,
59.5182198819255));
#103364=CARTESIAN_POINT('Ctrl Pts',(-22.0990564322483,638.936468721493,
59.4757675990208));
#103365=CARTESIAN_POINT('Ctrl Pts',(-22.163889678691,638.922571825977,59.4343845095441));
#103366=CARTESIAN_POINT('Ctrl Pts',(-22.2295390374144,638.908851679777,
59.3941319438193));
#103367=CARTESIAN_POINT('Ctrl Pts',(-22.3576108890827,638.882085774319,
59.3156053484799));
#103368=CARTESIAN_POINT('Ctrl Pts',(-22.4883155563332,638.856091013215,
59.2416680648132));
#103369=CARTESIAN_POINT('Ctrl Pts',(-22.6210518826277,638.831204223815,
59.1726911130992));
#103370=CARTESIAN_POINT('Ctrl Pts',(-22.7582179760615,638.805486895519,
59.1014122155458));
#103371=CARTESIAN_POINT('Ctrl Pts',(-22.8975352876073,638.780921855692,
59.0352728308619));
#103372=CARTESIAN_POINT('Ctrl Pts',(-23.0391982842766,638.757684060641,
58.974232786797));
#103373=CARTESIAN_POINT('Ctrl Pts',(-23.07924643566,638.751114732335,58.9569767567635));
#103374=CARTESIAN_POINT('Ctrl Pts',(-23.1194821783114,638.744651545692,
58.9401285470228));
#103375=CARTESIAN_POINT('Ctrl Pts',(-23.159910205694,638.738298632261,58.9236879248849));
#103376=CARTESIAN_POINT('Ctrl Pts',(-23.3335921112647,638.711006029033,
58.8530577515488));
#103377=CARTESIAN_POINT('Ctrl Pts',(-23.5106709624866,638.685770612436,
58.7900097568909));
#103378=CARTESIAN_POINT('Ctrl Pts',(-23.6913019668401,638.662951844834,
58.7345974353322));
#103379=CARTESIAN_POINT('Ctrl Pts',(-23.8453703780755,638.643488678566,
58.6873337422804));
#103380=CARTESIAN_POINT('Ctrl Pts',(-24.0027408049985,638.625730877479,
58.6455484140267));
#103381=CARTESIAN_POINT('Ctrl Pts',(-24.1612188560548,638.610135581286,
58.6099678299653));
#103382=CARTESIAN_POINT('Ctrl Pts',(-24.1934780298083,638.606961063639,
58.6027251850954));
#103383=CARTESIAN_POINT('Ctrl Pts',(-24.2257795091491,638.603876337104,
58.5957405138027));
#103384=CARTESIAN_POINT('Ctrl Pts',(-24.2581039558078,638.600885318481,
58.5890200208385));
#103385=CARTESIAN_POINT('Ctrl Pts',(-24.4490665789934,638.583215324987,
58.5493174706578));
#103386=CARTESIAN_POINT('Ctrl Pts',(-24.6409245786182,638.568764510727,
58.5186878559351));
#103387=CARTESIAN_POINT('Ctrl Pts',(-24.8336179601762,638.557716475292,
58.4971174009262));
#103388=CARTESIAN_POINT('Ctrl Pts',(-24.956409356204,638.550676255833,58.4833719040021));
#103389=CARTESIAN_POINT('Ctrl Pts',(-25.0797134668603,638.545021125185,
58.4732899575493));
#103390=CARTESIAN_POINT('Ctrl Pts',(-25.2033487449366,638.540792331728,
58.4669566006054));
#103391=CARTESIAN_POINT('Ctrl Pts',(-25.3294688219745,638.536478548761,
58.4604959570246));
#103392=CARTESIAN_POINT('Ctrl Pts',(-25.4559981094795,638.533643884368,
58.457928470776));
#103393=CARTESIAN_POINT('Ctrl Pts',(-25.582949758537,638.532336794653,58.4593676132319));
#103394=CARTESIAN_POINT('Ctrl Pts',(-25.6324008606534,638.531827647844,
58.4599281981559));
#103395=CARTESIAN_POINT('Ctrl Pts',(-25.681916058785,638.531550479522,58.4610972295894));
#103396=CARTESIAN_POINT('Ctrl Pts',(-25.7314961026847,638.531508928283,
58.4628834273625));
#103397=CARTESIAN_POINT('Ctrl Pts',(-25.8208733205009,638.531434024473,
58.4661033798851));
#103398=CARTESIAN_POINT('Ctrl Pts',(-25.9103675409668,638.532125410603,
58.4713269333322));
#103399=CARTESIAN_POINT('Ctrl Pts',(-25.9998450012477,638.533598565417,
58.4785846158281));
#103400=CARTESIAN_POINT('Ctrl Pts',(-26.0874286185417,638.535040540045,
58.4856886852124));
#103401=CARTESIAN_POINT('Ctrl Pts',(-26.1744866897434,638.537216683504,
58.4946845281867));
#103402=CARTESIAN_POINT('Ctrl Pts',(-26.260956425424,638.54010194845,58.5055543459801));
#103403=CARTESIAN_POINT('Ctrl Pts',(-26.4140421982678,638.545210013261,
58.5247982403261));
#103404=CARTESIAN_POINT('Ctrl Pts',(-26.5656810056143,638.552564467409,
58.5499668723704));
#103405=CARTESIAN_POINT('Ctrl Pts',(-26.7157330220559,638.562036190887,
58.5810246871823));
#103406=CARTESIAN_POINT('Ctrl Pts',(-26.858938066883,638.571075713429,58.6106653135986));
#103407=CARTESIAN_POINT('Ctrl Pts',(-27.0006979484278,638.582043429483,
58.6456695550396));
#103408=CARTESIAN_POINT('Ctrl Pts',(-27.1409029558934,638.594812782266,
58.6859663162781));
#103409=CARTESIAN_POINT('Ctrl Pts',(-27.1893002543444,638.599220628953,
58.699876335724));
#103410=CARTESIAN_POINT('Ctrl Pts',(-27.2375765636139,638.603856450057,
58.7144595173002));
#103411=CARTESIAN_POINT('Ctrl Pts',(-27.2856852257159,638.608706436981,
58.7296967699079));
#103412=CARTESIAN_POINT('Ctrl Pts',(-27.415223027167,638.621765553902,58.7707247286313));
#103413=CARTESIAN_POINT('Ctrl Pts',(-27.5439630743014,638.636437015089,
58.8166317822243));
#103414=CARTESIAN_POINT('Ctrl Pts',(-27.6709204151557,638.652471757745,
58.8670909282801));
#103415=CARTESIAN_POINT('Ctrl Pts',(-27.7999621376017,638.668769758297,
58.9183785109941));
#103416=CARTESIAN_POINT('Ctrl Pts',(-27.9271607180627,638.686475807047,
58.974368497831));
#103417=CARTESIAN_POINT('Ctrl Pts',(-28.0514926947167,638.705312224822,
59.0346686070573));
#103418=CARTESIAN_POINT('Ctrl Pts',(-28.106553485054,638.713653989167,59.0613726920464));
#103419=CARTESIAN_POINT('Ctrl Pts',(-28.1610523512498,638.722217263826,
59.0889214729824));
#103420=CARTESIAN_POINT('Ctrl Pts',(-28.2149021938079,638.730977240033,
59.1172782101099));
#103421=CARTESIAN_POINT('Ctrl Pts',(-28.2278313024328,638.733080471511,
59.1240865370642));
#103422=CARTESIAN_POINT('Ctrl Pts',(-28.2407267529919,638.735194947273,
59.1309410998825));
#103423=CARTESIAN_POINT('Ctrl Pts',(-28.2535884192766,638.737320402262,
59.1378417863349));
#103424=CARTESIAN_POINT('Ctrl Pts',(-28.5599916610745,638.787955077793,
59.3022367140878));
#103425=CARTESIAN_POINT('Ctrl Pts',(-28.8480542326587,638.844955355957,
59.4932554983916));
#103426=CARTESIAN_POINT('Ctrl Pts',(-29.1182177859427,638.905258731902,
59.7110768906355));
#103427=CARTESIAN_POINT('Ctrl Pts',(-29.1344578639101,638.908883689877,
59.7241705753683));
#103428=CARTESIAN_POINT('Ctrl Pts',(-29.1506332937596,638.912520616295,
59.7373611342055));
#103429=CARTESIAN_POINT('Ctrl Pts',(-29.1667441676304,638.916168843431,
59.7506486031058));
#103430=CARTESIAN_POINT('Ctrl Pts',(-29.3144417784627,638.949614231696,
59.8724624430206));
#103431=CARTESIAN_POINT('Ctrl Pts',(-29.4573274362203,638.984191717442,
60.0032376747088));
#103432=CARTESIAN_POINT('Ctrl Pts',(-29.5918674028682,639.018481680813,
60.1396878642134));
#103433=CARTESIAN_POINT('Ctrl Pts',(-29.6867899181019,639.042674414403,
60.2359581065406));
#103434=CARTESIAN_POINT('Ctrl Pts',(-29.7778370811571,639.066776771326,
60.3352163695295));
#103435=CARTESIAN_POINT('Ctrl Pts',(-29.8651104143972,639.09060876673,60.4374188246835));
#103436=CARTESIAN_POINT('Ctrl Pts',(-29.9015533966364,639.100560363088,
60.4800958042338));
#103437=CARTESIAN_POINT('Ctrl Pts',(-29.9373294444809,639.110462869717,
60.5232757287555));
#103438=CARTESIAN_POINT('Ctrl Pts',(-29.9724503412504,639.120304145742,
60.5669591429136));
#103439=CARTESIAN_POINT('Ctrl Pts',(-30.0771776841521,639.149649942222,
60.6972191395098));
#103440=CARTESIAN_POINT('Ctrl Pts',(-30.1762070237057,639.178479714589,
60.8320715218747));
#103441=CARTESIAN_POINT('Ctrl Pts',(-30.2694728974752,639.206447349291,
60.9715318367259));
#103442=CARTESIAN_POINT('Ctrl Pts',(-30.3375768093777,639.22686966726,61.0733675094394));
#103443=CARTESIAN_POINT('Ctrl Pts',(-30.4026067951602,639.246832284511,
61.1776608748026));
#103444=CARTESIAN_POINT('Ctrl Pts',(-30.4645235373007,639.266198028526,
61.284428590957));
#103445=CARTESIAN_POINT('Ctrl Pts',(-30.5108974286489,639.280702423908,
61.3643945952601));
#103446=CARTESIAN_POINT('Ctrl Pts',(-30.5555184235738,639.294872545955,
61.4457413550946));
#103447=CARTESIAN_POINT('Ctrl Pts',(-30.598331303557,639.308639388708,61.5284018708633));
#103448=CARTESIAN_POINT('Ctrl Pts',(-30.636366414163,639.320869899411,61.6018377588772));
#103449=CARTESIAN_POINT('Ctrl Pts',(-30.6727477715507,639.332705897609,
61.6758548871431));
#103450=CARTESIAN_POINT('Ctrl Pts',(-30.7074777887601,639.344119541394,
61.7504116450392));
#103451=CARTESIAN_POINT('Ctrl Pts',(-30.7813004242086,639.368380550517,
61.9088905863311));
#103452=CARTESIAN_POINT('Ctrl Pts',(-30.8477744207413,639.390757120824,
62.0700388044301));
#103453=CARTESIAN_POINT('Ctrl Pts',(-30.9070565975758,639.411020592166,
62.2338230900162));
#103454=CARTESIAN_POINT('Ctrl Pts',(-30.9505698013699,639.425894009526,
62.3540409932298));
#103455=CARTESIAN_POINT('Ctrl Pts',(-30.9901926242488,639.439629706583,
62.4756348854126));
#103456=CARTESIAN_POINT('Ctrl Pts',(-31.0260078756452,639.452145446073,
62.598642517993));
#103457=CARTESIAN_POINT('Ctrl Pts',(-31.0749693290293,639.469255162511,
62.7668008369673));
#103458=CARTESIAN_POINT('Ctrl Pts',(-31.116758386068,639.484088469113,62.9376198059619));
#103459=CARTESIAN_POINT('Ctrl Pts',(-31.1512286201053,639.496418452856,
63.1113174708579));
#103460=CARTESIAN_POINT('Ctrl Pts',(-31.1546163045033,639.497630225701,
63.128388224387));
#103461=CARTESIAN_POINT('Ctrl Pts',(-31.157933261746,639.498817806503,63.1454867960826));
#103462=CARTESIAN_POINT('Ctrl Pts',(-31.1611793284332,639.499980970938,
63.1626134020239));
#103463=CARTESIAN_POINT('Ctrl Pts',(-31.1665764304226,639.501914916752,
63.1910891075168));
#103464=CARTESIAN_POINT('Ctrl Pts',(-31.1717730915779,639.503779752154,
63.2196340647483));
#103465=CARTESIAN_POINT('Ctrl Pts',(-31.1767679222504,639.505574492154,
63.2482357712307));
#103466=CARTESIAN_POINT('Ctrl Pts',(-31.205332312064,639.515838234079,63.4118029363383));
#103467=CARTESIAN_POINT('Ctrl Pts',(-31.2272400925891,639.523787147066,
63.5768839956324));
#103468=CARTESIAN_POINT('Ctrl Pts',(-31.2422935239496,639.529260134671,
63.741146664961));
#103469=CARTESIAN_POINT('Ctrl Pts',(-31.2580716979021,639.534996617496,
63.913317707462));
#103470=CARTESIAN_POINT('Ctrl Pts',(-31.2665570468194,639.538079648504,
64.0854433189719));
#103471=CARTESIAN_POINT('Ctrl Pts',(-31.2677422818647,639.538509777967,
64.2576679511823));
#103472=CARTESIAN_POINT('Ctrl Pts',(-31.2678381792997,639.538544579767,
64.2716026559762));
#103473=CARTESIAN_POINT('Ctrl Pts',(-31.2678862604399,639.538562004858,
64.2855380090525));
#103474=CARTESIAN_POINT('Ctrl Pts',(-31.2678865073884,639.538562048433,
64.2994740869496));
#103475=CARTESIAN_POINT('',(-32.2137589216624,634.173842834478,64.2994740882088));
#103476=CARTESIAN_POINT('Ctrl Pts',(-18.4043140488937,645.223060947443,
64.2994740882088));
#103477=CARTESIAN_POINT('Ctrl Pts',(-18.4043140488817,645.223060947511,
65.0641297405231));
#103478=CARTESIAN_POINT('Ctrl Pts',(-18.55787437223,645.227580544767,65.8282089192698));
#103479=CARTESIAN_POINT('Ctrl Pts',(-19.1489700570526,645.244977711044,
67.2408536333967));
#103480=CARTESIAN_POINT('Ctrl Pts',(-19.5862728598217,645.257848435272,
67.8887255404523));
#103481=CARTESIAN_POINT('Ctrl Pts',(-20.6784752698278,645.28999420701,68.969916996367));
#103482=CARTESIAN_POINT('Ctrl Pts',(-21.3329451643959,645.309256607072,
69.4028111647124));
#103483=CARTESIAN_POINT('Ctrl Pts',(-22.7599763835661,645.351257081842,
69.9879477642043));
#103484=CARTESIAN_POINT('Ctrl Pts',(-23.5319762612528,645.373978631996,
70.1399599809771));
#103485=CARTESIAN_POINT('Ctrl Pts',(-25.0765837225078,645.419439618224,
70.1399599809771));
#103486=CARTESIAN_POINT('Ctrl Pts',(-25.8485836001935,645.442161168379,
69.9879477642046));
#103487=CARTESIAN_POINT('Ctrl Pts',(-27.2756148193656,645.484161643148,
69.402811164712));
#103488=CARTESIAN_POINT('Ctrl Pts',(-27.9300847139356,645.50342404321,68.9699169963641));
#103489=CARTESIAN_POINT('Ctrl Pts',(-29.0222871239361,645.535569814948,
67.8887255404551));
#103490=CARTESIAN_POINT('Ctrl Pts',(-29.4595899267082,645.548440539176,
67.2408536333963));
#103491=CARTESIAN_POINT('Ctrl Pts',(-30.0506856115305,645.565837705453,
65.8282089192702));
#103492=CARTESIAN_POINT('Ctrl Pts',(-30.2042459348789,645.570357302709,
65.0641297405228));
#103493=CARTESIAN_POINT('Ctrl Pts',(-30.204245934867,645.570357302777,64.2994740882088));
#103494=CARTESIAN_POINT('Ctrl Pts',(-31.2678163619919,639.53854967554,64.2994740882313));
#103495=CARTESIAN_POINT('Ctrl Pts',(-31.2678163619908,639.53854967554,64.5926872821248));
#103496=CARTESIAN_POINT('Ctrl Pts',(-31.2468826932858,639.530860720871,
64.885924677304));
#103497=CARTESIAN_POINT('Ctrl Pts',(-31.1615715333149,639.500058690408,
65.4724494968625));
#103498=CARTESIAN_POINT('Ctrl Pts',(-31.0977211744434,639.477145594786,
65.7607708453645));
#103499=CARTESIAN_POINT('Ctrl Pts',(-31.0141476947143,639.44800149248,66.0405185693756));
#103500=CARTESIAN_POINT('Origin',(-33.3604437899019,646.39670912511,26.2994740882088));
#103501=CARTESIAN_POINT('Ctrl Pts',(-29.2194381818547,646.39670912511,64.2994740882088));
#103502=CARTESIAN_POINT('Ctrl Pts',(-29.2194381818525,646.39670912511,64.9332064464068));
#103503=CARTESIAN_POINT('Ctrl Pts',(-29.0915097686747,646.39670912511,65.5664610340562));
#103504=CARTESIAN_POINT('Ctrl Pts',(-28.8452940426529,646.39670912511,66.1518478439682));
#103505=CARTESIAN_POINT('Ctrl Pts',(-28.5990783166312,646.39670912511,66.7372346538801));
#103506=CARTESIAN_POINT('Ctrl Pts',(-28.2347690183583,646.39670912511,67.2741788198361));
#103507=CARTESIAN_POINT('Ctrl Pts',(-27.7798216786158,646.39670912511,67.7222144872231));
#103508=CARTESIAN_POINT('Ctrl Pts',(-27.3248743388734,646.39670912511,68.1702501546101));
#103509=CARTESIAN_POINT('Ctrl Pts',(-26.779646943758,646.39670912511,68.529024776011));
#103510=CARTESIAN_POINT('Ctrl Pts',(-26.1852295986371,646.39670912511,68.7714999319471));
#103511=CARTESIAN_POINT('Ctrl Pts',(-25.5908122535162,646.39670912511,69.0139750878831));
#103512=CARTESIAN_POINT('Ctrl Pts',(-24.9476726899776,646.39670912511,69.1399599809771));
#103513=CARTESIAN_POINT('Ctrl Pts',(-24.3042799918803,646.39670912511,69.1399599809771));
#103514=CARTESIAN_POINT('Ctrl Pts',(-23.660887293783,646.39670912511,69.1399599809771));
#103515=CARTESIAN_POINT('Ctrl Pts',(-23.0177477302444,646.39670912511,69.0139750878831));
#103516=CARTESIAN_POINT('Ctrl Pts',(-22.4233303851235,646.39670912511,68.771499931947));
#103517=CARTESIAN_POINT('Ctrl Pts',(-21.8289130400026,646.39670912511,68.529024776011));
#103518=CARTESIAN_POINT('Ctrl Pts',(-21.2836856448871,646.39670912511,68.1702501546155));
#103519=CARTESIAN_POINT('Ctrl Pts',(-20.8287383051448,646.39670912511,67.7222144872231));
#103520=CARTESIAN_POINT('Ctrl Pts',(-20.3737909654025,646.39670912511,67.2741788198307));
#103521=CARTESIAN_POINT('Ctrl Pts',(-20.0094816671294,646.39670912511,66.7372346538801));
#103522=CARTESIAN_POINT('Ctrl Pts',(-19.7632659411077,646.39670912511,66.1518478439682));
#103523=CARTESIAN_POINT('Ctrl Pts',(-19.517050215086,646.39670912511,65.5664610340562));
#103524=CARTESIAN_POINT('Ctrl Pts',(-19.3891218019081,646.39670912511,64.9332064464068));
#103525=CARTESIAN_POINT('Ctrl Pts',(-19.3891218019059,646.39670912511,64.2994740882088));
#103526=CARTESIAN_POINT('Ctrl Pts',(-19.3891218019059,646.39670912511,64.2994740882088));
#103527=CARTESIAN_POINT('Ctrl Pts',(-18.1973682093116,646.39670912511,64.2994740882088));
#103528=CARTESIAN_POINT('Ctrl Pts',(-18.4043140488937,645.223060947443,
64.2994740882088));
#103529=CARTESIAN_POINT('Ctrl Pts',(-19.3891218019081,646.39670912511,64.9332064464068));
#103530=CARTESIAN_POINT('Ctrl Pts',(-18.1973682094106,646.39670912511,65.0917744634339));
#103531=CARTESIAN_POINT('Ctrl Pts',(-18.4043140488817,645.223060947511,
65.0641297405231));
#103532=CARTESIAN_POINT('Ctrl Pts',(-19.517050215086,646.39670912511,65.5664610340562));
#103533=CARTESIAN_POINT('Ctrl Pts',(-18.3617148294095,646.39670912511,65.8791739609459));
#103534=CARTESIAN_POINT('Ctrl Pts',(-18.55787437223,645.227580544767,65.8282089192698));
#103535=CARTESIAN_POINT('Ctrl Pts',(-20.0094816671294,646.39670912511,66.7372346538801));
#103536=CARTESIAN_POINT('Ctrl Pts',(-18.9941367827525,646.39670912511,67.3286306783986));
#103537=CARTESIAN_POINT('Ctrl Pts',(-19.1489700570526,645.244977711044,
67.2408536333967));
#103538=CARTESIAN_POINT('Ctrl Pts',(-20.3737909654025,646.39670912511,67.2741788198307));
#103539=CARTESIAN_POINT('Ctrl Pts',(-19.4561930076916,646.39670912511,67.984534756338));
#103540=CARTESIAN_POINT('Ctrl Pts',(-19.5862728598217,645.257848435272,
67.8887255404523));
#103541=CARTESIAN_POINT('Ctrl Pts',(-21.2836856448871,646.39670912511,68.1702501546155));
#103542=CARTESIAN_POINT('Ctrl Pts',(-20.6031006941251,646.39670912511,69.0621896001028));
#103543=CARTESIAN_POINT('Ctrl Pts',(-20.6784752698278,645.28999420701,68.969916996367));
#103544=CARTESIAN_POINT('Ctrl Pts',(-21.8289130400026,646.39670912511,68.529024776011));
#103545=CARTESIAN_POINT('Ctrl Pts',(-21.2802434100837,646.39670912511,69.4841561744855));
#103546=CARTESIAN_POINT('Ctrl Pts',(-21.3329451643959,645.309256607072,
69.4028111647124));
#103547=CARTESIAN_POINT('Ctrl Pts',(-23.0177477302444,646.39670912511,69.0139750878831));
#103548=CARTESIAN_POINT('Ctrl Pts',(-22.7425774139599,646.39670912511,70.0319693513056));
#103549=CARTESIAN_POINT('Ctrl Pts',(-22.7599763835661,645.351257081842,
69.9879477642043));
#103550=CARTESIAN_POINT('Ctrl Pts',(-23.660887293783,646.39670912511,69.1399599809771));
#103551=CARTESIAN_POINT('Ctrl Pts',(-23.5230979344017,646.39670912511,70.1629517811265));
#103552=CARTESIAN_POINT('Ctrl Pts',(-23.5319762612528,645.373978631996,
70.1399599809771));
#103553=CARTESIAN_POINT('Ctrl Pts',(-24.9476726899776,646.39670912511,69.1399599809771));
#103554=CARTESIAN_POINT('Ctrl Pts',(-25.0679049368901,646.39670912511,70.1174849228819));
#103555=CARTESIAN_POINT('Ctrl Pts',(-25.0765837225078,645.419439618224,
70.1399599809771));
#103556=CARTESIAN_POINT('Ctrl Pts',(-25.5908122535162,646.39670912511,69.0139750878831));
#103557=CARTESIAN_POINT('Ctrl Pts',(-25.832528214473,646.39670912511,69.9473649702541));
#103558=CARTESIAN_POINT('Ctrl Pts',(-25.8485836001935,645.442161168379,
69.9879477642046));
#103559=CARTESIAN_POINT('Ctrl Pts',(-26.779646943758,646.39670912511,68.529024776011));
#103560=CARTESIAN_POINT('Ctrl Pts',(-27.2309350653711,646.39670912511,69.3342934556171));
#103561=CARTESIAN_POINT('Ctrl Pts',(-27.2756148193656,645.484161643148,
69.402811164712));
#103562=CARTESIAN_POINT('Ctrl Pts',(-27.3248743388734,646.39670912511,68.1702501546101));
#103563=CARTESIAN_POINT('Ctrl Pts',(-27.8689763870033,646.39670912511,68.8953702631505));
#103564=CARTESIAN_POINT('Ctrl Pts',(-27.9300847139356,645.50342404321,68.9699169963641));
#103565=CARTESIAN_POINT('Ctrl Pts',(-28.2347690183583,646.39670912511,67.2741788198361));
#103566=CARTESIAN_POINT('Ctrl Pts',(-28.9235388845863,646.39670912511,67.8163374818037));
#103567=CARTESIAN_POINT('Ctrl Pts',(-29.0222871239361,645.535569814948,
67.8887255404551));
#103568=CARTESIAN_POINT('Ctrl Pts',(-28.5990783166312,646.39670912511,66.7372346538801));
#103569=CARTESIAN_POINT('Ctrl Pts',(-29.3454369712419,646.39670912511,67.1763037368409));
#103570=CARTESIAN_POINT('Ctrl Pts',(-29.4595899267082,645.548440539176,
67.2408536333963));
#103571=CARTESIAN_POINT('Ctrl Pts',(-29.0915097686747,646.39670912511,65.5664610340562));
#103572=CARTESIAN_POINT('Ctrl Pts',(-29.9111456379665,646.39670912511,65.7921343507568));
#103573=CARTESIAN_POINT('Ctrl Pts',(-30.0506856115305,645.565837705453,
65.8282089192702));
#103574=CARTESIAN_POINT('Ctrl Pts',(-29.2194381818525,646.39670912511,64.9332064464067));
#103575=CARTESIAN_POINT('Ctrl Pts',(-30.058537813076,646.39670912511,65.04472225858));
#103576=CARTESIAN_POINT('Ctrl Pts',(-30.2042459348789,645.570357302709,
65.0641297405228));
#103577=CARTESIAN_POINT('Ctrl Pts',(-29.2194381818547,646.39670912511,64.2994740882088));
#103578=CARTESIAN_POINT('Ctrl Pts',(-30.058537813032,646.39670912511,64.2994740882088));
#103579=CARTESIAN_POINT('Ctrl Pts',(-30.204245934867,645.570357302777,64.2994740882088));
#103580=CARTESIAN_POINT('Origin',(-48.,620.675373764374,64.2994740882088));
#103581=CARTESIAN_POINT('Ctrl Pts',(-2.31092134190293,635.230245103769,
51.3976052199539));
#103582=CARTESIAN_POINT('Ctrl Pts',(-1.92439042612671,635.165593126578,
51.3246699561202));
#103583=CARTESIAN_POINT('Ctrl Pts',(-1.53337526906528,635.116006409181,
51.2697641942075));
#103584=CARTESIAN_POINT('Ctrl Pts',(-1.1377271716918,635.083088344485,51.2334761581173));
#103585=CARTESIAN_POINT('Ctrl Pts',(-1.10108396587682,635.080039616517,
51.2301153180579));
#103586=CARTESIAN_POINT('Ctrl Pts',(-1.06440101541229,635.077133844473,
51.2269141451115));
#103587=CARTESIAN_POINT('Ctrl Pts',(-1.02767819909564,635.074372288393,
51.223873088555));
#103588=CARTESIAN_POINT('Ctrl Pts',(-1.02189271947806,635.07393722028,51.2233939866645));
#103589=CARTESIAN_POINT('Ctrl Pts',(-1.0161058148073,635.073505788182,51.2229189177151));
#103590=CARTESIAN_POINT('Ctrl Pts',(-1.01031752097321,635.07307799376,51.2224478826357));
#103591=CARTESIAN_POINT('Ctrl Pts',(-0.769279298802908,635.055263623935,
51.2028328697539));
#103592=CARTESIAN_POINT('Ctrl Pts',(-0.525719603099018,635.043759102955,
51.1902149545465));
#103593=CARTESIAN_POINT('Ctrl Pts',(-0.282374958370322,635.038699233314,
51.1846774469337));
#103594=CARTESIAN_POINT('Ctrl Pts',(-0.0944016631441944,635.034790701155,
51.180399959938));
#103595=CARTESIAN_POINT('Ctrl Pts',(0.093442328449993,635.034726965756,
51.1803465302695));
#103596=CARTESIAN_POINT('Ctrl Pts',(0.279895468563292,635.038555816393,
51.1845398016811));
#103597=CARTESIAN_POINT('Ctrl Pts',(0.291911936050454,635.038802576835,
51.1848100481867));
#103598=CARTESIAN_POINT('Ctrl Pts',(0.303924672822358,635.039065220646,
51.1850974258479));
#103599=CARTESIAN_POINT('Ctrl Pts',(0.315933663727289,635.039343708228,
51.1854019212719));
#103600=CARTESIAN_POINT('Ctrl Pts',(0.743857359011281,635.049267226064,
51.1962521923799));
#103601=CARTESIAN_POINT('Ctrl Pts',(1.16718217071826,635.079312657792,51.2288431932868));
#103602=CARTESIAN_POINT('Ctrl Pts',(1.58621543213723,635.127765019396,51.2826473556403));
#103603=CARTESIAN_POINT('Ctrl Pts',(2.0052486935562,635.176217381,51.3364515179938));
#103604=CARTESIAN_POINT('Ctrl Pts',(2.41999047219474,635.243076943181,51.4114688925647));
#103605=CARTESIAN_POINT('Ctrl Pts',(2.83074822463683,635.326669258824,51.5072092257538));
#103606=CARTESIAN_POINT('Ctrl Pts',(2.8531115207118,635.331220359061,51.5124217126873));
#103607=CARTESIAN_POINT('Ctrl Pts',(2.8754606313574,635.335821069522,51.5176966435968));
#103608=CARTESIAN_POINT('Ctrl Pts',(2.89779414296658,635.340470518694,51.5230334110954));
#103609=CARTESIAN_POINT('Ctrl Pts',(3.2059760252613,635.404628633299,51.5966758853225));
#103610=CARTESIAN_POINT('Ctrl Pts',(3.51096003017398,635.478035219308,51.682057065885));
#103611=CARTESIAN_POINT('Ctrl Pts',(3.80902312884625,635.558364152402,51.7775305592728));
#103612=CARTESIAN_POINT('Ctrl Pts',(3.89243156637124,635.580842986002,51.804247368378));
#103613=CARTESIAN_POINT('Ctrl Pts',(3.9752983018007,635.603864039638,51.8317545824764));
#103614=CARTESIAN_POINT('Ctrl Pts',(4.05754235020458,635.627376688186,51.8600163602557));
#103615=CARTESIAN_POINT('Ctrl Pts',(4.08324888549469,635.634725897538,51.8688499768146));
#103616=CARTESIAN_POINT('Ctrl Pts',(4.10890664396029,635.642125363381,51.8777598513787));
#103617=CARTESIAN_POINT('Ctrl Pts',(4.13451596947741,635.649574255906,51.8867457715323));
#103618=CARTESIAN_POINT('Ctrl Pts',(4.42402771911023,635.733783498605,51.9883310110177));
#103619=CARTESIAN_POINT('Ctrl Pts',(4.70743818545356,635.824338401075,52.099671909975));
#103620=CARTESIAN_POINT('Ctrl Pts',(4.98507049296477,635.919988661691,52.2203911200408));
#103621=CARTESIAN_POINT('Ctrl Pts',(5.06347338651508,635.947000133333,52.2544820205599));
#103622=CARTESIAN_POINT('Ctrl Pts',(5.14141563710596,635.974417869963,52.2893205600875));
#103623=CARTESIAN_POINT('Ctrl Pts',(5.21890487245677,636.002213564635,52.3248976144886));
#103624=CARTESIAN_POINT('Ctrl Pts',(5.24645122189637,636.01209454894,52.3375447643556));
#103625=CARTESIAN_POINT('Ctrl Pts',(5.27394681459041,636.022026291278,52.3502900634043));
#103626=CARTESIAN_POINT('Ctrl Pts',(5.30139053208206,636.032007124586,52.3631325099365));
#103627=CARTESIAN_POINT('Ctrl Pts',(5.66366362029753,636.163759949502,52.5326602995614));
#103628=CARTESIAN_POINT('Ctrl Pts',(6.01738163217709,636.304261509107,52.7193702986017));
#103629=CARTESIAN_POINT('Ctrl Pts',(6.36015875743509,636.449853171429,52.9212117806643));
#103630=CARTESIAN_POINT('Ctrl Pts',(6.6668495712861,636.58011748056,53.1018041359916));
#103631=CARTESIAN_POINT('Ctrl Pts',(6.96478180978636,636.714455521892,53.294508596502));
#103632=CARTESIAN_POINT('Ctrl Pts',(7.252286828916,636.850261023332,53.4978360667219));
#103633=CARTESIAN_POINT('Ctrl Pts',(7.286115672764,636.866240372548,53.5217602864134));
#103634=CARTESIAN_POINT('Ctrl Pts',(7.31980020593987,636.882240065713,53.5458315632047));
#103635=CARTESIAN_POINT('Ctrl Pts',(7.3533377524904,636.89825588133,53.5700474603553));
#103636=CARTESIAN_POINT('Ctrl Pts',(7.38103000654088,636.911480284439,53.5900427445943));
#103637=CARTESIAN_POINT('Ctrl Pts',(7.40863101404073,636.924718513479,53.6101387611507));
#103638=CARTESIAN_POINT('Ctrl Pts',(7.43614101292839,636.937969405349,53.6303357171611));
#103639=CARTESIAN_POINT('Ctrl Pts',(7.75229632205443,637.090253665066,53.8624467723794));
#103640=CARTESIAN_POINT('Ctrl Pts',(8.05648904258589,637.244211023545,54.1078905944875));
#103641=CARTESIAN_POINT('Ctrl Pts',(8.34929453939061,637.398218046919,54.367192659054));
#103642=CARTESIAN_POINT('Ctrl Pts',(8.64210003619533,637.552225070293,54.6264947236205));
#103643=CARTESIAN_POINT('Ctrl Pts',(8.92351801894892,637.706282566528,54.8996548343145));
#103644=CARTESIAN_POINT('Ctrl Pts',(9.19408464066941,637.858782543927,55.1872316250658));
#103645=CARTESIAN_POINT('Ctrl Pts',(9.21816683588506,637.872356037223,55.2128278363439));
#103646=CARTESIAN_POINT('Ctrl Pts',(9.24215653499201,637.885914773942,55.2385359314635));
#103647=CARTESIAN_POINT('Ctrl Pts',(9.26605121704551,637.899456160225,55.264352878163));
#103648=CARTESIAN_POINT('Ctrl Pts',(9.44919177119536,638.003243981389,55.4622266106705));
#103649=CARTESIAN_POINT('Ctrl Pts',(9.62656991923521,638.105909953643,55.6662959234571));
#103650=CARTESIAN_POINT('Ctrl Pts',(9.79718029221805,638.206352078217,55.875291238877));
#103651=CARTESIAN_POINT('Ctrl Pts',(9.86608440420505,638.246917462835,55.9596978102167));
#103652=CARTESIAN_POINT('Ctrl Pts',(9.93388438713161,638.287120177701,56.0449084297527));
#103653=CARTESIAN_POINT('Ctrl Pts',(10.0005127777516,638.326887615128,56.1308414745918));
#103654=CARTESIAN_POINT('Ctrl Pts',(10.0215035613001,638.339416053284,56.1579140472159));
#103655=CARTESIAN_POINT('Ctrl Pts',(10.042387340134,638.351906539481,56.1850678260703));
#103656=CARTESIAN_POINT('Ctrl Pts',(10.0631644425131,638.3643584128,56.2123033808313));
#103657=CARTESIAN_POINT('Ctrl Pts',(10.2934195924269,638.502352051449,56.5141321262486));
#103658=CARTESIAN_POINT('Ctrl Pts',(10.5104654401652,638.635528067867,56.8258408735637));
#103659=CARTESIAN_POINT('Ctrl Pts',(10.7144165406335,638.762815059803,57.1477632880394));
#103660=CARTESIAN_POINT('Ctrl Pts',(10.7319264752442,638.773743105302,57.1754014837356));
#103661=CARTESIAN_POINT('Ctrl Pts',(10.7493409367416,638.78462813815,57.2031141332604));
#103662=CARTESIAN_POINT('Ctrl Pts',(10.7666595412329,638.795469398194,57.230901767464));
#103663=CARTESIAN_POINT('Ctrl Pts',(10.9204731636551,638.891755070628,57.477695132226));
#103664=CARTESIAN_POINT('Ctrl Pts',(11.0666558808102,638.984520457955,57.7302247072842));
#103665=CARTESIAN_POINT('Ctrl Pts',(11.2050607147562,639.073307885872,57.9890220210292));
#103666=CARTESIAN_POINT('Ctrl Pts',(11.3377551216451,639.158432044838,58.2371416500389));
#103667=CARTESIAN_POINT('Ctrl Pts',(11.4633001687123,639.239900016211,58.4910223940965));
#103668=CARTESIAN_POINT('Ctrl Pts',(11.5815311313975,639.317292073406,58.75115916475));
#103669=CARTESIAN_POINT('Ctrl Pts',(11.6797499746333,639.381584524053,58.9672644227669));
#103670=CARTESIAN_POINT('Ctrl Pts',(11.772920633671,639.443063906455,59.1876875040297));
#103671=CARTESIAN_POINT('Ctrl Pts',(11.8609291144948,639.501478257648,59.4127277678694));
#103672=CARTESIAN_POINT('Ctrl Pts',(11.8711982768748,639.508294265061,59.4389863169294));
#103673=CARTESIAN_POINT('Ctrl Pts',(11.8813850119675,639.515060403206,59.4652785322609));
#103674=CARTESIAN_POINT('Ctrl Pts',(11.8914892131512,639.52177641536,59.4916044497248));
#103675=CARTESIAN_POINT('Ctrl Pts',(11.9959186669105,639.59118808561,59.763689410277));
#103676=CARTESIAN_POINT('Ctrl Pts',(12.0913107765294,639.655087543383,60.0387465906077));
#103677=CARTESIAN_POINT('Ctrl Pts',(12.1776505788846,639.713252624643,60.3167757884058));
#103678=CARTESIAN_POINT('Ctrl Pts',(12.2628096616696,639.770622283075,60.5910028635912));
#103679=CARTESIAN_POINT('Ctrl Pts',(12.3391623321398,639.822413503614,60.8681213879122));
#103680=CARTESIAN_POINT('Ctrl Pts',(12.4066531860897,639.868389472887,61.1481479683271));
#103681=CARTESIAN_POINT('Ctrl Pts',(12.4690433776627,639.91089078029,61.407011369442));
#103682=CARTESIAN_POINT('Ctrl Pts',(12.5238602515816,639.948422497839,61.6683601245959));
#103683=CARTESIAN_POINT('Ctrl Pts',(12.5710279567737,639.980777202583,61.9322186969404));
#103684=CARTESIAN_POINT('Ctrl Pts',(12.5745024304964,639.983160519113,61.9516550819074));
#103685=CARTESIAN_POINT('Ctrl Pts',(12.5779356066442,639.985516021405,61.9711086414617));
#103686=CARTESIAN_POINT('Ctrl Pts',(12.5813273486773,639.987843586439,61.9905791155502));
#103687=CARTESIAN_POINT('Ctrl Pts',(12.6482309907011,640.033755856973,62.3746430024116));
#103688=CARTESIAN_POINT('Ctrl Pts',(12.6989827550157,640.068776619721,62.7651309615334));
#103689=CARTESIAN_POINT('Ctrl Pts',(12.7325045718648,640.091936878102,63.1594985618337));
#103690=CARTESIAN_POINT('Ctrl Pts',(12.7352361632803,640.093824137473,63.1916343841963));
#103691=CARTESIAN_POINT('Ctrl Pts',(12.7378533692285,640.095632658281,63.2237959670548));
#103692=CARTESIAN_POINT('Ctrl Pts',(12.7403556191587,640.097361925308,63.2559819337451));
#103693=CARTESIAN_POINT('Ctrl Pts',(12.7415108518539,640.098160289125,63.2708414729934));
#103694=CARTESIAN_POINT('Ctrl Pts',(12.7426411255945,640.098941441112,63.2856985588883));
#103695=CARTESIAN_POINT('Ctrl Pts',(12.7437464711904,640.099705399842,63.3005531880157));
#103696=CARTESIAN_POINT('Ctrl Pts',(12.7759162994634,640.121939551085,63.7328802989446));
#103697=CARTESIAN_POINT('Ctrl Pts',(12.7870003318299,640.129625522797,64.1634229287959));
#103698=CARTESIAN_POINT('Ctrl Pts',(12.7776731523991,640.123170325736,64.5922349254529));
#103699=CARTESIAN_POINT('Ctrl Pts',(12.7774670029556,640.123027652885,64.6017125338895));
#103700=CARTESIAN_POINT('Ctrl Pts',(12.7772508808923,640.122878071158,64.6111892966089));
#103701=CARTESIAN_POINT('Ctrl Pts',(12.7770247866986,640.122721582759,64.6206652136733));
#103702=CARTESIAN_POINT('Ctrl Pts',(12.7666730268079,640.115556735669,65.0545216369199));
#103703=CARTESIAN_POINT('Ctrl Pts',(12.7354157605725,640.093909778564,65.4866513230427));
#103704=CARTESIAN_POINT('Ctrl Pts',(12.6833305290434,640.05800335744,65.9169319880768));
#103705=CARTESIAN_POINT('Ctrl Pts',(12.6828077078149,640.057642935903,65.9212510600921));
#103706=CARTESIAN_POINT('Ctrl Pts',(12.6822827336681,640.057281040276,65.9255701772016));
#103707=CARTESIAN_POINT('Ctrl Pts',(12.6817556078935,640.056917671866,65.9298893314512));
#103708=CARTESIAN_POINT('Ctrl Pts',(12.6329480531516,640.023272715739,66.3298078474232));
#103709=CARTESIAN_POINT('Ctrl Pts',(12.5656816350177,639.976995913131,66.7301336276553));
#103710=CARTESIAN_POINT('Ctrl Pts',(12.4809092885621,639.91907782816,67.1247607525797));
#103711=CARTESIAN_POINT('Ctrl Pts',(12.4735560157396,639.914053931831,67.158991265643));
#103712=CARTESIAN_POINT('Ctrl Pts',(12.4660710046806,639.908942431424,67.1931788821358));
#103713=CARTESIAN_POINT('Ctrl Pts',(12.4584548648209,639.903743965574,67.2273196043471));
#103714=CARTESIAN_POINT('Ctrl Pts',(12.4583195473824,639.90365160342,67.2279261892));
#103715=CARTESIAN_POINT('Ctrl Pts',(12.4581841884965,639.903559213782,67.228532759456));
#103716=CARTESIAN_POINT('Ctrl Pts',(12.4580487881665,639.903466796663,67.2291393150922));
#103717=CARTESIAN_POINT('Ctrl Pts',(12.3287543193047,639.815217216541,67.8083423998278));
#103718=CARTESIAN_POINT('Ctrl Pts',(12.1635881082219,639.703112683783,68.3695526413109));
#103719=CARTESIAN_POINT('Ctrl Pts',(11.9641361655058,639.570100576874,68.9140157869479));
#103720=CARTESIAN_POINT('Ctrl Pts',(11.8692267001007,639.506806593435,69.1730992803526));
#103721=CARTESIAN_POINT('Ctrl Pts',(11.76655415419,639.438778971279,69.4283910409158));
#103722=CARTESIAN_POINT('Ctrl Pts',(11.6562914846914,639.36633818961,69.6800273323468));
#103723=CARTESIAN_POINT('Ctrl Pts',(11.6528123180315,639.364052433665,69.6879673232751));
#103724=CARTESIAN_POINT('Ctrl Pts',(11.6493255850376,639.361762281841,69.6959036824858));
#103725=CARTESIAN_POINT('Ctrl Pts',(11.6458312910723,639.359467744224,69.7038364142171));
#103726=CARTESIAN_POINT('Ctrl Pts',(11.4971366810822,639.261827024956,70.0414023038092));
#103727=CARTESIAN_POINT('Ctrl Pts',(11.3338413940789,639.155709421531,70.3735482476988));
#103728=CARTESIAN_POINT('Ctrl Pts',(11.1589239953535,639.043766058966,70.6951271369094));
#103729=CARTESIAN_POINT('Ctrl Pts',(11.1357897462097,639.028960638474,70.7376585614365));
#103730=CARTESIAN_POINT('Ctrl Pts',(11.1124522364092,639.014053343863,70.7800050873094));
#103731=CARTESIAN_POINT('Ctrl Pts',(11.08891838951,638.999050337027,70.8221547543116));
#103732=CARTESIAN_POINT('Ctrl Pts',(11.0832572973831,638.995441347632,70.8322939019418));
#103733=CARTESIAN_POINT('Ctrl Pts',(11.0775847776858,638.991826767618,70.8424218051789));
#103734=CARTESIAN_POINT('Ctrl Pts',(11.0719009273916,638.988206683529,70.8525382931254));
#103735=CARTESIAN_POINT('Ctrl Pts',(10.8933793466194,638.874505037529,71.170282661222));
#103736=CARTESIAN_POINT('Ctrl Pts',(10.7034240270576,638.755189205572,71.4776963878882));
#103737=CARTESIAN_POINT('Ctrl Pts',(10.5023371609787,638.631287386234,71.7752823633198));
#103738=CARTESIAN_POINT('Ctrl Pts',(10.477246088299,638.61582725393,71.8124143326205));
#103739=CARTESIAN_POINT('Ctrl Pts',(10.4519817462916,638.60029575369,71.8493933295574));
#103740=CARTESIAN_POINT('Ctrl Pts',(10.4265447575929,638.584694910286,71.8862203643523));
#103741=CARTESIAN_POINT('Ctrl Pts',(10.4188131204951,638.579952994446,71.89741403479));
#103742=CARTESIAN_POINT('Ctrl Pts',(10.4110654988077,638.57520465167,71.9085937144694));
#103743=CARTESIAN_POINT('Ctrl Pts',(10.4033019069229,638.570449936256,71.9197594373552));
#103744=CARTESIAN_POINT('Ctrl Pts',(10.1743043134857,638.430203204648,72.249107464377));
#103745=CARTESIAN_POINT('Ctrl Pts',(9.9314107080512,638.28440118465,72.5663065584188));
#103746=CARTESIAN_POINT('Ctrl Pts',(9.67444603037878,638.134398646701,72.8718105219762));
#103747=CARTESIAN_POINT('Ctrl Pts',(9.66485722564937,638.128801204055,72.8832106018516));
#103748=CARTESIAN_POINT('Ctrl Pts',(9.65524877276325,638.12319788993,72.894594446214));
#103749=CARTESIAN_POINT('Ctrl Pts',(9.64562066556107,638.117588777634,72.9059620729246));
#103750=CARTESIAN_POINT('Ctrl Pts',(9.42731586112809,637.990409453907,73.1637082190586));
#103751=CARTESIAN_POINT('Ctrl Pts',(9.19804063693805,637.859784539816,73.4138743235853));
#103752=CARTESIAN_POINT('Ctrl Pts',(8.96066185930502,637.728380992124,73.6534663850734));
#103753=CARTESIAN_POINT('Ctrl Pts',(8.91843648227902,637.70500668546,73.6960854651346));
#103754=CARTESIAN_POINT('Ctrl Pts',(8.87595480168801,637.681607813329,73.738369934181));
#103755=CARTESIAN_POINT('Ctrl Pts',(8.83323308819527,637.658199473966,73.7803029115011));
#103756=CARTESIAN_POINT('Ctrl Pts',(8.82225322068705,637.652183318626,73.7910800666655));
#103757=CARTESIAN_POINT('Ctrl Pts',(8.8112573568705,637.646166453333,73.8018341562657));
#103758=CARTESIAN_POINT('Ctrl Pts',(8.80024576806366,637.640149131977,73.8125648963688));
#103759=CARTESIAN_POINT('Ctrl Pts',(8.45642397146976,637.452266504349,74.1476175763908));
#103760=CARTESIAN_POINT('Ctrl Pts',(8.09685247539544,637.263431908529,74.461195042532));
#103761=CARTESIAN_POINT('Ctrl Pts',(7.72053287787403,637.07685274923,74.75389752882));
#103762=CARTESIAN_POINT('Ctrl Pts',(7.4646028508242,636.949962707891,74.9529606542237));
#103763=CARTESIAN_POINT('Ctrl Pts',(7.20092632659578,636.824116856345,75.1423691924486));
#103764=CARTESIAN_POINT('Ctrl Pts',(6.92918660057919,636.700336265871,75.3223177033396));
#103765=CARTESIAN_POINT('Ctrl Pts',(6.91763580200828,636.695074743426,75.3299667469039));
#103766=CARTESIAN_POINT('Ctrl Pts',(6.90607038322277,636.689816954487,75.3375986977512));
#103767=CARTESIAN_POINT('Ctrl Pts',(6.89449031796739,636.684562976726,75.3452135726443));
#103768=CARTESIAN_POINT('Ctrl Pts',(6.56315230202816,636.534231995945,75.5630964155352));
#103769=CARTESIAN_POINT('Ctrl Pts',(6.21970864445252,636.387065880779,75.7668655454909));
#103770=CARTESIAN_POINT('Ctrl Pts',(5.8626639024424,636.245440217798,75.9560400598351));
#103771=CARTESIAN_POINT('Ctrl Pts',(5.85210062245606,636.241250178413,75.9616368468093));
#103772=CARTESIAN_POINT('Ctrl Pts',(5.84152543830141,636.237064998961,75.9672208471966));
#103773=CARTESIAN_POINT('Ctrl Pts',(5.83093831658855,636.232884744127,75.9727920447534));
#103774=CARTESIAN_POINT('Ctrl Pts',(5.51616734454452,636.108599512216,76.1384320853574));
#103775=CARTESIAN_POINT('Ctrl Pts',(5.19319897983501,635.989681238602,76.2913913409048));
#103776=CARTESIAN_POINT('Ctrl Pts',(4.863933133145,635.878703176547,76.4304781402202));
#103777=CARTESIAN_POINT('Ctrl Pts',(4.81686179178898,635.862837922697,76.4503617761166));
#103778=CARTESIAN_POINT('Ctrl Pts',(4.76966181406017,635.847134946092,76.4699619551446));
#103779=CARTESIAN_POINT('Ctrl Pts',(4.72233881323827,635.831601761893,76.4892752541631));
#103780=CARTESIAN_POINT('Ctrl Pts',(4.71410218547924,635.828898191664,76.4926367581263));
#103781=CARTESIAN_POINT('Ctrl Pts',(4.7058617639725,635.826199741836,76.495989600344));
#103782=CARTESIAN_POINT('Ctrl Pts',(4.69761757561058,635.823506451461,76.4993337633957));
#103783=CARTESIAN_POINT('Ctrl Pts',(4.33883025531642,635.706294375029,76.6448718378883));
#103784=CARTESIAN_POINT('Ctrl Pts',(3.97204499540476,635.598372180541,76.7746808977565));
#103785=CARTESIAN_POINT('Ctrl Pts',(3.59624449099713,635.502338704144,76.8878059230238));
#103786=CARTESIAN_POINT('Ctrl Pts',(3.23104131737279,635.40901330957,76.9977408958602));
#103787=CARTESIAN_POINT('Ctrl Pts',(2.85732420826786,635.326915434987,77.0919195272795));
#103788=CARTESIAN_POINT('Ctrl Pts',(2.4741421477009,635.258470242481,77.169441631003));
#103789=CARTESIAN_POINT('Ctrl Pts',(2.40382931954546,635.245910742562,77.1836667185483));
#103790=CARTESIAN_POINT('Ctrl Pts',(2.33319774590726,635.233811059836,77.1973308945058));
#103791=CARTESIAN_POINT('Ctrl Pts',(2.26224148372674,635.222186336159,77.2104285068931));
#103792=CARTESIAN_POINT('Origin',(28.,620.675373764374,64.2994740882088));
#103793=CARTESIAN_POINT('Ctrl Pts',(1.86306288877798,634.816577773823,79.840079036097));
#103794=CARTESIAN_POINT('Ctrl Pts',(2.1402114497942,634.853975948363,79.8060484936876));
#103795=CARTESIAN_POINT('Ctrl Pts',(2.41337614608207,634.898916808426,79.7649147909196));
#103796=CARTESIAN_POINT('Ctrl Pts',(2.68283184001296,634.950697211643,79.7169704303209));
#103797=CARTESIAN_POINT('Ctrl Pts',(2.97414735926638,635.006678344683,79.6651365421617));
#103798=CARTESIAN_POINT('Ctrl Pts',(3.26112767369113,635.070653432778,79.605341209851));
#103799=CARTESIAN_POINT('Ctrl Pts',(3.54412011469586,635.141683071731,79.5379106224164));
#103800=CARTESIAN_POINT('Ctrl Pts',(3.88187814635018,635.22645859067,79.457430654809));
#103801=CARTESIAN_POINT('Ctrl Pts',(4.21395546218051,635.321283246751,79.3660724895557));
#103802=CARTESIAN_POINT('Ctrl Pts',(4.54094258490074,635.424491558278,79.2643522128287));
#103803=CARTESIAN_POINT('Ctrl Pts',(4.66022073584993,635.462139819345,79.2272467561333));
#103804=CARTESIAN_POINT('Ctrl Pts',(4.7788215654647,635.500903092017,79.1887623167328));
#103805=CARTESIAN_POINT('Ctrl Pts',(4.89677373712177,635.540698981156,79.1489238821404));
#103806=CARTESIAN_POINT('Ctrl Pts',(5.16043615149924,635.62965605643,79.0598717036));
#103807=CARTESIAN_POINT('Ctrl Pts',(5.42147464015965,635.724158708811,78.9636635925424));
#103808=CARTESIAN_POINT('Ctrl Pts',(5.67881724162163,635.822969674527,78.8608748149905));
#103809=CARTESIAN_POINT('Ctrl Pts',(5.89134528490862,635.904573346361,78.7759860416554));
#103810=CARTESIAN_POINT('Ctrl Pts',(6.1013525895396,635.98911515618,78.686609180123));
#103811=CARTESIAN_POINT('Ctrl Pts',(6.30823535587315,636.075909817726,78.5930930229847));
#103812=CARTESIAN_POINT('Ctrl Pts',(6.60818034578659,636.201747384303,78.4575104256195));
#103813=CARTESIAN_POINT('Ctrl Pts',(6.90074477300754,636.33186003416,78.3137274985375));
#103814=CARTESIAN_POINT('Ctrl Pts',(7.1866141870702,636.465136951872,78.1619208948133));
#103815=CARTESIAN_POINT('Ctrl Pts',(7.33667046294903,636.535095600641,78.0822357921472));
#103816=CARTESIAN_POINT('Ctrl Pts',(7.48488204463925,636.605925993923,78.0003406744232));
#103817=CARTESIAN_POINT('Ctrl Pts',(7.63134808340531,636.677467493344,77.9162670025646));
#103818=CARTESIAN_POINT('Ctrl Pts',(7.91723728696255,636.817110392566,77.7521623726431));
#103819=CARTESIAN_POINT('Ctrl Pts',(8.19655198249425,636.959386851472,77.5798506235794));
#103820=CARTESIAN_POINT('Ctrl Pts',(8.46960770405218,637.103497273499,77.399123356496));
#103821=CARTESIAN_POINT('Ctrl Pts',(8.73947522321689,637.245925060239,77.2205062634905));
#103822=CARTESIAN_POINT('Ctrl Pts',(9.00322907486019,637.390143982264,77.0336684769876));
#103823=CARTESIAN_POINT('Ctrl Pts',(9.26117386904128,637.535339977012,76.8384370553729));
#103824=CARTESIAN_POINT('Ctrl Pts',(9.51911866322236,637.680535971759,76.6432056337581));
#103825=CARTESIAN_POINT('Ctrl Pts',(9.77125439994123,637.826708823744,76.4395799971643));
#103826=CARTESIAN_POINT('Ctrl Pts',(10.0178856892571,637.973005429087,76.2274241122122));
#103827=CARTESIAN_POINT('Ctrl Pts',(10.203587578906,638.083159968426,76.0676805985443));
#103828=CARTESIAN_POINT('Ctrl Pts',(10.3856411221024,638.193166844564,75.9034085015197));
#103829=CARTESIAN_POINT('Ctrl Pts',(10.5636740062097,638.302444690353,75.7349637390155));
#103830=CARTESIAN_POINT('Ctrl Pts',(10.7417068903169,638.411722536141,75.5665189765113));
#103831=CARTESIAN_POINT('Ctrl Pts',(10.9157191153351,638.520270922481,75.3939015342056));
#103832=CARTESIAN_POINT('Ctrl Pts',(11.0853383686276,638.627547204778,75.2175106217998));
#103833=CARTESIAN_POINT('Ctrl Pts',(11.2982866914253,638.762227106663,74.9960608263053));
#103834=CARTESIAN_POINT('Ctrl Pts',(11.5047763502784,638.895162465455,74.7682551816796));
#103835=CARTESIAN_POINT('Ctrl Pts',(11.7048608093241,639.02588366622,74.5338690056148));
#103836=CARTESIAN_POINT('Ctrl Pts',(11.823522007374,639.103408599278,74.3948649840589));
#103837=CARTESIAN_POINT('Ctrl Pts',(11.9399304013403,639.180153876557,74.2535467954849));
#103838=CARTESIAN_POINT('Ctrl Pts',(12.0540971431182,639.256013429961,74.1098707468977));
#103839=CARTESIAN_POINT('Ctrl Pts',(12.2247846330212,639.369428918167,73.8950647209866));
#103840=CARTESIAN_POINT('Ctrl Pts',(12.3904618758828,639.480866713069,73.6749899684775));
#103841=CARTESIAN_POINT('Ctrl Pts',(12.5510400004964,639.590004181669,73.449381692131));
#103842=CARTESIAN_POINT('Ctrl Pts',(12.6789711937418,639.676953052317,73.2696415434122));
#103843=CARTESIAN_POINT('Ctrl Pts',(12.8036658898911,639.76244096806,73.0863892069992));
#103844=CARTESIAN_POINT('Ctrl Pts',(12.9250791491289,639.846281360739,72.8994947227659));
#103845=CARTESIAN_POINT('Ctrl Pts',(13.0388387824086,639.924836638681,72.7243816575058));
#103846=CARTESIAN_POINT('Ctrl Pts',(13.149577296258,640.001877851171,72.5462085445932));
#103847=CARTESIAN_POINT('Ctrl Pts',(13.2569702277696,640.077040702749,72.3654131529155));
#103848=CARTESIAN_POINT('Ctrl Pts',(13.3632468260264,640.15142224787,72.1864971019469));
#103849=CARTESIAN_POINT('Ctrl Pts',(13.4662470340887,640.223964114305,72.0050131874289));
#103850=CARTESIAN_POINT('Ctrl Pts',(13.5656564024644,640.294356943015,71.821412137635));
#103851=CARTESIAN_POINT('Ctrl Pts',(13.6075769852428,640.324041352554,71.7439882174165));
#103852=CARTESIAN_POINT('Ctrl Pts',(13.6488590164015,640.353344153431,71.6661881202239));
#103853=CARTESIAN_POINT('Ctrl Pts',(13.6894789155558,640.382244612178,71.5880469506538));
#103854=CARTESIAN_POINT('Ctrl Pts',(13.8286010750807,640.481227975402,71.3204153591252));
#103855=CARTESIAN_POINT('Ctrl Pts',(13.960518022757,640.575774225862,71.0480331379661));
#103856=CARTESIAN_POINT('Ctrl Pts',(14.0849573496661,640.66553284446,70.7707639855962));
#103857=CARTESIAN_POINT('Ctrl Pts',(14.2077624538306,640.754112691205,70.4971361222502));
#103858=CARTESIAN_POINT('Ctrl Pts',(14.3232850500893,640.838029842505,70.2187485294791));
#103859=CARTESIAN_POINT('Ctrl Pts',(14.4312633215793,640.916900373456,69.9354880623769));
#103860=CARTESIAN_POINT('Ctrl Pts',(14.5371375665815,640.994234061078,69.6577471087608));
#103861=CARTESIAN_POINT('Ctrl Pts',(14.6357586344064,641.066715828707,69.3753210477021));
#103862=CARTESIAN_POINT('Ctrl Pts',(14.7268797169126,641.133938640373,69.0881248582813));
#103863=CARTESIAN_POINT('Ctrl Pts',(14.765817850058,641.162664493042,68.9653993247939));
#103864=CARTESIAN_POINT('Ctrl Pts',(14.8033864488709,641.190429470735,68.8418030398912));
#103865=CARTESIAN_POINT('Ctrl Pts',(14.8395662545944,641.217199266066,68.7173308130521));
#103866=CARTESIAN_POINT('Ctrl Pts',(14.9306676469202,641.28460608537,68.4039075388212));
#103867=CARTESIAN_POINT('Ctrl Pts',(15.0120041807898,641.344996930947,68.0882301956662));
#103868=CARTESIAN_POINT('Ctrl Pts',(15.0834994605392,641.398252513301,67.7702592069465));
#103869=CARTESIAN_POINT('Ctrl Pts',(15.1544872250653,641.45113005645,67.4545453618861));
#103870=CARTESIAN_POINT('Ctrl Pts',(15.2157729575024,641.496973294811,67.1365698743781));
#103871=CARTESIAN_POINT('Ctrl Pts',(15.2672818775681,641.535614532624,66.8162990868602));
#103872=CARTESIAN_POINT('Ctrl Pts',(15.3181640307078,641.573785579064,66.4999253939952));
#103873=CARTESIAN_POINT('Ctrl Pts',(15.3595058548198,641.604928781656,66.1813114971206));
#103874=CARTESIAN_POINT('Ctrl Pts',(15.391235266347,641.628832901803,65.860436342483));
#103875=CARTESIAN_POINT('Ctrl Pts',(15.399680349928,641.635195209922,65.7750323791085));
#103876=CARTESIAN_POINT('Ctrl Pts',(15.407444481865,641.641044422465,65.6894683089283));
#103877=CARTESIAN_POINT('Ctrl Pts',(15.414526303025,641.6463759616,65.6037439326523));
#103878=CARTESIAN_POINT('Ctrl Pts',(15.4364643525561,641.662891991443,65.3381871542066));
#103879=CARTESIAN_POINT('Ctrl Pts',(15.4517893452765,641.674443724131,65.0710724250625));
#103880=CARTESIAN_POINT('Ctrl Pts',(15.4603232031337,641.680876931242,64.8023554757184));
#103881=CARTESIAN_POINT('Ctrl Pts',(15.4648538948456,641.684292371084,64.6596915509598));
#103882=CARTESIAN_POINT('Ctrl Pts',(15.4674510190573,641.68626151627,64.5165142301015));
#103883=CARTESIAN_POINT('Ctrl Pts',(15.4681203454456,641.686765325652,64.3734851808154));
#103884=CARTESIAN_POINT('Ctrl Pts',(15.4687117396317,641.687210474604,64.2471095445317));
#103885=CARTESIAN_POINT('Ctrl Pts',(15.4677981227552,641.686512405933,64.1208497755977));
#103886=CARTESIAN_POINT('Ctrl Pts',(15.465383474685,641.684691870118,63.9951622171671));
#103887=CARTESIAN_POINT('Ctrl Pts',(15.4594523424331,641.680220063719,63.6864341914555));
#103888=CARTESIAN_POINT('Ctrl Pts',(15.444557626696,641.6689755171,63.3797508309682));
#103889=CARTESIAN_POINT('Ctrl Pts',(15.4209342345179,641.65118995091,63.0750606401239));
#103890=CARTESIAN_POINT('Ctrl Pts',(15.4035532438903,641.638104160481,62.8508838025451));
#103891=CARTESIAN_POINT('Ctrl Pts',(15.381447132351,641.621476462837,62.6277854531146));
#103892=CARTESIAN_POINT('Ctrl Pts',(15.3547094604652,641.60138204407,62.4057395605387));
#103893=CARTESIAN_POINT('Ctrl Pts',(15.3159115020446,641.572223842595,62.083537711986));
#103894=CARTESIAN_POINT('Ctrl Pts',(15.2673586125668,641.535768218365,61.7635549646432));
#103895=CARTESIAN_POINT('Ctrl Pts',(15.209136597126,641.49220316936,61.4457630820078));
#103896=CARTESIAN_POINT('Ctrl Pts',(15.1727005295007,641.464939615193,61.2468849353337));
#103897=CARTESIAN_POINT('Ctrl Pts',(15.1324776324191,641.434890687182,61.0488645460175));
#103898=CARTESIAN_POINT('Ctrl Pts',(15.0884889362004,641.402092265999,60.8516931877507));
#103899=CARTESIAN_POINT('Ctrl Pts',(15.0441618970615,641.36904157288,60.6530052686653));
#103900=CARTESIAN_POINT('Ctrl Pts',(14.9958796103505,641.333129102149,60.454790109615));
#103901=CARTESIAN_POINT('Ctrl Pts',(14.9437846854314,641.294465026022,60.2575526977022));
#103902=CARTESIAN_POINT('Ctrl Pts',(14.8915150909167,641.255671312726,60.0596539664951));
#103903=CARTESIAN_POINT('Ctrl Pts',(14.8354072484664,641.214107571676,59.8627397875055));
#103904=CARTESIAN_POINT('Ctrl Pts',(14.7756052067288,641.169936228604,59.667308030848));
#103905=CARTESIAN_POINT('Ctrl Pts',(14.7413494348752,641.144634024753,59.5553609221125));
#103906=CARTESIAN_POINT('Ctrl Pts',(14.7058815145681,641.118477144786,59.4438999846865));
#103907=CARTESIAN_POINT('Ctrl Pts',(14.6692285204308,641.091503479503,59.3330165540888));
#103908=CARTESIAN_POINT('Ctrl Pts',(14.5803938226745,641.026128263667,59.0642719051131));
#103909=CARTESIAN_POINT('Ctrl Pts',(14.4851858741749,640.956266144212,58.8001708828617));
#103910=CARTESIAN_POINT('Ctrl Pts',(14.3837715170968,640.882274341514,58.5405486633777));
#103911=CARTESIAN_POINT('Ctrl Pts',(14.2810607054585,640.807336647004,58.2776075014868));
#103912=CARTESIAN_POINT('Ctrl Pts',(14.1719837887646,640.728162967591,58.0192600662555));
#103913=CARTESIAN_POINT('Ctrl Pts',(14.0567140899262,640.645072609331,57.7653191294626));
#103914=CARTESIAN_POINT('Ctrl Pts',(13.9392204614165,640.560379166175,57.506478841064));
#103915=CARTESIAN_POINT('Ctrl Pts',(13.8152927875581,640.471616451942,57.2522164161331));
#103916=CARTESIAN_POINT('Ctrl Pts',(13.685114617953,640.379069406133,57.0023218326963));
#103917=CARTESIAN_POINT('Ctrl Pts',(13.602335492943,640.320219573649,56.8434161189011));
#103918=CARTESIAN_POINT('Ctrl Pts',(13.5170289340378,640.259838448468,56.6862763549364));
#103919=CARTESIAN_POINT('Ctrl Pts',(13.4292421368317,640.197988495442,56.5308469864962));
#103920=CARTESIAN_POINT('Ctrl Pts',(13.2697747250469,640.085636157255,56.248504767742));
#103921=CARTESIAN_POINT('Ctrl Pts',(13.1018986617114,639.968380260892,55.9716775249343));
#103922=CARTESIAN_POINT('Ctrl Pts',(12.9258526145704,639.846811878008,55.7006361644966));
#103923=CARTESIAN_POINT('Ctrl Pts',(12.828662025543,639.779697035435,55.55100105539));
#103924=CARTESIAN_POINT('Ctrl Pts',(12.7289813349122,639.711268159354,55.403128539522));
#103925=CARTESIAN_POINT('Ctrl Pts',(12.6268507021078,639.64162697107,55.2570578025761));
#103926=CARTESIAN_POINT('Ctrl Pts',(12.4693452509776,639.534226610603,55.0317880995707));
#103927=CARTESIAN_POINT('Ctrl Pts',(12.3071295901739,639.424692655522,54.8123661471315));
#103928=CARTESIAN_POINT('Ctrl Pts',(12.1402844332092,639.31338341686,54.5985128380537));
#103929=CARTESIAN_POINT('Ctrl Pts',(12.002978936203,639.221781295386,54.4225219047624));
#103930=CARTESIAN_POINT('Ctrl Pts',(11.8625381156246,639.128975808109,54.2503020731748));
#103931=CARTESIAN_POINT('Ctrl Pts',(11.7190069566274,639.035140454571,54.0816944827995));
#103932=CARTESIAN_POINT('Ctrl Pts',(11.5129986901229,638.900459883089,53.8396943648085));
#103933=CARTESIAN_POINT('Ctrl Pts',(11.3007022404411,638.763614383175,53.6050605705702));
#103934=CARTESIAN_POINT('Ctrl Pts',(11.0819551471624,638.625229473852,53.3776274956168));
#103935=CARTESIAN_POINT('Ctrl Pts',(10.8537269626186,638.480846587891,53.1403368554358));
#103936=CARTESIAN_POINT('Ctrl Pts',(10.6184768396454,638.33478826757,52.9108844662543));
#103937=CARTESIAN_POINT('Ctrl Pts',(10.3760202645821,638.187715079138,52.6890496920728));
#103938=CARTESIAN_POINT('Ctrl Pts',(10.1335636895188,638.040641890706,52.4672149178913));
#103939=CARTESIAN_POINT('Ctrl Pts',(9.88390066236547,637.892553766813,52.2529973474516));
#103940=CARTESIAN_POINT('Ctrl Pts',(9.62684666946167,637.744061124887,52.046149446617));
#103941=CARTESIAN_POINT('Ctrl Pts',(9.46346234490038,637.649678735689,51.9146762717287));
#103942=CARTESIAN_POINT('Ctrl Pts',(9.29686479133905,637.555081299247,51.7861174760067));
#103943=CARTESIAN_POINT('Ctrl Pts',(9.1275807697391,637.460801611946,51.6609035615571));
#103944=CARTESIAN_POINT('Ctrl Pts',(8.95353419623788,637.363869507129,51.5321669415345));
#103945=CARTESIAN_POINT('Ctrl Pts',(8.77664786888201,637.267273530126,51.406966138181));
#103946=CARTESIAN_POINT('Ctrl Pts',(8.59749427003405,637.171630477508,51.2857287611495));
#103947=CARTESIAN_POINT('Ctrl Pts',(8.54536693178636,637.143801744025,51.250452987727));
#103948=CARTESIAN_POINT('Ctrl Pts',(8.49304764555581,637.116053909166,51.2155125022222));
#103949=CARTESIAN_POINT('Ctrl Pts',(8.44055051338909,637.088402691147,51.1809172151339));
#103950=CARTESIAN_POINT('Ctrl Pts',(8.16409659561434,636.942789259763,50.9987357843133));
#103951=CARTESIAN_POINT('Ctrl Pts',(7.88203506759558,636.79939500734,50.8255502039267));
#103952=CARTESIAN_POINT('Ctrl Pts',(7.59396676190408,636.659228030904,50.6612756819119));
#103953=CARTESIAN_POINT('Ctrl Pts',(7.45646787272285,636.592324441793,50.5828652360158));
#103954=CARTESIAN_POINT('Ctrl Pts',(7.31760047037385,636.526155614565,50.5064843721738));
#103955=CARTESIAN_POINT('Ctrl Pts',(7.1773211472115,636.460828180361,50.4321209931152));
#103956=CARTESIAN_POINT('Ctrl Pts',(6.88018284129507,636.322452240901,50.274605202637));
#103957=CARTESIAN_POINT('Ctrl Pts',(6.57671769730352,636.187844122741,50.1261374141606));
#103958=CARTESIAN_POINT('Ctrl Pts',(6.26623698972816,636.058320110097,49.9869266312468));
#103959=CARTESIAN_POINT('Ctrl Pts',(6.12304923299931,635.998586115809,49.9227252840084));
#103960=CARTESIAN_POINT('Ctrl Pts',(5.97836935164948,635.939933327015,49.8604919927752));
#103961=CARTESIAN_POINT('Ctrl Pts',(5.83212979029488,635.882489700749,49.8002438368877));
#103962=CARTESIAN_POINT('Ctrl Pts',(5.60046097050222,635.791489037329,49.7048003123048));
#103963=CARTESIAN_POINT('Ctrl Pts',(5.36486309244537,635.70354017929,49.6143579168887));
#103964=CARTESIAN_POINT('Ctrl Pts',(5.12496004470658,635.619272900355,49.5291006468632));
#103965=CARTESIAN_POINT('Ctrl Pts',(4.92336015566138,635.548459818806,49.4574556371836));
#103966=CARTESIAN_POINT('Ctrl Pts',(4.71807804535173,635.480062142841,49.3892915169399));
#103967=CARTESIAN_POINT('Ctrl Pts',(4.51111271500933,635.415177638747,49.3254220404758));
#103968=CARTESIAN_POINT('Ctrl Pts',(4.47179014429899,635.402849846957,49.3132870998056));
#103969=CARTESIAN_POINT('Ctrl Pts',(4.43240681194781,635.390648970691,49.3013070706534));
#103970=CARTESIAN_POINT('Ctrl Pts',(4.39297642822443,635.378582662943,49.2894873770812));
#103971=CARTESIAN_POINT('Ctrl Pts',(4.12486075126194,635.29653511573,49.2091167378853));
#103972=CARTESIAN_POINT('Ctrl Pts',(3.85444033265441,635.220537807346,49.1359860390466));
#103973=CARTESIAN_POINT('Ctrl Pts',(3.58156371892505,635.151343123417,49.0702139584702));
#103974=CARTESIAN_POINT('Ctrl Pts',(3.32312890924843,635.08581051977,49.0079228192864));
#103975=CARTESIAN_POINT('Ctrl Pts',(3.06249100951263,635.026379694471,48.9522313546328));
#103976=CARTESIAN_POINT('Ctrl Pts',(2.79952136274532,634.973653473136,48.90326512778));
#103977=CARTESIAN_POINT('Ctrl Pts',(2.55448969638528,634.924523871932,48.8576390400981));
#103978=CARTESIAN_POINT('Ctrl Pts',(2.30743354479113,634.881215358141,48.8178516695863));
#103979=CARTESIAN_POINT('Ctrl Pts',(2.0582488241727,634.844182631359,48.7840331252826));
#103980=CARTESIAN_POINT('Ctrl Pts',(1.81685586891611,634.808307882149,48.7512720541715));
#103981=CARTESIAN_POINT('Ctrl Pts',(1.57346538001366,634.778322729849,48.7241119998909));
#103982=CARTESIAN_POINT('Ctrl Pts',(1.32798273535137,634.754607307784,48.7027040439557));
#103983=CARTESIAN_POINT('Ctrl Pts',(1.093192418537,634.731924842929,48.6822285404296));
#103984=CARTESIAN_POINT('Ctrl Pts',(0.855738997651462,634.715070446946,
48.6670981287459));
#103985=CARTESIAN_POINT('Ctrl Pts',(0.616984794805639,634.704331439349,
48.6574665592196));
#103986=CARTESIAN_POINT('Ctrl Pts',(0.386532831300444,634.693965861037,
48.6481699098516));
#103987=CARTESIAN_POINT('Ctrl Pts',(0.154868977576536,634.689297832698,
48.6439961961591));
#103988=CARTESIAN_POINT('Ctrl Pts',(-0.076781676442522,634.690552953027,
48.645119892231));
#103989=CARTESIAN_POINT('Ctrl Pts',(-0.145864683307238,634.690927255818,
48.6454550015954));
#103990=CARTESIAN_POINT('Ctrl Pts',(-0.21494651624892,634.691828105029,
48.6462614978511));
#103991=CARTESIAN_POINT('Ctrl Pts',(-0.283994682921353,634.693260874937,
48.6475446883329));
#103992=CARTESIAN_POINT('Ctrl Pts',(-0.520075952304442,634.698159631196,
48.6519320204288));
#103993=CARTESIAN_POINT('Ctrl Pts',(-0.755839055281249,634.709248379301,
48.6618612476738));
#103994=CARTESIAN_POINT('Ctrl Pts',(-0.990327191986353,634.726188034766,
48.67709682602));
#103995=CARTESIAN_POINT('Ctrl Pts',(-1.23740315666479,634.744037047402,
48.6931502830104));
#103996=CARTESIAN_POINT('Ctrl Pts',(-1.48306359503919,634.768381892692,
48.7150953295273));
#103997=CARTESIAN_POINT('Ctrl Pts',(-1.72618919815624,634.798786848871,
48.7426988494953));
#103998=CARTESIAN_POINT('Ctrl Pts',(-1.7805517045467,634.805585349742,48.7488709535905));
#103999=CARTESIAN_POINT('Ctrl Pts',(-1.83478747864479,634.81268669057,48.7553261113014));
#104000=CARTESIAN_POINT('Ctrl Pts',(-1.8888840075986,634.820085762158,48.7620619651124));
#104001=CARTESIAN_POINT('Ctrl Pts',(-0.252645464510396,637.415474030314,
76.9980210944396));
#104002=CARTESIAN_POINT('Ctrl Pts',(-1.11302381605652,637.42877366079,76.980488604498));
#104003=CARTESIAN_POINT('Ctrl Pts',(-1.94758251680077,637.509665462313,
76.8749778358584));
#104004=CARTESIAN_POINT('Ctrl Pts',(-3.16572559796507,637.712565815082,
76.5970874596841));
#104005=CARTESIAN_POINT('Ctrl Pts',(-3.56612249316459,637.793779472012,
76.4843247054231));
#104006=CARTESIAN_POINT('Ctrl Pts',(-4.35605342916383,637.979980203759,
76.2184083741727));
#104007=CARTESIAN_POINT('Ctrl Pts',(-4.74439125163809,638.08483946683,76.0653418396745));
#104008=CARTESIAN_POINT('Ctrl Pts',(-5.86615041872897,638.420465470767,
75.5582538330123));
#104009=CARTESIAN_POINT('Ctrl Pts',(-6.56690401319744,638.674272442424,
75.153793775975));
#104010=CARTESIAN_POINT('Ctrl Pts',(-7.55642794248227,639.075238610304,
74.4484723523538));
#104011=CARTESIAN_POINT('Ctrl Pts',(-7.87639888507424,639.212635032722,
74.1960774136137));
#104012=CARTESIAN_POINT('Ctrl Pts',(-8.48513868812207,639.485777362373,
73.6665189366011));
#104013=CARTESIAN_POINT('Ctrl Pts',(-8.77540631388641,639.622107542019,
73.3883947993268));
#104014=CARTESIAN_POINT('Ctrl Pts',(-9.32889245043522,639.891043814546,
72.8050737176796));
#104015=CARTESIAN_POINT('Ctrl Pts',(-9.59210827130408,640.023658956193,
72.4998783443379));
#104016=CARTESIAN_POINT('Ctrl Pts',(-10.0915350771624,640.28212906445,71.8610821467425));
#104017=CARTESIAN_POINT('Ctrl Pts',(-10.3287739497107,640.408558271658,
71.525776856965));
#104018=CARTESIAN_POINT('Ctrl Pts',(-10.9894725080146,640.768129166215,
70.4882632613146));
#104019=CARTESIAN_POINT('Ctrl Pts',(-11.3625914305347,640.981504678687,
69.7564109606946));
#104020=CARTESIAN_POINT('Ctrl Pts',(-11.818404938002,641.247406419786,68.5929331071031));
#104021=CARTESIAN_POINT('Ctrl Pts',(-11.9534576443998,641.327342492746,
68.1916750120165));
#104022=CARTESIAN_POINT('Ctrl Pts',(-12.182174157639,641.463778556434,67.3809131335881));
#104023=CARTESIAN_POINT('Ctrl Pts',(-12.276307508626,641.520542453502,66.9709644805429));
#104024=CARTESIAN_POINT('Ctrl Pts',(-12.4242394369779,641.610119675406,
66.1418454500847));
#104025=CARTESIAN_POINT('Ctrl Pts',(-12.4780399075043,641.642936469747,
65.7226757432849));
#104026=CARTESIAN_POINT('Ctrl Pts',(-12.5441585218638,641.683305659608,
64.8747881241364));
#104027=CARTESIAN_POINT('Ctrl Pts',(-12.5562467120334,641.690716433489,
64.4432644779558));
#104028=CARTESIAN_POINT('Ctrl Pts',(-12.5282315834883,641.673580507606,
63.1661747786782));
#104029=CARTESIAN_POINT('Ctrl Pts',(-12.4261421803805,641.610839125609,
62.3315318096105));
#104030=CARTESIAN_POINT('Ctrl Pts',(-12.1532157238051,641.446489533143,
61.1033176255798));
#104031=CARTESIAN_POINT('Ctrl Pts',(-12.0418922330986,641.379825623817,
60.6972107540752));
#104032=CARTESIAN_POINT('Ctrl Pts',(-11.7789498235242,641.224316920002,
59.8958888312612));
#104033=CARTESIAN_POINT('Ctrl Pts',(-11.6297082784345,641.136886271958,
59.5076325746472));
#104034=CARTESIAN_POINT('Ctrl Pts',(-11.1319937919119,640.849938512318,
58.3769969850098));
#104035=CARTESIAN_POINT('Ctrl Pts',(-10.7340829199422,640.625798126202,
57.6684452447755));
#104036=CARTESIAN_POINT('Ctrl Pts',(-10.040023576069,640.255218646015,56.6679468437341));
#104037=CARTESIAN_POINT('Ctrl Pts',(-9.79091798691913,640.125241864666,
56.3433436698442));
#104038=CARTESIAN_POINT('Ctrl Pts',(-9.26667744604236,639.860382199086,
55.7243454178727));
#104039=CARTESIAN_POINT('Ctrl Pts',(-8.99185892776024,639.725615805067,
55.4299091303579));
#104040=CARTESIAN_POINT('Ctrl Pts',(-8.1292937094432,639.319056101314,54.5894500217195));
#104041=CARTESIAN_POINT('Ctrl Pts',(-7.5038764230366,639.044668394762,54.0856572853192));
#104042=CARTESIAN_POINT('Ctrl Pts',(-6.14010017594243,638.518378987584,
53.1918099095666));
#104043=CARTESIAN_POINT('Ctrl Pts',(-5.42038031899213,638.273835975921,
52.8139552665562));
#104044=CARTESIAN_POINT('Ctrl Pts',(-4.27629107737484,637.959970371973,
52.3511891253608));
#104045=CARTESIAN_POINT('Ctrl Pts',(-3.88308899204296,637.864026388571,
52.2141438459509));
#104046=CARTESIAN_POINT('Ctrl Pts',(-3.07656099875632,637.695968083433,
51.9785830844804));
#104047=CARTESIAN_POINT('Ctrl Pts',(-2.66897700762064,637.625031584555,
51.8816585325753));
#104048=CARTESIAN_POINT('Ctrl Pts',(-1.84491113503772,637.512268879597,
51.7291914233704));
#104049=CARTESIAN_POINT('Ctrl Pts',(-1.42842899531872,637.470445472889,
51.67364863131));
#104050=CARTESIAN_POINT('Ctrl Pts',(-0.586133086793797,637.418625085894,
51.6050092571627));
#104051=CARTESIAN_POINT('Ctrl Pts',(-0.159088542674411,637.408657678832,
51.5919408760206));
#104052=CARTESIAN_POINT('Ctrl Pts',(0.270210553101167,637.415754985731,
51.6012974652903));
#104053=CARTESIAN_POINT('Ctrl Pts',(0.422698892023407,637.418949661958,
51.6054949190759));
#104054=CARTESIAN_POINT('Ctrl Pts',(0.401375821438588,637.722772699625,
52.0060233138173));
#104055=CARTESIAN_POINT('Ctrl Pts',(0.414276434700987,637.21974803095,52.0064418924399));
#104056=CARTESIAN_POINT('Ctrl Pts',(-0.485687802890622,637.395421830215,
51.5746539347076));
#104057=CARTESIAN_POINT('Ctrl Pts',(-0.464187114878885,637.702785894513,
51.9782978993784));
#104058=CARTESIAN_POINT('Ctrl Pts',(-0.476010708084271,637.196500386218,
51.9765750164005));
#104059=CARTESIAN_POINT('Ctrl Pts',(-1.37343881346729,637.448508508017,
51.6430377951267));
#104060=CARTESIAN_POINT('Ctrl Pts',(-1.28833508012202,637.745869850797,
52.037024971321));
#104061=CARTESIAN_POINT('Ctrl Pts',(-1.3460709313523,637.248954683656,52.0427987467284));
#104062=CARTESIAN_POINT('Ctrl Pts',(-2.65150548283939,637.622235142896,
51.8778512479119));
#104063=CARTESIAN_POINT('Ctrl Pts',(-2.52264148011033,637.898282658345,
52.2542948909666));
#104064=CARTESIAN_POINT('Ctrl Pts',(-2.59867283526968,637.420612734044,
52.2701959516384));
#104065=CARTESIAN_POINT('Ctrl Pts',(-3.05701248764582,637.692361961531,
51.9736219146518));
#104066=CARTESIAN_POINT('Ctrl Pts',(-2.9104992780375,637.959022674606,52.3416256351175));
#104067=CARTESIAN_POINT('Ctrl Pts',(-2.99609991422878,637.489904443202,
52.3629416887653));
#104068=CARTESIAN_POINT('Ctrl Pts',(-3.85966274491754,637.858622815906,
52.2064814361353));
#104069=CARTESIAN_POINT('Ctrl Pts',(-3.68456306759803,638.105545872289,
52.5572384796229));
#104070=CARTESIAN_POINT('Ctrl Pts',(-3.78275735662804,637.654185523528,
52.5884464824649));
#104071=CARTESIAN_POINT('Ctrl Pts',(-4.2516957080172,637.953733553696,52.342197416409));
#104072=CARTESIAN_POINT('Ctrl Pts',(-4.06360822860176,638.189474882183,
52.6827304516184));
#104073=CARTESIAN_POINT('Ctrl Pts',(-4.166979050703,637.748163685361,52.7198758782938));
#104074=CARTESIAN_POINT('Ctrl Pts',(-5.39252319671764,638.265104382238,
52.8006937061185));
#104075=CARTESIAN_POINT('Ctrl Pts',(-5.15820380454856,638.464354488508,
53.106143986478));
#104076=CARTESIAN_POINT('Ctrl Pts',(-5.28507434996358,638.055826516981,
53.1638902156519));
#104077=CARTESIAN_POINT('Ctrl Pts',(-6.11111639604367,638.508142463439,
53.1755283868842));
#104078=CARTESIAN_POINT('Ctrl Pts',(-5.8622172477199,638.682290229399,53.4546201335385));
#104079=CARTESIAN_POINT('Ctrl Pts',(-5.98934985904857,638.295970472941,
53.5268853366489));
#104080=CARTESIAN_POINT('Ctrl Pts',(-7.47414788157404,639.032208675362,
54.0634384892155));
#104081=CARTESIAN_POINT('Ctrl Pts',(-7.20845486530066,639.164782335859,
54.3026771532069));
#104082=CARTESIAN_POINT('Ctrl Pts',(-7.32522403708878,638.813796828574,
54.3867510931747));
#104083=CARTESIAN_POINT('Ctrl Pts',(-8.10110508190111,639.306397424697,
54.5652847276252));
#104084=CARTESIAN_POINT('Ctrl Pts',(-7.83452284189272,639.419779216059,
54.7821223431411));
#104085=CARTESIAN_POINT('Ctrl Pts',(-7.93969011684976,639.084720971824,
54.8727462625326));
#104086=CARTESIAN_POINT('Ctrl Pts',(-8.96598822614474,639.713072351722,
55.4030453263832));
#104087=CARTESIAN_POINT('Ctrl Pts',(-8.70809531403378,639.8065991219,55.6034482729444));
#104088=CARTESIAN_POINT('Ctrl Pts',(-8.78734281065214,639.486554596994,
55.6840474437807));
#104089=CARTESIAN_POINT('Ctrl Pts',(-9.24171805717354,639.847996124981,
55.6967061098111));
#104090=CARTESIAN_POINT('Ctrl Pts',(-8.98356312241736,639.933680039658,
55.887647513816));
#104091=CARTESIAN_POINT('Ctrl Pts',(-9.05757910582421,639.619871964218,
55.9684328676933));
#104092=CARTESIAN_POINT('Ctrl Pts',(-9.76801292518633,640.113392489719,
56.3144572329125));
#104093=CARTESIAN_POINT('Ctrl Pts',(-9.50901929974678,640.184197151179,
56.4871657754348));
#104094=CARTESIAN_POINT('Ctrl Pts',(-9.57338818638589,639.882108498261,
56.5666721248706));
#104095=CARTESIAN_POINT('Ctrl Pts',(-10.0185033275,640.243874592087,56.6388958448344));
#104096=CARTESIAN_POINT('Ctrl Pts',(-9.7600322735385,640.307954662928,56.8025965430298));
#104097=CARTESIAN_POINT('Ctrl Pts',(-9.8188879556435,640.011037106482,56.8808632052432));
#104098=CARTESIAN_POINT('Ctrl Pts',(-10.716727326934,640.616151015162,57.6394451240119));
#104099=CARTESIAN_POINT('Ctrl Pts',(-10.4506899105479,640.65724880266,57.7657813921744));
#104100=CARTESIAN_POINT('Ctrl Pts',(-10.5031997469232,640.378880679238,
57.8498081873022));
#104101=CARTESIAN_POINT('Ctrl Pts',(-11.1175203099313,640.841694041044,
58.3487305133394));
#104102=CARTESIAN_POINT('Ctrl Pts',(-10.8571731765776,640.874517949965,
58.4602774988305));
#104103=CARTESIAN_POINT('Ctrl Pts',(-10.8960080548356,640.601738696694,
58.5366905083561));
#104104=CARTESIAN_POINT('Ctrl Pts',(-11.619394535175,641.130841438184,59.4818150157709));
#104105=CARTESIAN_POINT('Ctrl Pts',(-11.3646047806954,641.153135988497,
59.5771443494444));
#104106=CARTESIAN_POINT('Ctrl Pts',(-11.3878836354649,640.887443837893,
59.6339866130622));
#104107=CARTESIAN_POINT('Ctrl Pts',(-11.7699948379489,641.219020908331,
59.8711153341678));
#104108=CARTESIAN_POINT('Ctrl Pts',(-11.5161693648167,641.237777958691,
59.9583961633857));
#104109=CARTESIAN_POINT('Ctrl Pts',(-11.5354834909803,640.974573487447,
60.0109905179452));
#104110=CARTESIAN_POINT('Ctrl Pts',(-12.0355183921279,641.375990158675,
60.6750733074951));
#104111=CARTESIAN_POINT('Ctrl Pts',(-11.7825939140218,641.388123439216,
60.7452930450769));
#104112=CARTESIAN_POINT('Ctrl Pts',(-11.7957168424692,641.129673875916,
60.7895545484208));
#104113=CARTESIAN_POINT('Ctrl Pts',(-12.1481703593011,641.443430005107,
61.0832468504235));
#104114=CARTESIAN_POINT('Ctrl Pts',(-11.8961009417762,641.453030580109,
61.145720101883));
#104115=CARTESIAN_POINT('Ctrl Pts',(-11.9061244276539,641.196310824918,
61.1848355228865));
#104116=CARTESIAN_POINT('Ctrl Pts',(-12.4242303319733,641.609632067201,
62.3171054077186));
#104117=CARTESIAN_POINT('Ctrl Pts',(-12.1719915811263,641.611765497776,
62.3490805674734));
#104118=CARTESIAN_POINT('Ctrl Pts',(-12.1766841067953,641.360534000301,
62.3797203320405));
#104119=CARTESIAN_POINT('Ctrl Pts',(-12.5276874182953,641.673215309511,
63.1559355922065));
#104120=CARTESIAN_POINT('Ctrl Pts',(-12.2775058411409,641.673796783702,
63.1776792731061));
#104121=CARTESIAN_POINT('Ctrl Pts',(-12.2780801673297,641.423360360423,
63.1920557640221));
#104122=CARTESIAN_POINT('Ctrl Pts',(-12.5564129571305,641.690785777535,
64.4400267385226));
#104123=CARTESIAN_POINT('Ctrl Pts',(-12.3063643128568,641.69068276132,64.4370638410256));
#104124=CARTESIAN_POINT('Ctrl Pts',(-12.3062333905587,641.440721636806,
64.4355871579955));
#104125=CARTESIAN_POINT('Ctrl Pts',(-12.5443205872794,641.683372183581,
64.8740772469317));
#104126=CARTESIAN_POINT('Ctrl Pts',(-12.2941718209377,641.68353116687,64.8634434416355));
#104127=CARTESIAN_POINT('Ctrl Pts',(-12.2943819383328,641.433396304253,
64.8559276849426));
#104128=CARTESIAN_POINT('Ctrl Pts',(-12.4777330003823,641.64271664739,65.7266035670265));
#104129=CARTESIAN_POINT('Ctrl Pts',(-12.2273094971991,641.644483451026,
65.6991136324248));
#104130=CARTESIAN_POINT('Ctrl Pts',(-12.2291210200655,641.393224809202,
65.6815257693198));
#104131=CARTESIAN_POINT('Ctrl Pts',(-12.4234779559463,641.609622661129,
66.1479562446186));
#104132=CARTESIAN_POINT('Ctrl Pts',(-12.1726163502219,641.612576505469,
66.1128812981191));
#104133=CARTESIAN_POINT('Ctrl Pts',(-12.1759469061432,641.360524818572,
66.0895695514284));
#104134=CARTESIAN_POINT('Ctrl Pts',(-12.2742573339491,641.519271348643,
66.9811892328191));
#104135=CARTESIAN_POINT('Ctrl Pts',(-12.0228067561347,641.525859578493,
66.9293351464561));
#104136=CARTESIAN_POINT('Ctrl Pts',(-12.0296993061205,641.271249220213,
66.896483765114));
#104137=CARTESIAN_POINT('Ctrl Pts',(-12.1792897304192,641.462010453369,
67.393068477219));
#104138=CARTESIAN_POINT('Ctrl Pts',(-11.9271007354986,641.470712297851,
67.3335484589464));
#104139=CARTESIAN_POINT('Ctrl Pts',(-11.9366237554634,641.214670037509,
67.2953533735953));
#104140=CARTESIAN_POINT('Ctrl Pts',(-11.9485583932798,641.324400942808,
68.20744886739));
#104141=CARTESIAN_POINT('Ctrl Pts',(-11.6955378132595,641.338808940148,
68.130976713246));
#104142=CARTESIAN_POINT('Ctrl Pts',(-11.7104894329877,641.078698892736,
68.0840105657425));
#104143=CARTESIAN_POINT('Ctrl Pts',(-11.8123667673948,641.243813984238,
68.6102326743059));
#104144=CARTESIAN_POINT('Ctrl Pts',(-11.5583984649845,641.261357597934,
68.5257596552219));
#104145=CARTESIAN_POINT('Ctrl Pts',(-11.5770111802493,640.999071358111,
68.474072058525));
#104146=CARTESIAN_POINT('Ctrl Pts',(-11.3530417450549,640.975973416792,
69.7773368489012));
#104147=CARTESIAN_POINT('Ctrl Pts',(-11.094177851908,641.003183187458,69.6760041353329));
#104148=CARTESIAN_POINT('Ctrl Pts',(-11.1268371472754,640.734419412521,
69.6043131395056));
#104149=CARTESIAN_POINT('Ctrl Pts',(-10.9773436374481,640.761257671499,
70.5106549236237));
#104150=CARTESIAN_POINT('Ctrl Pts',(-10.7127265394219,640.795865883309,
70.3951256963504));
#104151=CARTESIAN_POINT('Ctrl Pts',(-10.7586237260962,640.522259749011,
70.3144690681693));
#104152=CARTESIAN_POINT('Ctrl Pts',(-10.3128000119404,640.399951370545,
71.5492638109213));
#104153=CARTESIAN_POINT('Ctrl Pts',(-10.0546064812974,640.45606535248,71.3965629016389));
#104154=CARTESIAN_POINT('Ctrl Pts',(-10.1073211782066,640.165255645638,
71.3202714227271));
#104155=CARTESIAN_POINT('Ctrl Pts',(-10.0744570782856,640.273083587572,
71.8844906020682));
#104156=CARTESIAN_POINT('Ctrl Pts',(-9.81559960598111,640.335484419032,
71.722883385682));
#104157=CARTESIAN_POINT('Ctrl Pts',(-9.87372685329524,640.039898320491,
71.6449099002616));
#104158=CARTESIAN_POINT('Ctrl Pts',(-9.5730180198315,640.013923785954,72.5228060041743));
#104159=CARTESIAN_POINT('Ctrl Pts',(-9.31451031820139,640.090283649802,
72.3432405042314));
#104160=CARTESIAN_POINT('Ctrl Pts',(-9.38227834633797,639.783824086546,
72.2630638437438));
#104161=CARTESIAN_POINT('Ctrl Pts',(-9.30888880145443,639.881056246463,
72.827584871394));
#104162=CARTESIAN_POINT('Ctrl Pts',(-9.05028270509328,639.96475736298,72.6387917490736));
#104163=CARTESIAN_POINT('Ctrl Pts',(-9.12341151926098,639.652538458904,
72.5582161648588));
#104164=CARTESIAN_POINT('Ctrl Pts',(-8.75381487614663,639.611825072234,
73.40978275451));
#104165=CARTESIAN_POINT('Ctrl Pts',(-8.49692150109578,639.711562811131,
73.2025036527718));
#104166=CARTESIAN_POINT('Ctrl Pts',(-8.57939679683925,639.386512790825,
73.1220252238533));
#104167=CARTESIAN_POINT('Ctrl Pts',(-8.46287263080748,639.475452444918,
73.6871999316855));
#104168=CARTESIAN_POINT('Ctrl Pts',(-8.2067446500672,639.583671139382,73.4702530911214));
#104169=CARTESIAN_POINT('Ctrl Pts',(-8.29425119061942,639.251763833223,
73.3906801363316));
#104170=CARTESIAN_POINT('Ctrl Pts',(-7.85308898859091,639.202454098524,
74.2151005589185));
#104171=CARTESIAN_POINT('Ctrl Pts',(-7.60084562786785,639.328898689758,
73.978892784628));
#104172=CARTESIAN_POINT('Ctrl Pts',(-7.69661684926344,638.982015887313,
73.9019070495361));
#104173=CARTESIAN_POINT('Ctrl Pts',(-7.53269227808987,639.065231345536,
74.4665545912258));
#104174=CARTESIAN_POINT('Ctrl Pts',(-7.28274092847238,639.201467950777,
74.2199817961026));
#104175=CARTESIAN_POINT('Ctrl Pts',(-7.3826036898993,638.84642696737,74.1454188990161));
#104176=CARTESIAN_POINT('Ctrl Pts',(-6.54436688094676,638.665837118865,
75.1676209958109));
#104177=CARTESIAN_POINT('Ctrl Pts',(-6.28966522125244,638.826499839077,
74.9017755309047));
#104178=CARTESIAN_POINT('Ctrl Pts',(-6.41396819947268,638.45178748053,74.8243434255003));
#104179=CARTESIAN_POINT('Ctrl Pts',(-5.84677300034356,638.414131609539,
75.5680603372253));
#104180=CARTESIAN_POINT('Ctrl Pts',(-5.60308614276541,638.598811561366,
75.2765310704285));
#104181=CARTESIAN_POINT('Ctrl Pts',(-5.73027341984355,638.20307921196,75.2121345157478));
#104182=CARTESIAN_POINT('Ctrl Pts',(-4.735123634144,638.082280084104,76.0690872002211));
#104183=CARTESIAN_POINT('Ctrl Pts',(-4.53330991520824,638.304130947767,
75.7410809439269));
#104184=CARTESIAN_POINT('Ctrl Pts',(-4.64077478504796,637.875179554541,
75.6973360141623));
#104185=CARTESIAN_POINT('Ctrl Pts',(-4.35360434329439,637.979334203798,
76.2193388306527));
#104186=CARTESIAN_POINT('Ctrl Pts',(-4.16281829720205,638.212579524345,
75.8808099165903));
#104187=CARTESIAN_POINT('Ctrl Pts',(-4.26685720707408,637.773459525923,
75.8428419591479));
#104188=CARTESIAN_POINT('Ctrl Pts',(-3.56604570114688,637.793748701365,
76.4843606975452));
#104189=CARTESIAN_POINT('Ctrl Pts',(-3.40047115190969,638.047948850038,
76.127370335997));
#104190=CARTESIAN_POINT('Ctrl Pts',(-3.49499057985149,637.590083879434,
76.0994932686235));
#104191=CARTESIAN_POINT('Ctrl Pts',(-3.16152317445562,637.71170299198,76.5982831453345));
#104192=CARTESIAN_POINT('Ctrl Pts',(-3.01184896420212,637.976344024389,
76.2318455359098));
#104193=CARTESIAN_POINT('Ctrl Pts',(-3.09852828926658,637.509015197064,
76.2098174680871));
#104194=CARTESIAN_POINT('Ctrl Pts',(-1.89224989733331,637.500669633967,
76.887268497963));
#104195=CARTESIAN_POINT('Ctrl Pts',(-1.77973073550203,637.789819969329,
76.5008366075363));
#104196=CARTESIAN_POINT('Ctrl Pts',(-1.85454421885567,637.300494574968,
76.4896756819702));
#104197=CARTESIAN_POINT('Ctrl Pts',(-1.0083393223673,637.41933676935,76.9927644491279));
#104198=CARTESIAN_POINT('Ctrl Pts',(-0.956219519798643,637.723350752829,
76.5919508447244));
#104199=CARTESIAN_POINT('Ctrl Pts',(-0.988247314567113,637.220130545011,
76.5918392124773));
#104200=CARTESIAN_POINT('Ctrl Pts',(-0.100242643464739,637.413790050648,
77.0002550481953));
#104201=CARTESIAN_POINT('Ctrl Pts',(-0.0952647791071383,637.71834699738,
76.5990988612787));
#104202=CARTESIAN_POINT('Ctrl Pts',(-0.098245300777777,637.214649861766,
76.5990932436941));
#104203=CARTESIAN_POINT('Ctrl Pts',(-3.14894350550333,635.052705176108,
48.9762189006802));
#104204=CARTESIAN_POINT('Ctrl Pts',(-3.17805581581006,634.981774591649,
48.9095429264701));
#104205=CARTESIAN_POINT('Ctrl Pts',(-3.19988829483125,634.881466988651,
48.9136642378198));
#104206=CARTESIAN_POINT('Ctrl Pts',(-2.26217542759882,634.844413884159,
48.7825198376226));
#104207=CARTESIAN_POINT('Ctrl Pts',(-2.28874499765809,634.773843548207,
48.7179545738432));
#104208=CARTESIAN_POINT('Ctrl Pts',(-2.2988111695793,634.675657800926,48.7191843934846));
#104209=CARTESIAN_POINT('Ctrl Pts',(-1.27865210597201,634.714844669714,
48.6668762937005));
#104210=CARTESIAN_POINT('Ctrl Pts',(-1.29103235742706,634.643610831895,
48.6027815718824));
#104211=CARTESIAN_POINT('Ctrl Pts',(-1.29934864835061,634.547626991756,
48.6030696395671));
#104212=CARTESIAN_POINT('Ctrl Pts',(0.242130489444798,634.682105481683,
48.6375535275712));
#104213=CARTESIAN_POINT('Ctrl Pts',(0.244224674588167,634.610876552288,
48.5737334451187));
#104214=CARTESIAN_POINT('Ctrl Pts',(0.24604904762521,634.515277216675,48.5736280341214));
#104215=CARTESIAN_POINT('Ctrl Pts',(0.781040459010377,634.702757772588,
48.6559104137994));
#104216=CARTESIAN_POINT('Ctrl Pts',(0.788931574693899,634.631577480282,
48.5919652205538));
#104217=CARTESIAN_POINT('Ctrl Pts',(0.793683375382584,634.535683985946,
48.5920594319863));
#104218=CARTESIAN_POINT('Ctrl Pts',(2.35874810817493,634.852789214134,48.791311990248));
#104219=CARTESIAN_POINT('Ctrl Pts',(2.38338099377123,634.781749974576,48.7262413336859));
#104220=CARTESIAN_POINT('Ctrl Pts',(2.39693158170349,634.683931291769,48.7280101254697));
#104221=CARTESIAN_POINT('Ctrl Pts',(3.37298184661552,635.068933230022,48.9865958531244));
#104222=CARTESIAN_POINT('Ctrl Pts',(3.41253860309941,634.999941019321,48.9217203889832));
#104223=CARTESIAN_POINT('Ctrl Pts',(3.42759398731837,634.897509402095,48.9240904248496));
#104224=CARTESIAN_POINT('Ctrl Pts',(4.60280256700872,635.442476264948,49.351977573634));
#104225=CARTESIAN_POINT('Ctrl Pts',(4.64765158093338,635.37152943939,49.2817265518851));
#104226=CARTESIAN_POINT('Ctrl Pts',(4.67730317816144,635.266604909258,49.2909483904667));
#104227=CARTESIAN_POINT('Ctrl Pts',(4.84718746008067,635.522512124264,49.4313666860681));
#104228=CARTESIAN_POINT('Ctrl Pts',(4.89464885506356,635.451676187017,49.3604691881232));
#104229=CARTESIAN_POINT('Ctrl Pts',(4.92564398215479,635.345689107181,49.3706595461052));
#104230=CARTESIAN_POINT('Ctrl Pts',(5.32584062015199,635.689537216775,49.6000512954552));
#104231=CARTESIAN_POINT('Ctrl Pts',(5.37840998526045,635.618886104377,49.5277111330022));
#104232=CARTESIAN_POINT('Ctrl Pts',(5.41204506061927,635.510728093336,49.5400282810896));
#104233=CARTESIAN_POINT('Ctrl Pts',(5.56095277341081,635.776762458102,49.6895734166027));
#104234=CARTESIAN_POINT('Ctrl Pts',(5.61612178002954,635.706265107494,49.6165277399625));
#104235=CARTESIAN_POINT('Ctrl Pts',(5.65096311005464,635.596916271685,49.6299136263926));
#104236=CARTESIAN_POINT('Ctrl Pts',(6.25472898600255,636.04770447283,49.973139660512));
#104237=CARTESIAN_POINT('Ctrl Pts',(6.31941936621702,635.978335899727,49.8984892971421));
#104238=CARTESIAN_POINT('Ctrl Pts',(6.35597407519104,635.864638452226,49.914631946893));
#104239=CARTESIAN_POINT('Ctrl Pts',(6.70189742601776,636.240627504047,50.1821258540263));
#104240=CARTESIAN_POINT('Ctrl Pts',(6.77205222396553,636.171955285493,50.1062416227097));
#104241=CARTESIAN_POINT('Ctrl Pts',(6.81038188975856,636.05526856269,50.1244671165347));
#104242=CARTESIAN_POINT('Ctrl Pts',(7.56968515550765,636.642919469563,50.6387960920349));
#104243=CARTESIAN_POINT('Ctrl Pts',(7.65049736475119,636.575382508907,50.5595723308578));
#104244=CARTESIAN_POINT('Ctrl Pts',(7.69221803306948,636.452778493096,50.5829910891641));
#104245=CARTESIAN_POINT('Ctrl Pts',(7.99028738530131,636.852312016469,50.8864885495721));
#104246=CARTESIAN_POINT('Ctrl Pts',(8.07671976444589,636.785759599221,50.8060183026103));
#104247=CARTESIAN_POINT('Ctrl Pts',(8.11963001506569,636.659682895894,50.831690360471));
#104248=CARTESIAN_POINT('Ctrl Pts',(8.80740286369044,637.281161742136,51.4212246124972));
#104249=CARTESIAN_POINT('Ctrl Pts',(8.90504619960573,637.216475096936,51.3374439703381));
#104250=CARTESIAN_POINT('Ctrl Pts',(8.94997490797288,637.083436369467,51.3685986628816));
#104251=CARTESIAN_POINT('Ctrl Pts',(9.20548162083383,637.501580052554,51.7096442401456));
#104252=CARTESIAN_POINT('Ctrl Pts',(9.30897039084119,637.438216925406,51.6247044118637));
#104253=CARTESIAN_POINT('Ctrl Pts',(9.35449918700437,637.301236129998,51.658191408593));
#104254=CARTESIAN_POINT('Ctrl Pts',(10.3487844505047,638.160185666631,52.6234603889831));
#104255=CARTESIAN_POINT('Ctrl Pts',(10.4792441450531,638.106209094922,52.541391505325));
#104256=CARTESIAN_POINT('Ctrl Pts',(10.5163351536716,637.952029241467,52.575739049541));
#104257=CARTESIAN_POINT('Ctrl Pts',(11.0469172883128,638.596769704622,53.2977962975319));
#104258=CARTESIAN_POINT('Ctrl Pts',(11.1886816147118,638.54672121981,53.2166715576217));
#104259=CARTESIAN_POINT('Ctrl Pts',(11.2257713012345,638.383429089509,53.2528256613287));
#104260=CARTESIAN_POINT('Ctrl Pts',(12.004918884179,639.222046706336,54.4157870888981));
#104261=CARTESIAN_POINT('Ctrl Pts',(12.1575997879902,639.173534897356,54.3239043685374));
#104262=CARTESIAN_POINT('Ctrl Pts',(12.1992715391054,639.001272383721,54.3753501795627));
#104263=CARTESIAN_POINT('Ctrl Pts',(12.3091950227284,639.425602760796,54.8063260024279));
#104264=CARTESIAN_POINT('Ctrl Pts',(12.4682176936469,639.379586655534,54.7148446167707));
#104265=CARTESIAN_POINT('Ctrl Pts',(12.5084759793438,639.202412549241,54.7674817836186));
#104266=CARTESIAN_POINT('Ctrl Pts',(12.8866359918317,639.818864013947,55.6266595150129));
#104267=CARTESIAN_POINT('Ctrl Pts',(13.0590920906577,639.778506365938,55.5364326108684));
#104268=CARTESIAN_POINT('Ctrl Pts',(13.0952716020131,639.591007890039,55.5911613762021));
#104269=CARTESIAN_POINT('Ctrl Pts',(13.156552724659,640.006361596555,56.0520433785381));
#104270=CARTESIAN_POINT('Ctrl Pts',(13.335263436409,639.968754189557,55.9630634399455));
#104271=CARTESIAN_POINT('Ctrl Pts',(13.3695604686926,639.776280855815,56.0182814407224));
#104272=CARTESIAN_POINT('Ctrl Pts',(13.9047588183327,640.533044717664,57.36769888129));
#104273=CARTESIAN_POINT('Ctrl Pts',(14.1102991866389,640.509684718848,57.296294905319));
#104274=CARTESIAN_POINT('Ctrl Pts',(14.1299035774209,640.29672728974,57.3393334951756));
#104275=CARTESIAN_POINT('Ctrl Pts',(14.3247076934248,640.838404048473,58.3002140367118));
#104276=CARTESIAN_POINT('Ctrl Pts',(14.5388220217874,640.818919962782,58.233681282548));
#104277=CARTESIAN_POINT('Ctrl Pts',(14.5566498549489,640.598461612561,58.2756573376281));
#104278=CARTESIAN_POINT('Ctrl Pts',(14.7401433929705,641.144014898982,59.5471387316695));
#104279=CARTESIAN_POINT('Ctrl Pts',(14.9637997646997,641.128994182546,59.4803694808451));
#104280=CARTESIAN_POINT('Ctrl Pts',(14.9788110762547,640.900445339403,59.5276607666015));
#104281=CARTESIAN_POINT('Ctrl Pts',(14.8176813623333,641.201300483029,59.8008321998988));
#104282=CARTESIAN_POINT('Ctrl Pts',(15.0439529783747,641.187731406209,59.7367889937231));
#104283=CARTESIAN_POINT('Ctrl Pts',(15.0576058396701,640.957052162534,59.7823928247067));
#104284=CARTESIAN_POINT('Ctrl Pts',(14.9592279732976,641.306193352759,60.3093954217731));
#104285=CARTESIAN_POINT('Ctrl Pts',(15.1905205855739,641.295464675235,60.2513664040229));
#104286=CARTESIAN_POINT('Ctrl Pts',(15.2014471033479,641.060702480953,60.2930389236187));
#104287=CARTESIAN_POINT('Ctrl Pts',(15.0235498579237,641.354030625955,60.5651452400211));
#104288=CARTESIAN_POINT('Ctrl Pts',(15.2571084270983,641.344588327562,60.5101927719222));
#104289=CARTESIAN_POINT('Ctrl Pts',(15.2668116417703,641.107973039748,60.5498362104747));
#104290=CARTESIAN_POINT('Ctrl Pts',(15.1972467822455,641.483514247277,61.3368028828921));
#104291=CARTESIAN_POINT('Ctrl Pts',(15.4377062255518,641.478133269179,61.2940470335773));
#104292=CARTESIAN_POINT('Ctrl Pts',(15.4433255182961,641.23592371238,61.3246595339165));
#104293=CARTESIAN_POINT('Ctrl Pts',(15.2874077780666,641.551156104484,61.8571195614639));
#104294=CARTESIAN_POINT('Ctrl Pts',(15.5309261439817,641.547515205012,61.8206844364525));
#104295=CARTESIAN_POINT('Ctrl Pts',(15.5349475887123,641.302764009413,61.8471069255291));
#104296=CARTESIAN_POINT('Ctrl Pts',(15.4156790030771,641.647548755422,62.9097786108428));
#104297=CARTESIAN_POINT('Ctrl Pts',(15.6642372322958,641.646898393203,62.8892513959473));
#104298=CARTESIAN_POINT('Ctrl Pts',(15.6652986681034,641.398015292898,62.9040820559312));
#104299=CARTESIAN_POINT('Ctrl Pts',(15.4537982322333,641.67630751549,63.4421236247392));
#104300=CARTESIAN_POINT('Ctrl Pts',(15.7037030786927,641.676438218184,63.4286901969925));
#104301=CARTESIAN_POINT('Ctrl Pts',(15.7040356606937,641.426433309297,63.4386078350693));
#104302=CARTESIAN_POINT('Ctrl Pts',(15.4700545523021,641.68856386249,64.2501300119848));
#104303=CARTESIAN_POINT('Ctrl Pts',(15.720610340671,641.689084457603,64.2494068634906));
#104304=CARTESIAN_POINT('Ctrl Pts',(15.720555575138,641.438544541415,64.2499277579685));
#104305=CARTESIAN_POINT('Ctrl Pts',(15.4685832963044,641.687454020083,64.5221427161502));
#104306=CARTESIAN_POINT('Ctrl Pts',(15.7190815934227,641.687940364418,64.5256053426526));
#104307=CARTESIAN_POINT('Ctrl Pts',(15.7190604657519,641.437447841463,64.5230557734976));
#104308=CARTESIAN_POINT('Ctrl Pts',(15.4517606369933,641.67477231473,65.0625984317746));
#104309=CARTESIAN_POINT('Ctrl Pts',(15.7015814327667,641.674852353065,65.0746869533344));
#104310=CARTESIAN_POINT('Ctrl Pts',(15.7019650213429,641.424916281739,65.0657280699177));
#104311=CARTESIAN_POINT('Ctrl Pts',(15.4364817742608,641.663255235677,65.3311812375999));
#104312=CARTESIAN_POINT('Ctrl Pts',(15.685708149129,641.662981907014,65.3473542470335));
#104313=CARTESIAN_POINT('Ctrl Pts',(15.6864384446807,641.413535586959,65.3354120618728));
#104314=CARTESIAN_POINT('Ctrl Pts',(15.3266757045973,641.580587358346,66.6661082158761));
#104315=CARTESIAN_POINT('Ctrl Pts',(15.5718851336501,641.577969541552,66.6988378773207));
#104316=CARTESIAN_POINT('Ctrl Pts',(15.574852527381,641.331846983568,66.675805476863));
#104317=CARTESIAN_POINT('Ctrl Pts',(15.1329768512553,641.434622754534,67.7086964322208));
#104318=CARTESIAN_POINT('Ctrl Pts',(15.3741355634771,641.430085435439,67.7474289072551));
#104319=CARTESIAN_POINT('Ctrl Pts',(15.3780196332794,641.18761548309,67.7226505757277));
#104320=CARTESIAN_POINT('Ctrl Pts',(14.5395600793765,640.995589078133,69.7454059551597));
#104321=CARTESIAN_POINT('Ctrl Pts',(14.7598045961286,640.979270094842,69.8078650818198));
#104322=CARTESIAN_POINT('Ctrl Pts',(14.7749830115725,640.753782796594,69.7677006850111));
#104323=CARTESIAN_POINT('Ctrl Pts',(14.1502976929651,640.710325139517,70.7036228750289));
#104324=CARTESIAN_POINT('Ctrl Pts',(14.3625245593818,640.690337599714,70.7712664447536));
#104325=CARTESIAN_POINT('Ctrl Pts',(14.3794203054433,640.471905369692,70.7298312303411));
#104326=CARTESIAN_POINT('Ctrl Pts',(13.4435515701974,640.207670726134,72.0586962144293));
#104327=CARTESIAN_POINT('Ctrl Pts',(13.6295943491114,640.173459148157,72.1457661580742));
#104328=CARTESIAN_POINT('Ctrl Pts',(13.6612091794102,639.975202281057,72.0904647072316));
#104329=CARTESIAN_POINT('Ctrl Pts',(13.185856425802,640.026580539771,72.4987899104209));
#104330=CARTESIAN_POINT('Ctrl Pts',(13.3656347598372,639.989501793385,72.5875774487109));
#104331=CARTESIAN_POINT('Ctrl Pts',(13.3993396267296,639.796260366034,72.5323553744969));
#104332=CARTESIAN_POINT('Ctrl Pts',(12.6358638843126,639.647007028405,73.342434424191));
#104333=CARTESIAN_POINT('Ctrl Pts',(12.8021776094238,639.603984080128,73.4333645836815));
#104334=CARTESIAN_POINT('Ctrl Pts',(12.8404364611288,639.421189580259,73.3794426010547));
#104335=CARTESIAN_POINT('Ctrl Pts',(12.3442395607504,639.448958868854,73.745486468069));
#104336=CARTESIAN_POINT('Ctrl Pts',(12.5042121997375,639.403324003737,73.8371312504688));
#104337=CARTESIAN_POINT('Ctrl Pts',(12.5440885772941,639.225491647343,73.7841389135551));
#104338=CARTESIAN_POINT('Ctrl Pts',(11.7288256021103,639.040370142431,74.5171827762023));
#104339=CARTESIAN_POINT('Ctrl Pts',(11.875674081091,638.989684606096,74.6087740523791));
#104340=CARTESIAN_POINT('Ctrl Pts',(11.9187059559954,638.821752085494,74.5589805782249));
#104341=CARTESIAN_POINT('Ctrl Pts',(11.405033028947,638.829813906688,74.8858160421478));
#104342=CARTESIAN_POINT('Ctrl Pts',(11.5456832679028,638.776912022865,74.9772519297627));
#104343=CARTESIAN_POINT('Ctrl Pts',(11.5896694934917,638.613695450973,74.929116152772));
#104344=CARTESIAN_POINT('Ctrl Pts',(10.7249053554299,638.400136864158,75.5904935058696));
#104345=CARTESIAN_POINT('Ctrl Pts',(10.8529135843585,638.3431579851,75.6803058137442));
#104346=CARTESIAN_POINT('Ctrl Pts',(10.8985267731535,638.189120059749,75.6366626093528));
#104347=CARTESIAN_POINT('Ctrl Pts',(10.3672411512523,638.180215772508,75.9276498830203));
#104348=CARTESIAN_POINT('Ctrl Pts',(10.4891833026195,638.121410763412,76.0167162365072));
#104349=CARTESIAN_POINT('Ctrl Pts',(10.5350707806408,637.971810624902,75.9751917541415));
#104350=CARTESIAN_POINT('Ctrl Pts',(9.25217348404458,637.519731600676,76.8832498458298));
#104351=CARTESIAN_POINT('Ctrl Pts',(9.36501835682016,637.461581119493,76.9607377506827));
#104352=CARTESIAN_POINT('Ctrl Pts',(9.40196706845938,637.319183392587,76.9346610568732));
#104353=CARTESIAN_POINT('Ctrl Pts',(8.46041324950306,637.081923907435,77.4415886133237));
#104354=CARTESIAN_POINT('Ctrl Pts',(8.56117701294616,637.020060912213,77.5194907589741));
#104355=CARTESIAN_POINT('Ctrl Pts',(8.59738601729796,636.886574518512,77.495276682365));
#104356=CARTESIAN_POINT('Ctrl Pts',(7.18898333288859,636.462030730398,78.1691179476835));
#104357=CARTESIAN_POINT('Ctrl Pts',(7.26509469234156,636.394030650501,78.2466972418932));
#104358=CARTESIAN_POINT('Ctrl Pts',(7.30535316787382,636.274040082039,78.2257709379294));
#104359=CARTESIAN_POINT('Ctrl Pts',(6.75104020321683,636.261633925678,78.3931160864462));
#104360=CARTESIAN_POINT('Ctrl Pts',(6.82166576422308,636.192852698254,78.4694208274702));
#104361=CARTESIAN_POINT('Ctrl Pts',(6.86031993687873,636.076024891079,78.4506791819244));
#104362=CARTESIAN_POINT('Ctrl Pts',(5.84247174669281,635.881018125929,78.8029438408063));
#104363=CARTESIAN_POINT('Ctrl Pts',(5.902618394964,635.811465969196,78.8760152018326));
#104364=CARTESIAN_POINT('Ctrl Pts',(5.93704365902223,635.699934177541,78.8621698493515));
#104365=CARTESIAN_POINT('Ctrl Pts',(5.36938928293472,635.700106636653,78.9894068856547));
#104366=CARTESIAN_POINT('Ctrl Pts',(5.42397848879053,635.629978355184,79.0613189453554));
#104367=CARTESIAN_POINT('Ctrl Pts',(5.45630243005711,635.521173033899,79.0493901878842));
#104368=CARTESIAN_POINT('Ctrl Pts',(3.52314404173299,635.078196936271,79.6117444884673));
#104369=CARTESIAN_POINT('Ctrl Pts',(3.57309729308637,635.012413171809,79.6733677987882));
#104370=CARTESIAN_POINT('Ctrl Pts',(3.58020877289446,634.90667060112,79.6742394975195));
#104371=CARTESIAN_POINT('Ctrl Pts',(2.0770701544568,634.760124060554,79.8888901784769));
#104372=CARTESIAN_POINT('Ctrl Pts',(2.10064307445653,634.687981505965,79.9545722316598));
#104373=CARTESIAN_POINT('Ctrl Pts',(2.11068986848203,634.592364494609,79.9525257971374));
#104374=CARTESIAN_POINT('Ctrl Pts',(0.512173773971106,634.699225564137,
79.9473100410624));
#104375=CARTESIAN_POINT('Ctrl Pts',(0.516051947899616,634.628452832944,
80.0106401135641));
#104376=CARTESIAN_POINT('Ctrl Pts',(0.520472179553334,634.532196202332,
80.0111755920238));
#104377=CARTESIAN_POINT('Ctrl Pts',(3.90492814027074,633.321803177584,49.5221152197639));
#104378=CARTESIAN_POINT('Ctrl Pts',(4.14330398493611,632.870375197478,49.135784443326));
#104379=CARTESIAN_POINT('Ctrl Pts',(3.96801791400367,633.484430412185,49.0902664690196));
#104380=CARTESIAN_POINT('Ctrl Pts',(2.89083941488624,633.016561541034,49.2609200704197));
#104381=CARTESIAN_POINT('Ctrl Pts',(3.03742703509678,632.497931245809,48.8340694352976));
#104382=CARTESIAN_POINT('Ctrl Pts',(2.93755241694889,633.17526999398,48.8214432993564));
#104383=CARTESIAN_POINT('Ctrl Pts',(1.83964868594593,632.808625463471,49.0977046826038));
#104384=CARTESIAN_POINT('Ctrl Pts',(1.96126338863992,632.261216236514,48.6607567236519));
#104385=CARTESIAN_POINT('Ctrl Pts',(1.86937071959366,632.964660360168,48.6534581338935));
#104386=CARTESIAN_POINT('Ctrl Pts',(0.211280116816066,632.709872623992,
49.0195828117931));
#104387=CARTESIAN_POINT('Ctrl Pts',(0.224160992892843,632.141263789567,
48.5717336255604));
#104388=CARTESIAN_POINT('Ctrl Pts',(0.214693779414581,632.864638970137,
48.5730542692393));
#104389=CARTESIAN_POINT('Ctrl Pts',(-0.32245537920764,632.712766771114,
49.0218495189568));
#104390=CARTESIAN_POINT('Ctrl Pts',(-0.343446449653068,632.144773325884,
48.574308500153));
#104391=CARTESIAN_POINT('Ctrl Pts',(-0.327665155014434,632.867570296855,
48.5753871894563));
#104392=CARTESIAN_POINT('Ctrl Pts',(-1.37915307127922,632.785351839707,
49.0793205445456));
#104393=CARTESIAN_POINT('Ctrl Pts',(-1.47715237700549,632.233425912244,
48.6401671207799));
#104394=CARTESIAN_POINT('Ctrl Pts',(-1.40143442624709,632.941087722613,
48.6345369452367));
#104395=CARTESIAN_POINT('Ctrl Pts',(-1.90211842335103,632.855006180268,
49.1345303092449));
#104396=CARTESIAN_POINT('Ctrl Pts',(-2.02961823976853,632.316499577614,
48.701927360293));
#104397=CARTESIAN_POINT('Ctrl Pts',(-1.93284944505609,633.01163696098,48.6913595421491));
#104398=CARTESIAN_POINT('Ctrl Pts',(-2.93807698482498,633.054034036731,
49.2965498576802));
#104399=CARTESIAN_POINT('Ctrl Pts',(-3.12573547424563,632.554675921558,
48.8844736999008));
#104400=CARTESIAN_POINT('Ctrl Pts',(-2.98554566101708,633.213221513822,
48.858111903559));
#104401=CARTESIAN_POINT('Ctrl Pts',(-3.45374791090643,633.184501638302,
49.4043809868049));
#104402=CARTESIAN_POINT('Ctrl Pts',(-3.66252614078188,632.706685205911,
49.002867092975));
#104403=CARTESIAN_POINT('Ctrl Pts',(-3.50954896370792,633.345365412611,
48.969093235558));
#104404=CARTESIAN_POINT('Ctrl Pts',(-4.4468510663278,633.486560814703,49.6633692434331));
#104405=CARTESIAN_POINT('Ctrl Pts',(-4.69335204058051,633.057479661184,
49.2876872236508));
#104406=CARTESIAN_POINT('Ctrl Pts',(-4.51869902314396,633.651305216357,
49.2356474341197));
#104407=CARTESIAN_POINT('Ctrl Pts',(-4.92792605251174,633.658498481233,
49.8148076425706));
#104408=CARTESIAN_POINT('Ctrl Pts',(-5.18656612683332,633.252577971486,
49.4506178691368));
#104409=CARTESIAN_POINT('Ctrl Pts',(-5.00754801428307,633.825452135949,
49.3915102529955));
#104410=CARTESIAN_POINT('Ctrl Pts',(-5.86442374504572,634.032530746289,
50.1589844638927));
#104411=CARTESIAN_POINT('Ctrl Pts',(-6.14248615971892,633.674547007798,
49.8207309756671));
#104412=CARTESIAN_POINT('Ctrl Pts',(-5.95917956692151,634.204290165079,
49.7457424205663));
#104413=CARTESIAN_POINT('Ctrl Pts',(-6.32024772390201,634.234853771403,
50.351944968455));
#104414=CARTESIAN_POINT('Ctrl Pts',(-6.60402168968756,633.898761420426,
50.024761085077));
#104415=CARTESIAN_POINT('Ctrl Pts',(-6.4223701414918,634.409213025463,49.9443408012826));
#104416=CARTESIAN_POINT('Ctrl Pts',(-7.20798452548951,634.659869888413,
50.7781230179888));
#104417=CARTESIAN_POINT('Ctrl Pts',(-7.49937336947295,634.367016492284,
50.4751585816832));
#104418=CARTESIAN_POINT('Ctrl Pts',(-7.32445419098542,634.839690427277,
50.382970765863));
#104419=CARTESIAN_POINT('Ctrl Pts',(-7.63444059270741,634.879877998268,
51.0086543329385));
#104420=CARTESIAN_POINT('Ctrl Pts',(-7.92808282222852,634.606627980339,
50.7161247240279));
#104421=CARTESIAN_POINT('Ctrl Pts',(-7.75780268783223,635.062525716147,
50.6202380193044));
#104422=CARTESIAN_POINT('Ctrl Pts',(-8.86930646895302,635.551146061136,
51.7511985187908));
#104423=CARTESIAN_POINT('Ctrl Pts',(-9.13407034427917,635.315485808938,
51.4724609662051));
#104424=CARTESIAN_POINT('Ctrl Pts',(-9.01263265026787,635.742422596475,
51.3844819472612));
#104425=CARTESIAN_POINT('Ctrl Pts',(-9.63391884695173,636.013257995688,
52.3135263786952));
#104426=CARTESIAN_POINT('Ctrl Pts',(-9.90255020916195,635.809844851862,
52.0496752501994));
#104427=CARTESIAN_POINT('Ctrl Pts',(-9.78960325654475,636.21047313013,51.9632424341007));
#104428=CARTESIAN_POINT('Ctrl Pts',(-10.705439897833,636.697610172111,53.2657428837752));
#104429=CARTESIAN_POINT('Ctrl Pts',(-10.9910069155268,636.550097791243,
53.0515055379338));
#104430=CARTESIAN_POINT('Ctrl Pts',(-10.878441060838,636.903617518938,52.9432807545543));
#104431=CARTESIAN_POINT('Ctrl Pts',(-11.0508876799252,636.925101298073,
53.6025635511897));
#104432=CARTESIAN_POINT('Ctrl Pts',(-11.3347418937743,636.79016171467,53.3968965258403));
#104433=CARTESIAN_POINT('Ctrl Pts',(-11.229472953103,637.134032223376,53.2899442539113));
#104434=CARTESIAN_POINT('Ctrl Pts',(-11.7115273981156,637.370048161634,
54.31121164042));
#104435=CARTESIAN_POINT('Ctrl Pts',(-11.9901371105211,637.257589819536,
54.1232083059766));
#104436=CARTESIAN_POINT('Ctrl Pts',(-11.900792348141,637.58469745544,54.0193011734408));
#104437=CARTESIAN_POINT('Ctrl Pts',(-12.0239781544445,637.585612042381,
54.679895712359));
#104438=CARTESIAN_POINT('Ctrl Pts',(-12.3010560005085,637.484007381368,
54.5005517772709));
#104439=CARTESIAN_POINT('Ctrl Pts',(-12.218293964521,637.803031627762,54.3987594591597));
#104440=CARTESIAN_POINT('Ctrl Pts',(-12.9089989609887,638.206484722157,
55.8305641478284));
#104441=CARTESIAN_POINT('Ctrl Pts',(-13.1641372034306,638.122333337238,
55.657554710526));
#104442=CARTESIAN_POINT('Ctrl Pts',(-13.1176253793484,638.431885953125,
55.5830589493271));
#104443=CARTESIAN_POINT('Ctrl Pts',(-13.4299816943561,638.586242973041,
56.6565755853746));
#104444=CARTESIAN_POINT('Ctrl Pts',(-13.6882441199943,638.522792922679,
56.502781818501));
#104445=CARTESIAN_POINT('Ctrl Pts',(-13.6470291437565,638.81652388569,56.4332097702866));
#104446=CARTESIAN_POINT('Ctrl Pts',(-13.9880869203314,639.000081291731,
57.7753259736852));
#104447=CARTESIAN_POINT('Ctrl Pts',(-14.2513227291178,638.960240306637,
57.6633206048862));
#104448=CARTESIAN_POINT('Ctrl Pts',(-14.2141551453113,639.235679320329,
57.5846512128922));
#104449=CARTESIAN_POINT('Ctrl Pts',(-14.0949913651594,639.079785918328,
58.0034349097068));
#104450=CARTESIAN_POINT('Ctrl Pts',(-14.3573300164066,639.042991451251,
57.895659279968));
#104451=CARTESIAN_POINT('Ctrl Pts',(-14.3227879338756,639.316408326257,
57.8194266921124));
#104452=CARTESIAN_POINT('Ctrl Pts',(-14.2989297883243,639.23250072315,58.4689050674605));
#104453=CARTESIAN_POINT('Ctrl Pts',(-14.5593558255444,639.201314374317,
58.3695243760315));
#104454=CARTESIAN_POINT('Ctrl Pts',(-14.5300235323771,639.471085886935,
58.298500421927));
#104455=CARTESIAN_POINT('Ctrl Pts',(-14.3962813329383,639.305751532961,
58.707145038779));
#104456=CARTESIAN_POINT('Ctrl Pts',(-14.655901579792,639.277294876988,58.6120969468063));
#104457=CARTESIAN_POINT('Ctrl Pts',(-14.628948992512,639.545278131669,58.5437030695108));
#104458=CARTESIAN_POINT('Ctrl Pts',(-14.6697948864641,639.512315164104,
59.4288869888394));
#104459=CARTESIAN_POINT('Ctrl Pts',(-14.9255658148712,639.490221334045,
59.3430538394069));
#104460=CARTESIAN_POINT('Ctrl Pts',(-14.9068849327433,639.754496848634,
59.2865392357633));
#104461=CARTESIAN_POINT('Ctrl Pts',(-14.8276358084694,639.632573093502,
59.919163080231));
#104462=CARTESIAN_POINT('Ctrl Pts',(-15.0827345831201,639.615278031787,
59.8429002079945));
#104463=CARTESIAN_POINT('Ctrl Pts',(-15.0672776140326,639.876300254906,
59.7911438168927));
#104464=CARTESIAN_POINT('Ctrl Pts',(-15.0935663577189,639.836054760192,
60.9185223424128));
#104465=CARTESIAN_POINT('Ctrl Pts',(-15.3461975432606,639.825729960273,
60.8592543910126));
#104466=CARTESIAN_POINT('Ctrl Pts',(-15.3375077166812,640.082397178936,
60.8197103861867));
#104467=CARTESIAN_POINT('Ctrl Pts',(-15.2016635310883,639.919288867215,
61.427601771592));
#104468=CARTESIAN_POINT('Ctrl Pts',(-15.4538492122169,639.91219607755,61.3780952510847));
#104469=CARTESIAN_POINT('Ctrl Pts',(-15.4473524788766,640.166700956264,
61.3436679646832));
#104470=CARTESIAN_POINT('Ctrl Pts',(-15.3656085202112,640.045795416604,
62.4657118072439));
#104471=CARTESIAN_POINT('Ctrl Pts',(-15.6162781423566,640.042912732702,
62.4334323880538));
#104472=CARTESIAN_POINT('Ctrl Pts',(-15.6139481543257,640.29483344227,62.4121180900535));
#104473=CARTESIAN_POINT('Ctrl Pts',(-15.4213599206253,640.088993672632,
62.9982308158159));
#104474=CARTESIAN_POINT('Ctrl Pts',(-15.6718168191366,640.087770818522,
62.9761672199096));
#104475=CARTESIAN_POINT('Ctrl Pts',(-15.6706008816092,640.338586851437,
62.9602003371774));
#104476=CARTESIAN_POINT('Ctrl Pts',(-15.5027019825929,640.152021343924,
64.5826472633091));
#104477=CARTESIAN_POINT('Ctrl Pts',(-15.7522976417821,640.152776608118,
64.5843508815025));
#104478=CARTESIAN_POINT('Ctrl Pts',(-15.7532581285021,640.40242461464,64.5909241146122));
#104479=CARTESIAN_POINT('Ctrl Pts',(-15.4463343132364,640.108075542961,
65.6318366328334));
#104480=CARTESIAN_POINT('Ctrl Pts',(-15.6952083223957,640.10642266285,65.6625224224092));
#104481=CARTESIAN_POINT('Ctrl Pts',(-15.6959793937825,640.357914230718,
65.6707746519288));
#104482=CARTESIAN_POINT('Ctrl Pts',(-15.2386509518819,639.947832781043,
66.9345709030678));
#104483=CARTESIAN_POINT('Ctrl Pts',(-15.4907481596751,639.941893637217,
66.9784967286438));
#104484=CARTESIAN_POINT('Ctrl Pts',(-15.4849378554675,640.195611685116,
67.011585045083));
#104485=CARTESIAN_POINT('Ctrl Pts',(-15.1900189384783,639.910359834832,
67.1952431231479));
#104486=CARTESIAN_POINT('Ctrl Pts',(-15.442502106951,639.903116285289,67.2436796227911));
#104487=CARTESIAN_POINT('Ctrl Pts',(-15.4355195703926,640.15765712674,67.2798756894921));
#104488=CARTESIAN_POINT('Ctrl Pts',(-15.0803219964504,639.826036123596,
67.7086233424261));
#104489=CARTESIAN_POINT('Ctrl Pts',(-15.3338238879868,639.81595115727,67.7656619175894));
#104490=CARTESIAN_POINT('Ctrl Pts',(-15.3240490417368,640.072249639251,
67.8082600435595));
#104491=CARTESIAN_POINT('Ctrl Pts',(-15.0191594320567,639.779109751635,
67.9621453552883));
#104492=CARTESIAN_POINT('Ctrl Pts',(-15.2731532452162,639.767372623407,
68.0236001703991));
#104493=CARTESIAN_POINT('Ctrl Pts',(-15.2618976191312,640.024720157075,
68.0691914822997));
#104494=CARTESIAN_POINT('Ctrl Pts',(-14.8174033801442,639.624768231545,
68.7135999647743));
#104495=CARTESIAN_POINT('Ctrl Pts',(-15.0725761726714,639.607186299064,
68.7904931957739));
#104496=CARTESIAN_POINT('Ctrl Pts',(-15.0568797539538,639.86839508466,68.8426074874175));
#104497=CARTESIAN_POINT('Ctrl Pts',(-14.6585957360926,639.50381566693,69.202444416695));
#104498=CARTESIAN_POINT('Ctrl Pts',(-14.9144766233915,639.481427523697,
69.2887981194115));
#104499=CARTESIAN_POINT('Ctrl Pts',(-14.8955047156438,639.745888110387,
69.3457386057789));
#104500=CARTESIAN_POINT('Ctrl Pts',(-14.2945157770192,639.228940094288,
70.1573336769515));
#104501=CARTESIAN_POINT('Ctrl Pts',(-14.55378196445,639.196702300566,70.2605787665661));
#104502=CARTESIAN_POINT('Ctrl Pts',(-14.5255384316863,639.467479706879,
70.3285351375797));
#104503=CARTESIAN_POINT('Ctrl Pts',(-14.0881807313278,639.074224407355,
70.6254072326268));
#104504=CARTESIAN_POINT('Ctrl Pts',(-14.3484256804248,639.035608179291,
70.7379242119137));
#104505=CARTESIAN_POINT('Ctrl Pts',(-14.3158676780004,639.310775702103,
70.8102881691105));
#104506=CARTESIAN_POINT('Ctrl Pts',(-13.6346129612246,638.738060594009,
71.5295833283864));
#104507=CARTESIAN_POINT('Ctrl Pts',(-13.8990584488247,638.686648055336,
71.6590019112753));
#104508=CARTESIAN_POINT('Ctrl Pts',(-13.8549669417811,638.970291387194,
71.740888971284));
#104509=CARTESIAN_POINT('Ctrl Pts',(-13.3887414345827,638.557610315938,
71.9636076884644));
#104510=CARTESIAN_POINT('Ctrl Pts',(-13.6545221187428,638.498448696131,
72.1017559982509));
#104511=CARTESIAN_POINT('Ctrl Pts',(-13.6051205939733,638.787522044506,
72.1875975711325));
#104512=CARTESIAN_POINT('Ctrl Pts',(-12.8610969146662,638.176033974939,
72.7988987818575));
#104513=CARTESIAN_POINT('Ctrl Pts',(-13.1316816038927,638.101182146061,
72.9538576019717));
#104514=CARTESIAN_POINT('Ctrl Pts',(-13.0689457304277,638.401041596807,
73.0472996885173));
#104515=CARTESIAN_POINT('Ctrl Pts',(-12.5793162792295,637.974891871437,
73.2001530637705));
#104516=CARTESIAN_POINT('Ctrl Pts',(-12.851407762716,637.890759692315,73.3637342809632));
#104517=CARTESIAN_POINT('Ctrl Pts',(-12.7826098802753,638.197314518502,
73.4602802768307));
#104518=CARTESIAN_POINT('Ctrl Pts',(-11.9805147599271,637.55547313329,73.9719948691702));
#104519=CARTESIAN_POINT('Ctrl Pts',(-12.2578204673371,637.452363532576,
74.1526852709296));
#104520=CARTESIAN_POINT('Ctrl Pts',(-12.1741279655269,637.772505393729,
74.2546782628821));
#104521=CARTESIAN_POINT('Ctrl Pts',(-11.6620754094574,637.336246875743,
74.3439606423759));
#104522=CARTESIAN_POINT('Ctrl Pts',(-11.9410485726769,637.222125276071,
74.5332916257023));
#104523=CARTESIAN_POINT('Ctrl Pts',(-11.8505409335869,637.550461763023,
74.6375141662316));
#104524=CARTESIAN_POINT('Ctrl Pts',(-10.6667627124656,636.667502706153,
75.4012723114464));
#104525=CARTESIAN_POINT('Ctrl Pts',(-10.9336515194875,636.505188339921,
75.6390199582536));
#104526=CARTESIAN_POINT('Ctrl Pts',(-10.8391421878638,636.873125582928,
75.7257195228643));
#104527=CARTESIAN_POINT('Ctrl Pts',(-9.94964215326505,636.205767320931,
76.0314203061157));
#104528=CARTESIAN_POINT('Ctrl Pts',(-10.2135091666313,636.014005317852,
76.284404155343));
#104529=CARTESIAN_POINT('Ctrl Pts',(-10.1104306891926,636.405456574106,
76.3742823947935));
#104530=CARTESIAN_POINT('Ctrl Pts',(-8.39977812395367,635.286028861029,
77.1587292660183));
#104531=CARTESIAN_POINT('Ctrl Pts',(-8.66654368556743,635.029291056602,
77.453673623364));
#104532=CARTESIAN_POINT('Ctrl Pts',(-8.53551476998558,635.473898567317,
77.5345321156382));
#104533=CARTESIAN_POINT('Ctrl Pts',(-7.56052958968753,634.824608154755,
77.6580776200298));
#104534=CARTESIAN_POINT('Ctrl Pts',(-7.82150334606982,634.531572945309,
77.9681106439715));
#104535=CARTESIAN_POINT('Ctrl Pts',(-7.68270213057854,635.006547965821,
78.0484723196597));
#104536=CARTESIAN_POINT('Ctrl Pts',(-5.74312393564903,633.963249742456,
78.5165117385326));
#104537=CARTESIAN_POINT('Ctrl Pts',(-5.97772848586131,633.57629741229,78.8809740559797));
#104538=CARTESIAN_POINT('Ctrl Pts',(-5.83592524213799,634.134121869069,
78.9319873742495));
#104539=CARTESIAN_POINT('Ctrl Pts',(-4.75593424029188,633.563595057341,
78.8719595177936));
#104540=CARTESIAN_POINT('Ctrl Pts',(-4.97553001272719,633.135378140081,
79.2506052240653));
#104541=CARTESIAN_POINT('Ctrl Pts',(-4.83278432840491,633.729331434717,
79.2978208896897));
#104542=CARTESIAN_POINT('Ctrl Pts',(-3.68751695697931,633.257997703468,
79.1311980167567));
#104543=CARTESIAN_POINT('Ctrl Pts',(-3.91740045113657,632.79611528243,79.5230579121953));
#104544=CARTESIAN_POINT('Ctrl Pts',(-3.74709337805201,633.419805103089,
79.5646350435076));
#104545=CARTESIAN_POINT('Origin',(-48.,640.125373764374,64.2994740882088));
#104546=CARTESIAN_POINT('Ctrl Pts',(-2.24460771689896,634.860167926555,
52.2254855816307));
#104547=CARTESIAN_POINT('Ctrl Pts',(-2.07343281068578,635.935476877995,
52.1937144269263));
#104548=CARTESIAN_POINT('Ctrl Pts',(-2.33599035692052,635.234460352332,
51.4023619931513));
#104549=CARTESIAN_POINT('Ctrl Pts',(-1.83071110480402,634.789230599513,
52.1485430639701));
#104550=CARTESIAN_POINT('Ctrl Pts',(-1.68007361159745,635.884219683812,
52.1267455450006));
#104551=CARTESIAN_POINT('Ctrl Pts',(-1.90524322638816,635.161651519204,
51.3201743394719));
#104552=CARTESIAN_POINT('Ctrl Pts',(-1.41178093416776,634.736536724958,
52.0926096107395));
#104553=CARTESIAN_POINT('Ctrl Pts',(-1.29419848643582,635.848311670572,
52.0803434838513));
#104554=CARTESIAN_POINT('Ctrl Pts',(-1.46925731177574,635.107567404497,
51.2604278885429));
#104555=CARTESIAN_POINT('Ctrl Pts',(-0.57140262553684,634.672468556966,
52.0248171104673));
#104556=CARTESIAN_POINT('Ctrl Pts',(-0.520642208727863,635.80436668002,
52.0235847625471));
#104557=CARTESIAN_POINT('Ctrl Pts',(-0.594665493514755,635.041808942665,
51.1880140002959));
#104558=CARTESIAN_POINT('Ctrl Pts',(-0.147816545353252,634.660621292595,
52.0124327336182));
#104559=CARTESIAN_POINT('Ctrl Pts',(-0.136056956437475,635.796530340598,
52.0135137672583));
#104560=CARTESIAN_POINT('Ctrl Pts',(-0.153834462869262,635.029649119754,
51.1747853911568));
#104561=CARTESIAN_POINT('Ctrl Pts',(1.1024719364547,634.686646709549,52.0398201590788));
#104562=CARTESIAN_POINT('Ctrl Pts',(1.00747162781077,635.814178115524,52.0362579003524));
#104563=CARTESIAN_POINT('Ctrl Pts',(1.1473556856947,635.05636115653,51.2040398030431));
#104564=CARTESIAN_POINT('Ctrl Pts',(1.91894009807576,634.784664642294,52.1416799438264));
#104565=CARTESIAN_POINT('Ctrl Pts',(1.74120896424278,635.876480206933,52.1156863094179));
#104566=CARTESIAN_POINT('Ctrl Pts',(1.99706350164218,635.156964960755,51.3128431956377));
#104567=CARTESIAN_POINT('Ctrl Pts',(3.12055673201111,635.032654985143,52.414597409285));
#104568=CARTESIAN_POINT('Ctrl Pts',(2.89662070513935,636.059663351124,52.3569131035477));
#104569=CARTESIAN_POINT('Ctrl Pts',(3.24760126429163,635.411498116049,51.6043655628081));
#104570=CARTESIAN_POINT('Ctrl Pts',(3.51645511552271,635.132146568009,52.5259194378218));
#104571=CARTESIAN_POINT('Ctrl Pts',(3.27570850901759,636.133135826386,52.4544566039408));
#104572=CARTESIAN_POINT('Ctrl Pts',(3.65961769328675,635.513614580972,51.7232764264806));
#104573=CARTESIAN_POINT('Ctrl Pts',(4.28117411180073,635.353817098604,52.7819398834267));
#104574=CARTESIAN_POINT('Ctrl Pts',(4.01998858621208,636.303527595311,52.6857610821952));
#104575=CARTESIAN_POINT('Ctrl Pts',(4.45547060211493,635.741133515995,51.9967499482209));
#104576=CARTESIAN_POINT('Ctrl Pts',(4.6527703895603,635.476516292076,52.9272079191087));
#104577=CARTESIAN_POINT('Ctrl Pts',(4.38560256268007,636.399515892701,52.8180868283054));
#104578=CARTESIAN_POINT('Ctrl Pts',(4.84219570557192,635.867069920958,52.151921010376));
#104579=CARTESIAN_POINT('Ctrl Pts',(5.73871252059237,635.87149768931,53.412985235997));
#104580=CARTESIAN_POINT('Ctrl Pts',(5.44769236904264,636.712667166468,53.2632683827815));
#104581=CARTESIAN_POINT('Ctrl Pts',(5.97234965215429,636.27247217119,52.6708141112791));
#104582=CARTESIAN_POINT('Ctrl Pts',(6.42887593638936,636.172846954948,53.8068469880404));
#104583=CARTESIAN_POINT('Ctrl Pts',(6.15032378335572,636.963514950924,53.6342198283953));
#104584=CARTESIAN_POINT('Ctrl Pts',(6.69061225764372,636.581772120217,53.0915259083752));
#104585=CARTESIAN_POINT('Ctrl Pts',(7.70252122853822,636.789511859623,54.7027643205653));
#104586=CARTESIAN_POINT('Ctrl Pts',(7.45997458021479,637.499093628627,54.5105690457221));
#104587=CARTESIAN_POINT('Ctrl Pts',(8.01611292013624,637.214707153726,54.0485198842105));
#104588=CARTESIAN_POINT('Ctrl Pts',(8.29093833512778,637.106408722947,55.2059626243289));
#104589=CARTESIAN_POINT('Ctrl Pts',(8.07548401458602,637.781573825439,55.0065471941012));
#104590=CARTESIAN_POINT('Ctrl Pts',(8.62848726547417,637.539965112437,54.5860224232522));
#104591=CARTESIAN_POINT('Ctrl Pts',(9.10615860494565,637.572335029063,56.0502090602173));
#104592=CARTESIAN_POINT('Ctrl Pts',(8.93980322327443,638.210231222331,55.8666947129737));
#104593=CARTESIAN_POINT('Ctrl Pts',(9.47689944401278,638.018184818951,55.4878240797596));
#104594=CARTESIAN_POINT('Ctrl Pts',(9.36580248126735,637.725748496083,56.3462294979682));
#104595=CARTESIAN_POINT('Ctrl Pts',(9.21205942946594,638.350440979971,56.164626520581));
#104596=CARTESIAN_POINT('Ctrl Pts',(9.74711472218158,638.17564602195,55.8040251608737));
#104597=CARTESIAN_POINT('Ctrl Pts',(9.85277663850557,638.020454436639,56.9581425734282));
#104598=CARTESIAN_POINT('Ctrl Pts',(9.72214071534082,638.620905078637,56.782813652941));
#104599=CARTESIAN_POINT('Ctrl Pts',(10.2539160475817,638.478127626706,56.4576543706004));
#104600=CARTESIAN_POINT('Ctrl Pts',(10.0814069885408,638.162492524898,57.2753308908016));
#104601=CARTESIAN_POINT('Ctrl Pts',(9.96275939343532,638.752361475952,57.1043691500725));
#104602=CARTESIAN_POINT('Ctrl Pts',(10.4918551409475,638.62391333402,56.7964665120035));
#104603=CARTESIAN_POINT('Ctrl Pts',(10.7230189007579,638.568474894698,58.2619328657198));
#104604=CARTESIAN_POINT('Ctrl Pts',(10.6285633925527,639.124299658112,58.0946841395296));
#104605=CARTESIAN_POINT('Ctrl Pts',(11.1595901762937,639.040607207916,57.8503282493184));
#104606=CARTESIAN_POINT('Ctrl Pts',(11.0923717675951,638.812533808457,58.9658852559509));
#104607=CARTESIAN_POINT('Ctrl Pts',(11.0225929845114,639.355453995367,58.8154970554682));
#104608=CARTESIAN_POINT('Ctrl Pts',(11.543981587863,639.291105624835,58.6022718329819));
#104609=CARTESIAN_POINT('Ctrl Pts',(11.7014944118088,639.222460518805,60.4833358094967));
#104610=CARTESIAN_POINT('Ctrl Pts',(11.6644122825579,639.740850111134,60.3684103254258));
#104611=CARTESIAN_POINT('Ctrl Pts',(12.1779050110386,639.71184812148,60.223173033479));
#104612=CARTESIAN_POINT('Ctrl Pts',(11.9301672368271,639.380786781681,61.2707799874375));
#104613=CARTESIAN_POINT('Ctrl Pts',(11.9096549681383,639.892977017353,61.182086329466));
#104614=CARTESIAN_POINT('Ctrl Pts',(12.4158885617532,639.874351870955,61.0643007636695));
#104615=CARTESIAN_POINT('Ctrl Pts',(12.1537770914997,639.536320911666,62.4895659620246));
#104616=CARTESIAN_POINT('Ctrl Pts',(12.1464642268629,640.040786570914,62.4384492041064));
#104617=CARTESIAN_POINT('Ctrl Pts',(12.6486028978816,640.033989752196,62.3661767157842));
#104618=CARTESIAN_POINT('Ctrl Pts',(12.2085200304299,639.574645413003,62.9037553260946));
#104619=CARTESIAN_POINT('Ctrl Pts',(12.2044669680803,640.077264694283,62.864765245725));
#104620=CARTESIAN_POINT('Ctrl Pts',(12.7055747490575,640.073325442003,62.808603167802));
#104621=CARTESIAN_POINT('Ctrl Pts',(12.2753636450861,639.621482578138,63.7414063290601));
#104622=CARTESIAN_POINT('Ctrl Pts',(12.274978483213,640.121657485856,63.7252770410462));
#104623=CARTESIAN_POINT('Ctrl Pts',(12.7751399565671,640.121398393795,63.7033604237967));
#104624=CARTESIAN_POINT('Ctrl Pts',(12.2870666679087,639.629713325934,64.1583756132804));
#104625=CARTESIAN_POINT('Ctrl Pts',(12.2873846747713,640.129502073405,64.1547225574821));
#104626=CARTESIAN_POINT('Ctrl Pts',(12.787319479616,640.129846309535,64.148756333092));
#104627=CARTESIAN_POINT('Ctrl Pts',(12.268530884661,639.616704590037,64.9887244061268));
#104628=CARTESIAN_POINT('Ctrl Pts',(12.2678309313977,640.117168305939,65.0078610328854));
#104629=CARTESIAN_POINT('Ctrl Pts',(12.7680289967845,640.11649434121,65.0357135662794));
#104630=CARTESIAN_POINT('Ctrl Pts',(12.238288133047,639.595462971966,65.4021035317435));
#104631=CARTESIAN_POINT('Ctrl Pts',(12.235780004542,640.096933666824,65.4335305959216));
#104632=CARTESIAN_POINT('Ctrl Pts',(12.7365548811428,640.094692264775,65.4772745550034));
#104633=CARTESIAN_POINT('Ctrl Pts',(12.1360079708598,639.523971401827,66.2252982180572));
#104634=CARTESIAN_POINT('Ctrl Pts',(12.1278948320545,640.029206587871,66.2789946000502));
#104635=CARTESIAN_POINT('Ctrl Pts',(12.6301103000015,640.021314407659,66.3565899298897));
#104636=CARTESIAN_POINT('Ctrl Pts',(12.0634251058667,639.473341425651,66.6373579383003));
#104637=CARTESIAN_POINT('Ctrl Pts',(12.0509917691496,639.981048358942,66.7029848588286));
#104638=CARTESIAN_POINT('Ctrl Pts',(12.5545721539083,639.969348564671,66.7967415398965));
#104639=CARTESIAN_POINT('Ctrl Pts',(11.7851849710258,639.280776882324,67.8517603894219));
#104640=CARTESIAN_POINT('Ctrl Pts',(11.7560671806613,639.798044599605,67.9555151604994));
#104641=CARTESIAN_POINT('Ctrl Pts',(12.265003213869,639.771703221168,68.0939351245997));
#104642=CARTESIAN_POINT('Ctrl Pts',(11.5231511655743,639.100787569077,68.6226018819362));
#104643=CARTESIAN_POINT('Ctrl Pts',(11.4753688142236,639.625565690201,68.7506469944195));
#104644=CARTESIAN_POINT('Ctrl Pts',(11.9923003685254,639.586964845123,68.9173282151888));
#104645=CARTESIAN_POINT('Ctrl Pts',(11.0237873908383,638.768313052576,69.7270719203858));
#104646=CARTESIAN_POINT('Ctrl Pts',(10.9544028777391,639.316649953524,69.8689551387737));
#104647=CARTESIAN_POINT('Ctrl Pts',(11.4726049050073,639.245718209948,70.0970939152249));
#104648=CARTESIAN_POINT('Ctrl Pts',(10.8384310991565,638.646368112428,70.0880515743831));
#104649=CARTESIAN_POINT('Ctrl Pts',(10.7586359325232,639.202227930314,70.237687260735));
#104650=CARTESIAN_POINT('Ctrl Pts',(11.2797017252308,639.120555783983,70.4826829420179));
#104651=CARTESIAN_POINT('Ctrl Pts',(10.4390987804155,638.388472497937,70.7805569003536));
#104652=CARTESIAN_POINT('Ctrl Pts',(10.3387444088613,638.961980514628,70.9429750385828));
#104653=CARTESIAN_POINT('Ctrl Pts',(10.8641104504998,638.855855695182,71.2223989202368));
#104654=CARTESIAN_POINT('Ctrl Pts',(10.2247929217345,638.252281349441,71.1132662015513));
#104655=CARTESIAN_POINT('Ctrl Pts',(10.1129153329541,638.835266089697,71.2812239398438));
#104656=CARTESIAN_POINT('Ctrl Pts',(10.6410790491553,638.716071190731,71.5777902117513));
#104657=CARTESIAN_POINT('Ctrl Pts',(9.76784625223806,637.968524861273,71.7535556942923));
#104658=CARTESIAN_POINT('Ctrl Pts',(9.63349659380944,638.573272816231,71.9302320108111));
#104659=CARTESIAN_POINT('Ctrl Pts',(10.1655277254286,638.424827920137,72.261730451579));
#104660=CARTESIAN_POINT('Ctrl Pts',(9.5252037421373,637.820949216077,72.0611303923611));
#104661=CARTESIAN_POINT('Ctrl Pts',(9.37852363969348,638.437416201048,72.2410837179652));
#104662=CARTESIAN_POINT('Ctrl Pts',(9.91300599012881,638.273358557248,72.5902735372759));
#104663=CARTESIAN_POINT('Ctrl Pts',(9.01135722475072,637.517417174847,72.6522134952531));
#104664=CARTESIAN_POINT('Ctrl Pts',(8.84120033390604,638.160459112116,72.836293304798));
#104665=CARTESIAN_POINT('Ctrl Pts',(9.37823825283678,637.961817993545,73.2216526442934));
#104666=CARTESIAN_POINT('Ctrl Pts',(8.73891002500459,637.360785169889,72.9367840692432));
#104667=CARTESIAN_POINT('Ctrl Pts',(8.55620892724539,638.018341471135,73.1214587846384));
#104668=CARTESIAN_POINT('Ctrl Pts',(9.09469840048593,637.801053343874,73.5256232407945));
#104669=CARTESIAN_POINT('Ctrl Pts',(7.89012810647255,636.890473661098,73.7426824430362));
#104670=CARTESIAN_POINT('Ctrl Pts',(7.65796125292149,637.588671243196,73.939427215562));
#104671=CARTESIAN_POINT('Ctrl Pts',(8.21135820442717,637.318332755003,74.3864623908746));
#104672=CARTESIAN_POINT('Ctrl Pts',(7.28116846417886,636.574939347645,74.219742003199));
#104673=CARTESIAN_POINT('Ctrl Pts',(7.02391120497905,637.310866383018,74.4058463661051));
#104674=CARTESIAN_POINT('Ctrl Pts',(7.57760505325563,636.99447333735,74.8960441316923));
#104675=CARTESIAN_POINT('Ctrl Pts',(6.2965924934778,636.122015748582,74.8505072253373));
#104676=CARTESIAN_POINT('Ctrl Pts',(6.03600513843958,636.930051586802,75.0061312303154));
#104677=CARTESIAN_POINT('Ctrl Pts',(6.55294358412831,636.529600037755,75.5698095385058));
#104678=CARTESIAN_POINT('Ctrl Pts',(5.95642441709212,635.974486587073,75.0464903317535));
#104679=CARTESIAN_POINT('Ctrl Pts',(5.69039769264687,636.806083719561,75.193320382361));
#104680=CARTESIAN_POINT('Ctrl Pts',(6.19892597176367,636.378178494287,75.7791531330914));
#104681=CARTESIAN_POINT('Ctrl Pts',(5.24924375098351,635.691366240682,75.4090550759564));
#104682=CARTESIAN_POINT('Ctrl Pts',(4.97872636614066,636.572134933507,75.5368081438878));
#104683=CARTESIAN_POINT('Ctrl Pts',(5.46295346090092,636.087588372664,76.166434449957));
#104684=CARTESIAN_POINT('Ctrl Pts',(4.88532837447766,635.557125517645,75.5738955184618));
#104685=CARTESIAN_POINT('Ctrl Pts',(4.61623378897083,636.464208081758,75.6897044857469));
#104686=CARTESIAN_POINT('Ctrl Pts',(5.084221879631,635.9498059108,76.3425122362357));
#104687=CARTESIAN_POINT('Ctrl Pts',(3.7708907749372,635.18796386149,76.0143384748105));
#104688=CARTESIAN_POINT('Ctrl Pts',(3.4968238391205,636.167052993904,76.1025288496455));
#104689=CARTESIAN_POINT('Ctrl Pts',(3.92441156002437,635.570904328349,76.812980796566));
#104690=CARTESIAN_POINT('Ctrl Pts',(2.99381238346123,634.984436447013,76.238938541679));
#104691=CARTESIAN_POINT('Ctrl Pts',(2.75796680224509,636.02168241599,76.2927147804116));
#104692=CARTESIAN_POINT('Ctrl Pts',(3.11569968988111,635.362007903861,77.0528911109046));
#104693=CARTESIAN_POINT('Ctrl Pts',(2.17374385871217,634.848209408432,76.3864215127495));
#104694=CARTESIAN_POINT('Ctrl Pts',(2.00694303543428,635.926951046402,76.4163679119409));
#104695=CARTESIAN_POINT('Ctrl Pts',(2.26224148372674,635.222186336159,77.2104285068931));
#104696=CARTESIAN_POINT('Ctrl Pts',(2.24460771693217,606.490579602187,52.2254855816369));
#104697=CARTESIAN_POINT('Ctrl Pts',(2.07343281071693,605.415270650748,52.1937144269317));
#104698=CARTESIAN_POINT('Ctrl Pts',(2.33599035695507,606.116287176409,51.4023619931579));
#104699=CARTESIAN_POINT('Ctrl Pts',(1.83071110482637,606.561516929231,52.1485430639731));
#104700=CARTESIAN_POINT('Ctrl Pts',(1.68007361161791,605.466527844934,52.1267455450031));
#104701=CARTESIAN_POINT('Ctrl Pts',(1.90524322641147,606.18909600954,51.3201743394751));
#104702=CARTESIAN_POINT('Ctrl Pts',(1.4117809341791,606.614210803789,52.0926096107404));
#104703=CARTESIAN_POINT('Ctrl Pts',(1.29419848644613,605.502435858175,52.0803434838521));
#104704=CARTESIAN_POINT('Ctrl Pts',(1.46925731178754,606.24318012425,51.2604278885439));
#104705=CARTESIAN_POINT('Ctrl Pts',(0.571402625536841,606.678278971782,
52.0248171104673));
#104706=CARTESIAN_POINT('Ctrl Pts',(0.520642208727856,605.546380848727,
52.0235847625472));
#104707=CARTESIAN_POINT('Ctrl Pts',(0.594665493514755,606.308938586082,
51.1880140002959));
#104708=CARTESIAN_POINT('Ctrl Pts',(0.147816545353252,606.690126236152,
52.0124327336182));
#104709=CARTESIAN_POINT('Ctrl Pts',(0.136056956437473,605.554217188149,
52.0135137672583));
#104710=CARTESIAN_POINT('Ctrl Pts',(0.153834462869262,606.321098408993,
51.1747853911568));
#104711=CARTESIAN_POINT('Ctrl Pts',(-1.10247193645471,606.664100819198,
52.0398201590788));
#104712=CARTESIAN_POINT('Ctrl Pts',(-1.00747162781075,605.536569413224,
52.0362579003525));
#104713=CARTESIAN_POINT('Ctrl Pts',(-1.1473556856947,606.294386372217,51.2040398030431));
#104714=CARTESIAN_POINT('Ctrl Pts',(-1.91894009807577,606.566082886454,
52.1416799438264));
#104715=CARTESIAN_POINT('Ctrl Pts',(-1.74120896424276,605.474267321815,
52.1156863094179));
#104716=CARTESIAN_POINT('Ctrl Pts',(-1.99706350164218,606.193782567993,
51.3128431956377));
#104717=CARTESIAN_POINT('Ctrl Pts',(-3.12055673201112,606.318092543604,
52.414597409285));
#104718=CARTESIAN_POINT('Ctrl Pts',(-2.89662070513932,605.291084177624,
52.3569131035478));
#104719=CARTESIAN_POINT('Ctrl Pts',(-3.24760126429163,605.939249412698,
51.6043655628081));
#104720=CARTESIAN_POINT('Ctrl Pts',(-3.51645511552272,606.218600960739,
52.5259194378218));
#104721=CARTESIAN_POINT('Ctrl Pts',(-3.27570850901756,605.217611702361,
52.4544566039408));
#104722=CARTESIAN_POINT('Ctrl Pts',(-3.65961769328675,605.837132947776,
51.7232764264806));
#104723=CARTESIAN_POINT('Ctrl Pts',(-4.28117411180073,605.996930430144,
52.7819398834267));
#104724=CARTESIAN_POINT('Ctrl Pts',(-4.01998858621205,605.047219933437,
52.6857610821952));
#104725=CARTESIAN_POINT('Ctrl Pts',(-4.45547060211493,605.609614012752,
51.9967499482209));
#104726=CARTESIAN_POINT('Ctrl Pts',(-4.6527703895603,605.874231236671,52.9272079191087));
#104727=CARTESIAN_POINT('Ctrl Pts',(-4.38560256268003,604.951231636046,
52.8180868283054));
#104728=CARTESIAN_POINT('Ctrl Pts',(-4.84219570557192,605.48367760779,52.151921010376));
#104729=CARTESIAN_POINT('Ctrl Pts',(-5.73871252059238,605.479249839438,
53.412985235997));
#104730=CARTESIAN_POINT('Ctrl Pts',(-5.4476923690426,604.63808036228,53.2632683827815));
#104731=CARTESIAN_POINT('Ctrl Pts',(-5.97234965215429,605.078275357558,
52.6708141112791));
#104732=CARTESIAN_POINT('Ctrl Pts',(-6.42887593638937,605.1779005738,53.8068469880404));
#104733=CARTESIAN_POINT('Ctrl Pts',(-6.15032378335568,604.387232577824,
53.6342198283954));
#104734=CARTESIAN_POINT('Ctrl Pts',(-6.69061225764372,604.76897540853,53.0915259083752));
#104735=CARTESIAN_POINT('Ctrl Pts',(-7.70252122853823,604.561235669124,
54.7027643205653));
#104736=CARTESIAN_POINT('Ctrl Pts',(-7.45997458021475,603.85165390012,54.5105690457221));
#104737=CARTESIAN_POINT('Ctrl Pts',(-8.01611292013624,604.136040375022,
54.0485198842105));
#104738=CARTESIAN_POINT('Ctrl Pts',(-8.29093833512779,604.244338805801,
55.2059626243289));
#104739=CARTESIAN_POINT('Ctrl Pts',(-8.07548401458598,603.569173703309,
55.0065471941012));
#104740=CARTESIAN_POINT('Ctrl Pts',(-8.62848726547417,603.810782416311,
54.5860224232522));
#104741=CARTESIAN_POINT('Ctrl Pts',(-9.10615860494566,603.778412499685,
56.0502090602173));
#104742=CARTESIAN_POINT('Ctrl Pts',(-8.9398032232744,603.140516306416,55.8666947129738));
#104743=CARTESIAN_POINT('Ctrl Pts',(-9.47689944401278,603.332562709797,
55.4878240797596));
#104744=CARTESIAN_POINT('Ctrl Pts',(-9.36580248126736,603.624999032665,
56.3462294979683));
#104745=CARTESIAN_POINT('Ctrl Pts',(-9.21205942946592,603.000306548777,
56.164626520581));
#104746=CARTESIAN_POINT('Ctrl Pts',(-9.74711472218158,603.175101506797,
55.8040251608737));
#104747=CARTESIAN_POINT('Ctrl Pts',(-9.85277663850557,603.330293092108,
56.9581425734283));
#104748=CARTESIAN_POINT('Ctrl Pts',(-9.72214071534079,602.729842450111,
56.7828136529411));
#104749=CARTESIAN_POINT('Ctrl Pts',(-10.2539160475817,602.872619902042,
56.4576543706004));
#104750=CARTESIAN_POINT('Ctrl Pts',(-10.0814069885409,603.188255003849,
57.2753308908016));
#104751=CARTESIAN_POINT('Ctrl Pts',(-9.96275939343529,602.598386052796,
57.1043691500725));
#104752=CARTESIAN_POINT('Ctrl Pts',(-10.4918551409475,602.726834194727,
56.7964665120035));
#104753=CARTESIAN_POINT('Ctrl Pts',(-10.7230189007579,602.782272634049,
58.2619328657199));
#104754=CARTESIAN_POINT('Ctrl Pts',(-10.6285633925526,602.226447870635,
58.0946841395296));
#104755=CARTESIAN_POINT('Ctrl Pts',(-11.1595901762937,602.310140320832,
57.8503282493184));
#104756=CARTESIAN_POINT('Ctrl Pts',(-11.0923717675951,602.53821372029,58.9658852559509));
#104757=CARTESIAN_POINT('Ctrl Pts',(-11.0225929845114,601.995293533381,
58.8154970554682));
#104758=CARTESIAN_POINT('Ctrl Pts',(-11.543981587863,602.059641903912,58.6022718329819));
#104759=CARTESIAN_POINT('Ctrl Pts',(-11.7014944118088,602.128287009942,
60.4833358094967));
#104760=CARTESIAN_POINT('Ctrl Pts',(-11.6644122825579,601.609897417614,
60.3684103254258));
#104761=CARTESIAN_POINT('Ctrl Pts',(-12.1779050110386,601.638899407267,
60.223173033479));
#104762=CARTESIAN_POINT('Ctrl Pts',(-11.9301672368271,601.969960747067,
61.2707799874375));
#104763=CARTESIAN_POINT('Ctrl Pts',(-11.9096549681383,601.457770511395,
61.182086329466));
#104764=CARTESIAN_POINT('Ctrl Pts',(-12.4158885617532,601.476395657792,
61.0643007636695));
#104765=CARTESIAN_POINT('Ctrl Pts',(-12.1537770914997,601.814426617082,
62.4895659620246));
#104766=CARTESIAN_POINT('Ctrl Pts',(-12.1464642268629,601.309960957834,
62.4384492041064));
#104767=CARTESIAN_POINT('Ctrl Pts',(-12.6486028978816,601.316757776551,
62.3661767157842));
#104768=CARTESIAN_POINT('Ctrl Pts',(-12.2085200304299,601.776102115745,
62.9037553260946));
#104769=CARTESIAN_POINT('Ctrl Pts',(-12.2044669680803,601.273482834465,
62.864765245725));
#104770=CARTESIAN_POINT('Ctrl Pts',(-12.7055747490575,601.277422086745,
62.808603167802));
#104771=CARTESIAN_POINT('Ctrl Pts',(-12.2753636450861,601.729264950609,
63.7414063290601));
#104772=CARTESIAN_POINT('Ctrl Pts',(-12.274978483213,601.229090042892,63.7252770410462));
#104773=CARTESIAN_POINT('Ctrl Pts',(-12.7751399565671,601.229349134952,
63.7033604237967));
#104774=CARTESIAN_POINT('Ctrl Pts',(-12.2870666679087,601.721034202814,
64.1583756132804));
#104775=CARTESIAN_POINT('Ctrl Pts',(-12.2873846747713,601.221245455343,
64.1547225574821));
#104776=CARTESIAN_POINT('Ctrl Pts',(-12.787319479616,601.220901219213,64.148756333092));
#104777=CARTESIAN_POINT('Ctrl Pts',(-12.268530884661,601.734042938711,64.9887244061267));
#104778=CARTESIAN_POINT('Ctrl Pts',(-12.2678309313976,601.233579222809,
65.0078610328854));
#104779=CARTESIAN_POINT('Ctrl Pts',(-12.7680289967845,601.234253187538,
65.0357135662794));
#104780=CARTESIAN_POINT('Ctrl Pts',(-12.238288133047,601.755284556781,65.4021035317435));
#104781=CARTESIAN_POINT('Ctrl Pts',(-12.235780004542,601.253813861924,65.4335305959216));
#104782=CARTESIAN_POINT('Ctrl Pts',(-12.7365548811428,601.256055263972,
65.4772745550034));
#104783=CARTESIAN_POINT('Ctrl Pts',(-12.1360079708598,601.82677612692,66.2252982180572));
#104784=CARTESIAN_POINT('Ctrl Pts',(-12.1278948320545,601.321540940876,
66.2789946000502));
#104785=CARTESIAN_POINT('Ctrl Pts',(-12.6301103000015,601.329433121089,
66.3565899298897));
#104786=CARTESIAN_POINT('Ctrl Pts',(-12.0634251058667,601.877406103097,
66.6373579383003));
#104787=CARTESIAN_POINT('Ctrl Pts',(-12.0509917691496,601.369699169805,
66.7029848588286));
#104788=CARTESIAN_POINT('Ctrl Pts',(-12.5545721539083,601.381398964076,
66.7967415398965));
#104789=CARTESIAN_POINT('Ctrl Pts',(-11.7851849710258,602.069970646424,
67.8517603894219));
#104790=CARTESIAN_POINT('Ctrl Pts',(-11.7560671806612,601.552702929143,
67.9555151604994));
#104791=CARTESIAN_POINT('Ctrl Pts',(-12.265003213869,601.57904430758,68.0939351245997));
#104792=CARTESIAN_POINT('Ctrl Pts',(-11.5231511655743,602.249959959671,
68.6226018819362));
#104793=CARTESIAN_POINT('Ctrl Pts',(-11.4753688142236,601.725181838547,
68.7506469944195));
#104794=CARTESIAN_POINT('Ctrl Pts',(-11.9923003685254,601.763782683624,
68.9173282151888));
#104795=CARTESIAN_POINT('Ctrl Pts',(-11.0237873908383,602.582434476172,
69.7270719203858));
#104796=CARTESIAN_POINT('Ctrl Pts',(-10.9544028777391,602.034097575223,
69.8689551387738));
#104797=CARTESIAN_POINT('Ctrl Pts',(-11.4726049050073,602.105029318799,
70.0970939152249));
#104798=CARTESIAN_POINT('Ctrl Pts',(-10.8384310991565,602.704379416319,
70.0880515743831));
#104799=CARTESIAN_POINT('Ctrl Pts',(-10.7586359325232,602.148519598434,
70.237687260735));
#104800=CARTESIAN_POINT('Ctrl Pts',(-11.2797017252308,602.230191744764,
70.4826829420179));
#104801=CARTESIAN_POINT('Ctrl Pts',(-10.4390987804155,602.96227503081,70.7805569003536));
#104802=CARTESIAN_POINT('Ctrl Pts',(-10.3387444088613,602.388767014119,
70.9429750385828));
#104803=CARTESIAN_POINT('Ctrl Pts',(-10.8641104504998,602.494891833565,
71.2223989202368));
#104804=CARTESIAN_POINT('Ctrl Pts',(-10.2247929217345,603.098466179307,
71.1132662015513));
#104805=CARTESIAN_POINT('Ctrl Pts',(-10.112915332954,602.51548143905,71.2812239398437));
#104806=CARTESIAN_POINT('Ctrl Pts',(-10.6410790491553,602.634676338017,
71.5777902117513));
#104807=CARTESIAN_POINT('Ctrl Pts',(-9.76784625223807,603.382222667475,
71.7535556942923));
#104808=CARTESIAN_POINT('Ctrl Pts',(-9.63349659380942,602.777474712516,
71.9302320108111));
#104809=CARTESIAN_POINT('Ctrl Pts',(-10.1655277254286,602.92591960861,72.261730451579));
#104810=CARTESIAN_POINT('Ctrl Pts',(-9.52520374213731,603.529798312671,
72.0611303923611));
#104811=CARTESIAN_POINT('Ctrl Pts',(-9.37852363969346,602.9133313277,72.2410837179652));
#104812=CARTESIAN_POINT('Ctrl Pts',(-9.91300599012881,603.077388971499,
72.5902735372759));
#104813=CARTESIAN_POINT('Ctrl Pts',(-9.01135722475072,603.833330353901,
72.6522134952531));
#104814=CARTESIAN_POINT('Ctrl Pts',(-8.84120033390601,603.190288416632,
72.836293304798));
#104815=CARTESIAN_POINT('Ctrl Pts',(-9.37823825283678,603.388929535203,
73.2216526442934));
#104816=CARTESIAN_POINT('Ctrl Pts',(-8.7389100250046,603.989962358859,72.9367840692432));
#104817=CARTESIAN_POINT('Ctrl Pts',(-8.55620892724536,603.332406057612,
73.1214587846384));
#104818=CARTESIAN_POINT('Ctrl Pts',(-9.09469840048593,603.549694184874,
73.5256232407945));
#104819=CARTESIAN_POINT('Ctrl Pts',(-7.89012810647256,604.46027386765,73.7426824430362));
#104820=CARTESIAN_POINT('Ctrl Pts',(-7.65796125292146,603.762076285552,
73.9394272155619));
#104821=CARTESIAN_POINT('Ctrl Pts',(-8.21135820442717,604.032414773745,
74.3864623908746));
#104822=CARTESIAN_POINT('Ctrl Pts',(-7.28116846417887,604.775808181103,
74.219742003199));
#104823=CARTESIAN_POINT('Ctrl Pts',(-7.02391120497901,604.039881145729,
74.4058463661051));
#104824=CARTESIAN_POINT('Ctrl Pts',(-7.57760505325563,604.356274191398,
74.8960441316923));
#104825=CARTESIAN_POINT('Ctrl Pts',(-6.29659249347781,605.228731780166,
74.8505072253373));
#104826=CARTESIAN_POINT('Ctrl Pts',(-6.03600513843954,604.420695941946,
75.0061312303154));
#104827=CARTESIAN_POINT('Ctrl Pts',(-6.55294358412831,604.821147490993,
75.5698095385058));
#104828=CARTESIAN_POINT('Ctrl Pts',(-5.95642441709213,605.376260941674,
75.0464903317535));
#104829=CARTESIAN_POINT('Ctrl Pts',(-5.69039769264683,604.544663809187,
75.1933203823609));
#104830=CARTESIAN_POINT('Ctrl Pts',(-6.19892597176367,604.972569034461,
75.7791531330914));
#104831=CARTESIAN_POINT('Ctrl Pts',(-5.24924375098352,605.659381288065,
75.4090550759564));
#104832=CARTESIAN_POINT('Ctrl Pts',(-4.97872636614062,604.778612595241,
75.5368081438878));
#104833=CARTESIAN_POINT('Ctrl Pts',(-5.46295346090092,605.263159156084,
76.166434449957));
#104834=CARTESIAN_POINT('Ctrl Pts',(-4.88532837447767,605.793622011102,
75.5738955184618));
#104835=CARTESIAN_POINT('Ctrl Pts',(-4.61623378897079,604.886539446989,
75.6897044857469));
#104836=CARTESIAN_POINT('Ctrl Pts',(-5.084221879631,605.400941617948,76.3425122362357));
#104837=CARTESIAN_POINT('Ctrl Pts',(-3.77089077493721,606.162783667258,
76.0143384748105));
#104838=CARTESIAN_POINT('Ctrl Pts',(-3.49682383912046,605.183694534843,
76.1025288496454));
#104839=CARTESIAN_POINT('Ctrl Pts',(-3.92441156002437,605.779843200399,
76.812980796566));
#104840=CARTESIAN_POINT('Ctrl Pts',(-2.99381238346118,606.366311081735,
76.238938541679));
#104841=CARTESIAN_POINT('Ctrl Pts',(-2.75796680224509,605.329065112758,
76.2927147804116));
#104842=CARTESIAN_POINT('Ctrl Pts',(-3.11569968988111,605.988739624887,
77.0528911109046));
#104843=CARTESIAN_POINT('Ctrl Pts',(-2.17374385871217,606.502538120315,
76.3864215127495));
#104844=CARTESIAN_POINT('Ctrl Pts',(-2.00694303543426,605.423796482346,
76.4163679119408));
#104845=CARTESIAN_POINT('Ctrl Pts',(-2.26224148372674,606.128561192588,
77.2104285068931));
#104846=CARTESIAN_POINT('Ctrl Pts',(2.31092134190292,606.120502424978,51.3976052199539));
#104847=CARTESIAN_POINT('Ctrl Pts',(1.9243904261614,606.185154402164,51.3246699561266));
#104848=CARTESIAN_POINT('Ctrl Pts',(1.53337526913546,606.234741119557,51.2697641942173));
#104849=CARTESIAN_POINT('Ctrl Pts',(1.13772717179832,606.267659184254,51.2334761581271));
#104850=CARTESIAN_POINT('Ctrl Pts',(1.10108396594791,606.270707912225,51.2301153180641));
#104851=CARTESIAN_POINT('Ctrl Pts',(1.06440101544787,606.273613684272,51.2269141451144));
#104852=CARTESIAN_POINT('Ctrl Pts',(1.02767819909564,606.276375240354,51.223873088555));
#104853=CARTESIAN_POINT('Ctrl Pts',(1.02189271947807,606.276810308468,51.2233939866645));
#104854=CARTESIAN_POINT('Ctrl Pts',(1.01610581480731,606.277241740565,51.2229189177151));
#104855=CARTESIAN_POINT('Ctrl Pts',(1.01031752097323,606.277669534987,51.2224478826357));
#104856=CARTESIAN_POINT('Ctrl Pts',(0.769279298806018,606.295483904812,
51.2028328697541));
#104857=CARTESIAN_POINT('Ctrl Pts',(0.525719603105276,606.306988425792,
51.1902149545468));
#104858=CARTESIAN_POINT('Ctrl Pts',(0.282374958379684,606.312048295433,
51.1846774469339));
#104859=CARTESIAN_POINT('Ctrl Pts',(0.0944016631504275,606.315956827592,
51.180399959938));
#104860=CARTESIAN_POINT('Ctrl Pts',(-0.0934423284468907,606.316020562991,
51.1803465302694));
#104861=CARTESIAN_POINT('Ctrl Pts',(-0.279895468563284,606.312191712354,
51.1845398016811));
#104862=CARTESIAN_POINT('Ctrl Pts',(-0.291911936050446,606.311944951913,
51.1848100481868));
#104863=CARTESIAN_POINT('Ctrl Pts',(-0.303924672822357,606.311682308102,
51.1850974258479));
#104864=CARTESIAN_POINT('Ctrl Pts',(-0.315933663727288,606.311403820519,
51.1854019212719));
#104865=CARTESIAN_POINT('Ctrl Pts',(-0.743857359011278,606.301480302683,
51.19625219238));
#104866=CARTESIAN_POINT('Ctrl Pts',(-1.16718217071824,606.271434870956,
51.2288431932868));
#104867=CARTESIAN_POINT('Ctrl Pts',(-1.58621543213723,606.222982509351,
51.2826473556403));
#104868=CARTESIAN_POINT('Ctrl Pts',(-2.00524869355621,606.174530147747,
51.3364515179938));
#104869=CARTESIAN_POINT('Ctrl Pts',(-2.41999047219477,606.107670585567,
51.4114688925646));
#104870=CARTESIAN_POINT('Ctrl Pts',(-2.83074822463685,606.024078269923,
51.5072092257538));
#104871=CARTESIAN_POINT('Ctrl Pts',(-2.85311152071182,606.019527169687,
51.5124217126872));
#104872=CARTESIAN_POINT('Ctrl Pts',(-2.87546063135743,606.014926459225,
51.5176966435968));
#104873=CARTESIAN_POINT('Ctrl Pts',(-2.89779414296661,606.010277010054,
51.5230334110954));
#104874=CARTESIAN_POINT('Ctrl Pts',(-3.2059760252563,605.94611889545,51.5966758853213));
#104875=CARTESIAN_POINT('Ctrl Pts',(-3.51096003016406,605.872712309442,
51.6820570658823));
#104876=CARTESIAN_POINT('Ctrl Pts',(-3.80902312883169,605.79238337635,51.7775305592681));
#104877=CARTESIAN_POINT('Ctrl Pts',(-3.8924315663616,605.769904542748,51.8042473683747));
#104878=CARTESIAN_POINT('Ctrl Pts',(-3.97529830179592,605.746883489111,
51.8317545824747));
#104879=CARTESIAN_POINT('Ctrl Pts',(-4.0575423502046,605.723370840561,51.8600163602557));
#104880=CARTESIAN_POINT('Ctrl Pts',(-4.0832488854947,605.716021631209,51.8688499768145));
#104881=CARTESIAN_POINT('Ctrl Pts',(-4.10890664396029,605.708622165367,
51.8777598513787));
#104882=CARTESIAN_POINT('Ctrl Pts',(-4.1345159694774,605.701173272842,51.8867457715322));
#104883=CARTESIAN_POINT('Ctrl Pts',(-4.42402771904677,605.616964030161,
51.9883310109953));
#104884=CARTESIAN_POINT('Ctrl Pts',(-4.70743818532932,605.526409127712,
52.0996719099263));
#104885=CARTESIAN_POINT('Ctrl Pts',(-4.9850704927822,605.430758867119,52.2203911199615));
#104886=CARTESIAN_POINT('Ctrl Pts',(-5.06347338639407,605.403747395457,
52.2544820205059));
#104887=CARTESIAN_POINT('Ctrl Pts',(-5.14141563704577,605.376329658806,
52.2893205600599));
#104888=CARTESIAN_POINT('Ctrl Pts',(-5.21890487245671,605.348533964113,
52.3248976144887));
#104889=CARTESIAN_POINT('Ctrl Pts',(-5.24645122189632,605.338652979808,
52.3375447643557));
#104890=CARTESIAN_POINT('Ctrl Pts',(-5.27394681459037,605.32872123747,52.3502900634044));
#104891=CARTESIAN_POINT('Ctrl Pts',(-5.30139053208202,605.318740404161,
52.3631325099366));
#104892=CARTESIAN_POINT('Ctrl Pts',(-5.66366362029746,605.186987579246,
52.5326602995615));
#104893=CARTESIAN_POINT('Ctrl Pts',(-6.01738163217701,605.04648601964,52.7193702986017));
#104894=CARTESIAN_POINT('Ctrl Pts',(-6.36015875743499,604.900894357318,
52.9212117806643));
#104895=CARTESIAN_POINT('Ctrl Pts',(-6.66684957126459,604.770630048196,
53.101804135979));
#104896=CARTESIAN_POINT('Ctrl Pts',(-6.96478180974465,604.636292006874,
53.2945085964751));
#104897=CARTESIAN_POINT('Ctrl Pts',(-7.25228682885563,604.500486505444,
53.4978360666795));
#104898=CARTESIAN_POINT('Ctrl Pts',(-7.28611567272387,604.484507156219,
53.521760286385));
#104899=CARTESIAN_POINT('Ctrl Pts',(-7.3198002059198,604.468507463044,53.5458315631905));
#104900=CARTESIAN_POINT('Ctrl Pts',(-7.35333775249021,604.452491647418,
53.5700474603555));
#104901=CARTESIAN_POINT('Ctrl Pts',(-7.38103000654065,604.439267244309,
53.5900427445945));
#104902=CARTESIAN_POINT('Ctrl Pts',(-7.40863101404046,604.426029015268,
53.6101387611508));
#104903=CARTESIAN_POINT('Ctrl Pts',(-7.43614101292809,604.412778123398,
53.6303357171612));
#104904=CARTESIAN_POINT('Ctrl Pts',(-7.75229632205407,604.260493863682,
53.8624467723796));
#104905=CARTESIAN_POINT('Ctrl Pts',(-8.05648904258559,604.106536505203,
54.1078905944877));
#104906=CARTESIAN_POINT('Ctrl Pts',(-8.3492945393904,603.952529481828,54.3671926590542));
#104907=CARTESIAN_POINT('Ctrl Pts',(-8.64210003619521,603.798522458454,
54.6264947236207));
#104908=CARTESIAN_POINT('Ctrl Pts',(-8.9235180189489,603.644464962219,54.8996548343146));
#104909=CARTESIAN_POINT('Ctrl Pts',(-9.1940846406694,603.491964984821,55.1872316250658));
#104910=CARTESIAN_POINT('Ctrl Pts',(-9.21816683588502,603.478391491525,
55.2128278363438));
#104911=CARTESIAN_POINT('Ctrl Pts',(-9.24215653499197,603.464832754806,
55.2385359314634));
#104912=CARTESIAN_POINT('Ctrl Pts',(-9.26605121704545,603.451291368523,
55.2643528781629));
#104913=CARTESIAN_POINT('Ctrl Pts',(-9.44919177121111,603.34750354735,55.4622266106876));
#104914=CARTESIAN_POINT('Ctrl Pts',(-9.62656991926582,603.244837575087,
55.6662959234923));
#104915=CARTESIAN_POINT('Ctrl Pts',(-9.79718029226227,603.144395450504,
55.8752912389312));
#104916=CARTESIAN_POINT('Ctrl Pts',(-9.86608440423407,603.103830065895,
55.9596978102531));
#104917=CARTESIAN_POINT('Ctrl Pts',(-9.93388438714588,603.063627351038,
56.0449084297711));
#104918=CARTESIAN_POINT('Ctrl Pts',(-10.0005127777516,603.02385991362,56.1308414745918));
#104919=CARTESIAN_POINT('Ctrl Pts',(-10.0215035613001,603.011331475464,
56.1579140472159));
#104920=CARTESIAN_POINT('Ctrl Pts',(-10.042387340134,602.998840989267,56.1850678260703));
#104921=CARTESIAN_POINT('Ctrl Pts',(-10.0631644425131,602.986389115948,
56.2123033808313));
#104922=CARTESIAN_POINT('Ctrl Pts',(-10.293419592427,602.848395477299,56.5141321262486));
#104923=CARTESIAN_POINT('Ctrl Pts',(-10.5104654401652,602.71521946088,56.8258408735637));
#104924=CARTESIAN_POINT('Ctrl Pts',(-10.7144165406335,602.587932468945,
57.1477632880394));
#104925=CARTESIAN_POINT('Ctrl Pts',(-10.7319264752442,602.577004423445,
57.1754014837356));
#104926=CARTESIAN_POINT('Ctrl Pts',(-10.7493409367415,602.566119390598,
57.2031141332603));
#104927=CARTESIAN_POINT('Ctrl Pts',(-10.7666595412328,602.555278130554,
57.2309017674638));
#104928=CARTESIAN_POINT('Ctrl Pts',(-10.9204731636543,602.458992458119,
57.4776951322247));
#104929=CARTESIAN_POINT('Ctrl Pts',(-11.0666558808087,602.366227070793,
57.7302247072817));
#104930=CARTESIAN_POINT('Ctrl Pts',(-11.2050607147541,602.277439642877,
57.9890220210254));
#104931=CARTESIAN_POINT('Ctrl Pts',(-11.3377551216428,602.192315483911,
58.2371416500344));
#104932=CARTESIAN_POINT('Ctrl Pts',(-11.4633001687098,602.110847512538,
58.4910223940912));
#104933=CARTESIAN_POINT('Ctrl Pts',(-11.5815311313948,602.033455455343,
58.7511591647439));
#104934=CARTESIAN_POINT('Ctrl Pts',(-11.6797499746316,601.969163004696,
58.9672644227628));
#104935=CARTESIAN_POINT('Ctrl Pts',(-11.7729206336702,601.907683622293,
59.1876875040276));
#104936=CARTESIAN_POINT('Ctrl Pts',(-11.8609291144948,601.8492692711,59.4127277678694));
#104937=CARTESIAN_POINT('Ctrl Pts',(-11.8711982768748,601.842453263687,
59.4389863169294));
#104938=CARTESIAN_POINT('Ctrl Pts',(-11.8813850119675,601.835687125542,
59.4652785322609));
#104939=CARTESIAN_POINT('Ctrl Pts',(-11.8914892131512,601.828971113388,
59.4916044497248));
#104940=CARTESIAN_POINT('Ctrl Pts',(-11.9959186669114,601.759559443137,
59.7636894102792));
#104941=CARTESIAN_POINT('Ctrl Pts',(-12.091310776531,601.695659985364,60.0387465906123));
#104942=CARTESIAN_POINT('Ctrl Pts',(-12.1776505788867,601.637494904103,
60.3167757884128));
#104943=CARTESIAN_POINT('Ctrl Pts',(-12.2628096616721,601.580125245671,
60.5910028635999));
#104944=CARTESIAN_POINT('Ctrl Pts',(-12.3391623321425,601.528334025132,
60.8681213879226));
#104945=CARTESIAN_POINT('Ctrl Pts',(-12.4066531860926,601.482358055859,
61.1481479683393));
#104946=CARTESIAN_POINT('Ctrl Pts',(-12.4690433776644,601.439856748456,
61.4070113694502));
#104947=CARTESIAN_POINT('Ctrl Pts',(-12.5238602515823,601.402325030908,
61.6683601246001));
#104948=CARTESIAN_POINT('Ctrl Pts',(-12.5710279567737,601.369970326165,
61.9322186969404));
#104949=CARTESIAN_POINT('Ctrl Pts',(-12.5745024304964,601.367587009635,
61.9516550819074));
#104950=CARTESIAN_POINT('Ctrl Pts',(-12.5779356066442,601.365231507343,
61.9711086414617));
#104951=CARTESIAN_POINT('Ctrl Pts',(-12.5813273486773,601.362903942309,
61.9905791155502));
#104952=CARTESIAN_POINT('Ctrl Pts',(-12.6482309907147,601.316991671765,
62.3746430024895));
#104953=CARTESIAN_POINT('Ctrl Pts',(-12.6989827550363,601.281970909012,
62.7651309616918));
#104954=CARTESIAN_POINT('Ctrl Pts',(-12.7325045718852,601.258810650632,
63.1594985620737));
#104955=CARTESIAN_POINT('Ctrl Pts',(-12.7352361632934,601.256923391266,
63.1916343843564));
#104956=CARTESIAN_POINT('Ctrl Pts',(-12.7378533692347,601.255114870462,
63.2237959671349));
#104957=CARTESIAN_POINT('Ctrl Pts',(-12.7403556191587,601.25338560344,63.2559819337451));
#104958=CARTESIAN_POINT('Ctrl Pts',(-12.7415108518539,601.252587239622,
63.2708414729934));
#104959=CARTESIAN_POINT('Ctrl Pts',(-12.7426411255945,601.251806087635,
63.2856985588883));
#104960=CARTESIAN_POINT('Ctrl Pts',(-12.7437464711904,601.251042128905,
63.3005531880157));
#104961=CARTESIAN_POINT('Ctrl Pts',(-12.7759162994634,601.228807977662,
63.7328802989446));
#104962=CARTESIAN_POINT('Ctrl Pts',(-12.7870003318299,601.221122005951,
64.1634229287959));
#104963=CARTESIAN_POINT('Ctrl Pts',(-12.7776731523991,601.227577203012,
64.5922349254529));
#104964=CARTESIAN_POINT('Ctrl Pts',(-12.7774670029556,601.227719875863,
64.6017125338895));
#104965=CARTESIAN_POINT('Ctrl Pts',(-12.7772508808923,601.22786945759,64.611189296609));
#104966=CARTESIAN_POINT('Ctrl Pts',(-12.7770247866986,601.228025945988,
64.6206652136733));
#104967=CARTESIAN_POINT('Ctrl Pts',(-12.7666730268079,601.235190793079,
65.0545216369199));
#104968=CARTESIAN_POINT('Ctrl Pts',(-12.7354157605725,601.256837750184,
65.4866513230427));
#104969=CARTESIAN_POINT('Ctrl Pts',(-12.6833305290434,601.292744171308,
65.9169319880768));
#104970=CARTESIAN_POINT('Ctrl Pts',(-12.6828077078149,601.293104592845,
65.9212510600921));
#104971=CARTESIAN_POINT('Ctrl Pts',(-12.6822827336681,601.293466488472,
65.9255701772016));
#104972=CARTESIAN_POINT('Ctrl Pts',(-12.6817556078935,601.293829856882,
65.9298893314513));
#104973=CARTESIAN_POINT('Ctrl Pts',(-12.6329480531499,601.32747481301,66.3298078474378));
#104974=CARTESIAN_POINT('Ctrl Pts',(-12.5656816350128,601.37375161562,66.7301336276845));
#104975=CARTESIAN_POINT('Ctrl Pts',(-12.4809092885528,601.431669700594,
67.1247607526229));
#104976=CARTESIAN_POINT('Ctrl Pts',(-12.4735560157333,601.436693596921,
67.1589912656718));
#104977=CARTESIAN_POINT('Ctrl Pts',(-12.4660710046774,601.441805097326,
67.1931788821502));
#104978=CARTESIAN_POINT('Ctrl Pts',(-12.4584548648209,601.447003563173,
67.2273196043471));
#104979=CARTESIAN_POINT('Ctrl Pts',(-12.4583195473824,601.447095925327,
67.2279261892));
#104980=CARTESIAN_POINT('Ctrl Pts',(-12.4581841884965,601.447188314965,
67.228532759456));
#104981=CARTESIAN_POINT('Ctrl Pts',(-12.4580487881665,601.447280732084,
67.2291393150922));
#104982=CARTESIAN_POINT('Ctrl Pts',(-12.3287543192927,601.535530312215,
67.8083423998814));
#104983=CARTESIAN_POINT('Ctrl Pts',(-12.1635881081911,601.647634844985,
68.3695526414148));
#104984=CARTESIAN_POINT('Ctrl Pts',(-11.9641361654503,601.780646951911,
68.914015787099));
#104985=CARTESIAN_POINT('Ctrl Pts',(-11.8692267000605,601.843940935339,
69.1730992804518));
#104986=CARTESIAN_POINT('Ctrl Pts',(-11.7665541541683,601.911968557483,
69.4283910409647));
#104987=CARTESIAN_POINT('Ctrl Pts',(-11.6562914846912,601.984409339138,
69.6800273323468));
#104988=CARTESIAN_POINT('Ctrl Pts',(-11.6528123180314,601.986695095083,
69.6879673232751));
#104989=CARTESIAN_POINT('Ctrl Pts',(-11.6493255850375,601.988985246907,
69.6959036824858));
#104990=CARTESIAN_POINT('Ctrl Pts',(-11.6458312910721,601.991279784524,
69.703836414217));
#104991=CARTESIAN_POINT('Ctrl Pts',(-11.4971366810285,602.088920503827,
70.0414023039313));
#104992=CARTESIAN_POINT('Ctrl Pts',(-11.3338413939608,602.195038107293,
70.3735482479391));
#104993=CARTESIAN_POINT('Ctrl Pts',(-11.1589239951637,602.306981469902,
70.6951271372583));
#104994=CARTESIAN_POINT('Ctrl Pts',(-11.1357897460821,602.321786890355,
70.7376585616681));
#104995=CARTESIAN_POINT('Ctrl Pts',(-11.1124522363448,602.336694184926,
70.7800050874247));
#104996=CARTESIAN_POINT('Ctrl Pts',(-11.08891838951,602.351697191721,70.8221547543116));
#104997=CARTESIAN_POINT('Ctrl Pts',(-11.0832572973831,602.355306181115,
70.8322939019419));
#104998=CARTESIAN_POINT('Ctrl Pts',(-11.0775847776858,602.358920761129,
70.8424218051789));
#104999=CARTESIAN_POINT('Ctrl Pts',(-11.0719009273916,602.362540845218,
70.8525382931254));
#105000=CARTESIAN_POINT('Ctrl Pts',(-10.8933793466742,602.476242491184,
71.1702826611247));
#105001=CARTESIAN_POINT('Ctrl Pts',(-10.703424027174,602.595558323103,71.4776963876999));
#105002=CARTESIAN_POINT('Ctrl Pts',(-10.5023371611635,602.719460142399,
71.7752823630464));
#105003=CARTESIAN_POINT('Ctrl Pts',(-10.477246088423,602.734920274741,71.812414332439));
#105004=CARTESIAN_POINT('Ctrl Pts',(-10.451981746354,602.750451775019,71.849393329467));
#105005=CARTESIAN_POINT('Ctrl Pts',(-10.4265447575929,602.766052618462,
71.8862203643523));
#105006=CARTESIAN_POINT('Ctrl Pts',(-10.4188131204951,602.770794534301,
71.89741403479));
#105007=CARTESIAN_POINT('Ctrl Pts',(-10.4110654988077,602.775542877077,
71.9085937144694));
#105008=CARTESIAN_POINT('Ctrl Pts',(-10.403301906923,602.780297592492,71.9197594373552));
#105009=CARTESIAN_POINT('Ctrl Pts',(-10.1743043134857,602.9205443241,72.249107464377));
#105010=CARTESIAN_POINT('Ctrl Pts',(-9.9314107080512,603.066346344098,72.5663065584189));
#105011=CARTESIAN_POINT('Ctrl Pts',(-9.67444603037874,603.216348882047,
72.8718105219763));
#105012=CARTESIAN_POINT('Ctrl Pts',(-9.66485722564934,603.221946324693,
72.8832106018516));
#105013=CARTESIAN_POINT('Ctrl Pts',(-9.65524877276323,603.227549638817,
72.894594446214));
#105014=CARTESIAN_POINT('Ctrl Pts',(-9.64562066556107,603.233158751113,
72.9059620729246));
#105015=CARTESIAN_POINT('Ctrl Pts',(-9.42731586110791,603.360338074853,
73.1637082190824));
#105016=CARTESIAN_POINT('Ctrl Pts',(-9.19804063689573,603.490962988956,
73.4138743236315));
#105017=CARTESIAN_POINT('Ctrl Pts',(-8.9606618592393,603.62236653666,73.6534663851397));
#105018=CARTESIAN_POINT('Ctrl Pts',(-8.91843648223493,603.645740843312,
73.6960854651785));
#105019=CARTESIAN_POINT('Ctrl Pts',(-8.87595480166585,603.669139715431,
73.7383699342028));
#105020=CARTESIAN_POINT('Ctrl Pts',(-8.83323308819527,603.692548054781,
73.7803029115011));
#105021=CARTESIAN_POINT('Ctrl Pts',(-8.82225322068705,603.698564210122,
73.7910800666655));
#105022=CARTESIAN_POINT('Ctrl Pts',(-8.8112573568705,603.704581075414,73.8018341562657));
#105023=CARTESIAN_POINT('Ctrl Pts',(-8.80024576806367,603.710598396771,
73.8125648963688));
#105024=CARTESIAN_POINT('Ctrl Pts',(-8.45642397178709,603.898481024225,
74.1476175760816));
#105025=CARTESIAN_POINT('Ctrl Pts',(-8.09685247605963,604.087315619871,
74.4611950419538));
#105026=CARTESIAN_POINT('Ctrl Pts',(-7.72053287891659,604.273894779001,
74.7538975280105));
#105027=CARTESIAN_POINT('Ctrl Pts',(-7.46460285154065,604.400784820516,
74.9529606537106));
#105028=CARTESIAN_POINT('Ctrl Pts',(-7.20092632696537,604.526630672235,
75.1423691922054));
#105029=CARTESIAN_POINT('Ctrl Pts',(-6.92918660057972,604.650411262877,
75.3223177033401));
#105030=CARTESIAN_POINT('Ctrl Pts',(-6.91763580200879,604.655672785322,
75.3299667469043));
#105031=CARTESIAN_POINT('Ctrl Pts',(-6.90607038322324,604.660930574261,
75.3375986977517));
#105032=CARTESIAN_POINT('Ctrl Pts',(-6.89449031796784,604.666184552022,
75.3452135726448));
#105033=CARTESIAN_POINT('Ctrl Pts',(-6.56315230202821,604.816515532802,
75.5630964155351));
#105034=CARTESIAN_POINT('Ctrl Pts',(-6.21970864445251,604.963681647969,
75.7668655454909));
#105035=CARTESIAN_POINT('Ctrl Pts',(-5.86266390244237,605.105307310949,
75.9560400598351));
#105036=CARTESIAN_POINT('Ctrl Pts',(-5.85210062245604,605.109497350335,
75.9616368468093));
#105037=CARTESIAN_POINT('Ctrl Pts',(-5.84152543830141,605.113682529787,
75.9672208471966));
#105038=CARTESIAN_POINT('Ctrl Pts',(-5.83093831658856,605.11786278462,75.9727920447534));
#105039=CARTESIAN_POINT('Ctrl Pts',(-5.5161673445808,605.242148016517,76.1384320853383));
#105040=CARTESIAN_POINT('Ctrl Pts',(-5.19319897990937,605.361066290119,
76.2913913408696));
#105041=CARTESIAN_POINT('Ctrl Pts',(-4.86393313325879,605.472044352162,
76.4304781401722));
#105042=CARTESIAN_POINT('Ctrl Pts',(-4.81686179186501,605.487909606025,
76.4503617760851));
#105043=CARTESIAN_POINT('Ctrl Pts',(-4.76966181409826,605.503612582643,
76.4699619551291));
#105044=CARTESIAN_POINT('Ctrl Pts',(-4.72233881323819,605.519145766855,
76.4892752541632));
#105045=CARTESIAN_POINT('Ctrl Pts',(-4.71410218547921,605.521849337084,
76.4926367581264));
#105046=CARTESIAN_POINT('Ctrl Pts',(-4.70586176397251,605.524547786911,
76.4959896003441));
#105047=CARTESIAN_POINT('Ctrl Pts',(-4.69761757561064,605.527241077286,
76.4993337633958));
#105048=CARTESIAN_POINT('Ctrl Pts',(-4.3388302553356,605.644453153712,76.6448718378807));
#105049=CARTESIAN_POINT('Ctrl Pts',(-3.9720449954439,605.752375348195,76.7746808977428));
#105050=CARTESIAN_POINT('Ctrl Pts',(-3.59624449105719,605.848408824589,
76.8878059230058));
#105051=CARTESIAN_POINT('Ctrl Pts',(-3.23104131746731,605.941734219155,
76.9977408958338));
#105052=CARTESIAN_POINT('Ctrl Pts',(-2.85732420839845,606.023832093733,
77.0919195272477));
#105053=CARTESIAN_POINT('Ctrl Pts',(-2.47414214786944,606.092277286236,
77.1694416309688));
#105054=CARTESIAN_POINT('Ctrl Pts',(-2.40382931965833,606.104836786166,
77.1836667185264));
#105055=CARTESIAN_POINT('Ctrl Pts',(-2.33319774596395,606.116936468902,
77.1973308944953));
#105056=CARTESIAN_POINT('Ctrl Pts',(-2.26224148372675,606.128561192588,
77.2104285068931));
#105057=CARTESIAN_POINT('Ctrl Pts',(-31.0097671277257,639.446460969661,
66.0551195689836));
#105058=CARTESIAN_POINT('Ctrl Pts',(-30.8959801896217,640.044390291998,
66.0811757608045));
#105059=CARTESIAN_POINT('Ctrl Pts',(-31.4793952064496,640.026746757976,
66.2557082786456));
#105060=CARTESIAN_POINT('Ctrl Pts',(-31.1216215713103,639.485438110803,
65.6842493861687));
#105061=CARTESIAN_POINT('Ctrl Pts',(-31.011297302018,640.078355022162,65.7082942948574));
#105062=CARTESIAN_POINT('Ctrl Pts',(-31.6011050878646,640.068535529554,
65.8424727426508));
#105063=CARTESIAN_POINT('Ctrl Pts',(-31.199678803567,639.513756569195,65.2913781212572));
#105064=CARTESIAN_POINT('Ctrl Pts',(-31.0932130181999,640.10348882227,65.308332916704));
#105065=CARTESIAN_POINT('Ctrl Pts',(-31.6860601122613,640.098849863563,
65.4047068941051));
#105066=CARTESIAN_POINT('Ctrl Pts',(-31.2763918246953,639.541623224254,
64.5136325787294));
#105067=CARTESIAN_POINT('Ctrl Pts',(-31.173175859161,640.12806781138,64.5180893199653));
#105068=CARTESIAN_POINT('Ctrl Pts',(-31.7695504886776,640.128678316087,
64.5381010125616));
#105069=CARTESIAN_POINT('Ctrl Pts',(-31.2776919379551,639.542105193104,
64.127368726076));
#105070=CARTESIAN_POINT('Ctrl Pts',(-31.174545243998,640.128497521662,64.1236757188328));
#105071=CARTESIAN_POINT('Ctrl Pts',(-31.7709656050263,640.129193814483,
64.1077050217475));
#105072=CARTESIAN_POINT('Ctrl Pts',(-31.224600053557,639.522805357793,63.5480361507529));
#105073=CARTESIAN_POINT('Ctrl Pts',(-31.1192510473443,640.111488697363,
63.5355366548963));
#105074=CARTESIAN_POINT('Ctrl Pts',(-31.7131830184482,640.108535850692,
63.4621815431067));
#105075=CARTESIAN_POINT('Ctrl Pts',(-31.1974309863985,639.512951461025,
63.3538641004119));
#105076=CARTESIAN_POINT('Ctrl Pts',(-31.0908849094541,640.102784037384,
63.3381669310628));
#105077=CARTESIAN_POINT('Ctrl Pts',(-31.6836138753777,640.097987603797,
63.2458246077949));
#105078=CARTESIAN_POINT('Ctrl Pts',(-31.1249336139912,639.486977930442,
62.9713637144933));
#105079=CARTESIAN_POINT('Ctrl Pts',(-31.0154542096272,640.079925697966,
62.9501636895933));
#105080=CARTESIAN_POINT('Ctrl Pts',(-31.6047168885246,640.070170586937,
62.8196221380521));
#105081=CARTESIAN_POINT('Ctrl Pts',(-31.0798069669301,639.470931087843,
62.7834074755949));
#105082=CARTESIAN_POINT('Ctrl Pts',(-30.9684675402991,640.065797566145,
62.7595873868922));
#105083=CARTESIAN_POINT('Ctrl Pts',(-31.5556085077068,640.052979751955,
62.6101912064094));
#105084=CARTESIAN_POINT('Ctrl Pts',(-30.9184187369807,639.414526541786,
62.2291146946095));
#105085=CARTESIAN_POINT('Ctrl Pts',(-30.8006348715585,640.016214778984,
62.1974227483927));
#105086=CARTESIAN_POINT('Ctrl Pts',(-31.379994664234,639.992512479841,61.9925684320935));
#105087=CARTESIAN_POINT('Ctrl Pts',(-30.7764312493032,639.365891441069,
61.8722609501814));
#105088=CARTESIAN_POINT('Ctrl Pts',(-30.6528555145984,639.973496030507,
61.8369829267743));
#105089=CARTESIAN_POINT('Ctrl Pts',(-31.2255061246491,639.940331754255,
61.5949428691868));
#105090=CARTESIAN_POINT('Ctrl Pts',(-30.4202373697957,639.251358448989,
61.1845444688204));
#105091=CARTESIAN_POINT('Ctrl Pts',(-30.2872866136104,639.874270624505,
61.1477102937615));
#105092=CARTESIAN_POINT('Ctrl Pts',(-30.8380612906271,639.817121140284,
60.8286524472484));
#105093=CARTESIAN_POINT('Ctrl Pts',(-30.2110021753699,639.187131253443,
60.8636665662452));
#105094=CARTESIAN_POINT('Ctrl Pts',(-30.0729968186835,639.818885980513,
60.8282389397767));
#105095=CARTESIAN_POINT('Ctrl Pts',(-30.6105133697495,639.747885147849,
60.4711132048704));
#105096=CARTESIAN_POINT('Ctrl Pts',(-29.8531791687691,639.086868693642,
60.4186064777946));
#105097=CARTESIAN_POINT('Ctrl Pts',(-29.7133672861232,639.733791481457,
60.3901096029334));
#105098=CARTESIAN_POINT('Ctrl Pts',(-30.2215132342272,639.639334841987,
59.9752036724944));
#105099=CARTESIAN_POINT('Ctrl Pts',(-29.7264149308112,639.052757750992,
60.2761430493737));
#105100=CARTESIAN_POINT('Ctrl Pts',(-29.5858497865698,639.70481779123,60.2497909596439));
#105101=CARTESIAN_POINT('Ctrl Pts',(-30.0837246437525,639.602328735179,
59.8164633689678));
#105102=CARTESIAN_POINT('Ctrl Pts',(-29.4573261779289,638.984176116224,
60.0032337484715));
#105103=CARTESIAN_POINT('Ctrl Pts',(-29.3167867305768,639.646776340438,
59.9818071084143));
#105104=CARTESIAN_POINT('Ctrl Pts',(-29.7912900142244,639.52771251499,59.5123733782039));
#105105=CARTESIAN_POINT('Ctrl Pts',(-29.3144414166823,638.949599478752,
59.8724601150719));
#105106=CARTESIAN_POINT('Ctrl Pts',(-29.1746256162575,639.617633014463,
59.854007428715));
#105107=CARTESIAN_POINT('Ctrl Pts',(-29.6360356611041,639.489984964564,
59.3666584849922));
#105108=CARTESIAN_POINT('Ctrl Pts',(-28.8713588165294,638.849263193194,
59.5070266266901));
#105109=CARTESIAN_POINT('Ctrl Pts',(-28.7343122010769,639.53279745443,59.4959957724646));
#105110=CARTESIAN_POINT('Ctrl Pts',(-29.1546960250352,639.380077654759,
58.959473158275));
#105111=CARTESIAN_POINT('Ctrl Pts',(-28.5542773646734,638.786167723086,
59.2959879030435));
#105112=CARTESIAN_POINT('Ctrl Pts',(-28.4246322286205,639.480180811518,
59.2928614504489));
#105113=CARTESIAN_POINT('Ctrl Pts',(-28.8103644308171,639.310385750122,
58.724322722433));
#105114=CARTESIAN_POINT('Ctrl Pts',(-27.8755320887359,638.675756812919,
58.9385684071363));
#105115=CARTESIAN_POINT('Ctrl Pts',(-27.7672168563168,639.3865757007,58.9467223246297));
#105116=CARTESIAN_POINT('Ctrl Pts',(-28.0736484273117,639.186570194773,
58.3260670892298));
#105117=CARTESIAN_POINT('Ctrl Pts',(-27.5112853189433,638.62850564541,58.7924168303215));
#105118=CARTESIAN_POINT('Ctrl Pts',(-27.4195305018196,639.346056019806,
58.8059538597408));
#105119=CARTESIAN_POINT('Ctrl Pts',(-27.6784676113671,639.132473886899,
58.1632173161809));
#105120=CARTESIAN_POINT('Ctrl Pts',(-26.7705302994941,638.561026384799,
58.5795138846031));
#105121=CARTESIAN_POINT('Ctrl Pts',(-26.7123185573368,639.283986825685,
58.5954396179378));
#105122=CARTESIAN_POINT('Ctrl Pts',(-26.8752220660644,639.051904635401,
57.9259895427364));
#105123=CARTESIAN_POINT('Ctrl Pts',(-26.390262231729,638.540012680231,58.5102517531126));
#105124=CARTESIAN_POINT('Ctrl Pts',(-26.3531632859189,639.262102841207,
58.5245086708497));
#105125=CARTESIAN_POINT('Ctrl Pts',(-26.4630739366364,639.024566786374,
57.8488139449765));
#105126=CARTESIAN_POINT('Ctrl Pts',(-25.6094285011568,638.527157113703,
58.4469171473938));
#105127=CARTESIAN_POINT('Ctrl Pts',(-25.6080269458141,639.238702551721,
58.4501065549983));
#105128=CARTESIAN_POINT('Ctrl Pts',(-25.6172217634613,638.999604848902,
57.778242915881));
#105129=CARTESIAN_POINT('Ctrl Pts',(-25.2189809711016,638.535609798989,
58.453979164517));
#105130=CARTESIAN_POINT('Ctrl Pts',(-25.2361374307006,639.23752462347,58.4476660614292));
#105131=CARTESIAN_POINT('Ctrl Pts',(-25.194480338516,639.002435896301,57.7861115876274));
#105132=CARTESIAN_POINT('Ctrl Pts',(-24.6409354929901,638.568745456371,
58.5186871133032));
#105133=CARTESIAN_POINT('Ctrl Pts',(-24.6736512904528,639.251920802327,
58.4966619148348));
#105134=CARTESIAN_POINT('Ctrl Pts',(-24.5689264138619,639.027847597861,
57.8582122899254));
#105135=CARTESIAN_POINT('Ctrl Pts',(-24.4490972732004,638.583191576161,
58.5493117143284));
#105136=CARTESIAN_POINT('Ctrl Pts',(-24.4873728312289,639.259283169087,
58.5213924422961));
#105137=CARTESIAN_POINT('Ctrl Pts',(-24.3613718882865,639.039830475442,
57.8923357215899));
#105138=CARTESIAN_POINT('Ctrl Pts',(-24.0671081959017,638.618540338843,
58.6287302863804));
#105139=CARTESIAN_POINT('Ctrl Pts',(-24.1139136994163,639.279335311201,
58.5889529536862));
#105140=CARTESIAN_POINT('Ctrl Pts',(-23.9481847707517,639.070465560091,
57.9808278590847));
#105141=CARTESIAN_POINT('Ctrl Pts',(-23.8768636638465,638.639494936042,
58.6776732346629));
#105142=CARTESIAN_POINT('Ctrl Pts',(-23.9270215097293,639.291978429298,
58.6316256560464));
#105143=CARTESIAN_POINT('Ctrl Pts',(-23.7424514950666,639.089169818811,
58.0353625563298));
#105144=CARTESIAN_POINT('Ctrl Pts',(-23.3201749292324,638.709821703261,
58.8484494113552));
#105145=CARTESIAN_POINT('Ctrl Pts',(-23.3806749026967,639.336411072855,
58.7835372517324));
#105146=CARTESIAN_POINT('Ctrl Pts',(-23.1405719163352,639.15317327971,58.2256500255681));
#105147=CARTESIAN_POINT('Ctrl Pts',(-22.9636204205607,638.766962613931,
58.9946750187081));
#105148=CARTESIAN_POINT('Ctrl Pts',(-23.0243053306422,639.375032265077,
58.9173052658177));
#105149=CARTESIAN_POINT('Ctrl Pts',(-22.7552500131854,639.206615373746,
58.3885820845647));
#105150=CARTESIAN_POINT('Ctrl Pts',(-22.27848089945,638.895420482319,59.3507109235853));
#105151=CARTESIAN_POINT('Ctrl Pts',(-22.3317399785605,639.467210290523,
59.2554960516949));
#105152=CARTESIAN_POINT('Ctrl Pts',(-22.0151053084073,639.328507485308,
58.7852957947004));
#105153=CARTESIAN_POINT('Ctrl Pts',(-21.9500159216726,638.966926375171,
59.5614980956268));
#105154=CARTESIAN_POINT('Ctrl Pts',(-21.995648509837,639.520426082359,59.4584719479871));
#105155=CARTESIAN_POINT('Ctrl Pts',(-21.6604152666523,639.397153710713,
59.0201658778045));
#105156=CARTESIAN_POINT('Ctrl Pts',(-21.3460486897185,639.111793677402,
60.0320961056729));
#105157=CARTESIAN_POINT('Ctrl Pts',(-21.374045693413,639.631792692931,59.9216812301887));
#105158=CARTESIAN_POINT('Ctrl Pts',(-21.0084223762403,639.537151410169,
59.5445310201806));
#105159=CARTESIAN_POINT('Ctrl Pts',(-21.0669931238233,639.185808726979,
60.2934777106252));
#105160=CARTESIAN_POINT('Ctrl Pts',(-21.0834671017477,639.690247737726,
60.1816491447995));
#105161=CARTESIAN_POINT('Ctrl Pts',(-20.7072807213335,639.609122100779,
59.8357762715668));
#105162=CARTESIAN_POINT('Ctrl Pts',(-20.6843161289542,639.293828358263,
60.7275832942433));
#105163=CARTESIAN_POINT('Ctrl Pts',(-20.6816094426164,639.777663387302,
60.6221327845261));
#105164=CARTESIAN_POINT('Ctrl Pts',(-20.2944117951707,639.714527579313,
60.3194799830296));
#105165=CARTESIAN_POINT('Ctrl Pts',(-20.5629709963199,639.329293550566,
60.879349817338));
#105166=CARTESIAN_POINT('Ctrl Pts',(-20.554558284157,639.806446454198,60.7757280451264));
#105167=CARTESIAN_POINT('Ctrl Pts',(-20.1635106966246,639.749199037125,
60.4885863707933));
#105168=CARTESIAN_POINT('Ctrl Pts',(-20.3379823034572,639.396756759074,
61.1906817235449));
#105169=CARTESIAN_POINT('Ctrl Pts',(-20.3188450962156,639.861528013512,
61.0920285161997));
#105170=CARTESIAN_POINT('Ctrl Pts',(-19.9208290490855,639.815240108573,
60.8354890916476));
#105171=CARTESIAN_POINT('Ctrl Pts',(-20.2336008003601,639.428961041436,
61.3510394361652));
#105172=CARTESIAN_POINT('Ctrl Pts',(-20.2090499310174,639.888053434363,
61.2556019061011));
#105173=CARTESIAN_POINT('Ctrl Pts',(-19.8082522970898,639.846810887964,
61.0141682831509));
#105174=CARTESIAN_POINT('Ctrl Pts',(-19.9449136033705,639.519814097585,
61.8464125125788));
#105175=CARTESIAN_POINT('Ctrl Pts',(-19.9070847959734,639.962771595516,
61.7594811413053));
#105176=CARTESIAN_POINT('Ctrl Pts',(-19.4969257393655,639.935963708212,
61.5661395895971));
#105177=CARTESIAN_POINT('Ctrl Pts',(-19.7847575698374,639.57275723913,62.1955854246443));
#105178=CARTESIAN_POINT('Ctrl Pts',(-19.7367196925424,640.007397463489,
62.1194969013774));
#105179=CARTESIAN_POINT('Ctrl Pts',(-19.3242457747715,639.988037778914,
61.9552110306678));
#105180=CARTESIAN_POINT('Ctrl Pts',(-19.6604708015409,639.614602859825,
62.5660174884535));
#105181=CARTESIAN_POINT('Ctrl Pts',(-19.6043565557346,640.042864698584,
62.5045799077997));
#105182=CARTESIAN_POINT('Ctrl Pts',(-19.1902534503917,640.029230307342,
62.3679625261942));
#105183=CARTESIAN_POINT('Origin',(-48.,620.675373764374,64.2994740882088));
#105184=CARTESIAN_POINT('Origin',(28.,620.675373764374,64.2994740882088));
#105185=CARTESIAN_POINT('Ctrl Pts',(1.86306288877798,606.534169754924,79.840079036097));
#105186=CARTESIAN_POINT('Ctrl Pts',(2.14021144979533,606.496771580384,79.8060484936875));
#105187=CARTESIAN_POINT('Ctrl Pts',(2.4133761460843,606.451830720321,79.7649147909193));
#105188=CARTESIAN_POINT('Ctrl Pts',(2.68283184001625,606.400050317104,79.7169704303203));
#105189=CARTESIAN_POINT('Ctrl Pts',(2.97414735927081,606.344069184063,79.6651365421608));
#105190=CARTESIAN_POINT('Ctrl Pts',(3.26112767369667,606.280094095968,79.6053412098497));
#105191=CARTESIAN_POINT('Ctrl Pts',(3.54412011470249,606.209064457015,79.5379106224147));
#105192=CARTESIAN_POINT('Ctrl Pts',(3.88187814635567,606.124288938076,79.4574306548075));
#105193=CARTESIAN_POINT('Ctrl Pts',(4.21395546218491,606.029464281995,79.3660724895544));
#105194=CARTESIAN_POINT('Ctrl Pts',(4.54094258490408,605.926255970468,79.2643522128276));
#105195=CARTESIAN_POINT('Ctrl Pts',(4.66022073585215,605.888607709402,79.2272467561326));
#105196=CARTESIAN_POINT('Ctrl Pts',(4.7788215654658,605.84984443673,79.1887623167325));
#105197=CARTESIAN_POINT('Ctrl Pts',(4.89677373712177,605.810048547591,79.1489238821405));
#105198=CARTESIAN_POINT('Ctrl Pts',(5.16043615150262,605.721091472317,79.0598717035989));
#105199=CARTESIAN_POINT('Ctrl Pts',(5.42147464016636,605.626588819934,78.9636635925401));
#105200=CARTESIAN_POINT('Ctrl Pts',(5.67881724163154,605.527777854217,78.8608748149868));
#105201=CARTESIAN_POINT('Ctrl Pts',(5.89134528491515,605.446174182384,78.7759860416529));
#105202=CARTESIAN_POINT('Ctrl Pts',(6.10135258954282,605.361632372566,78.6866091801219));
#105203=CARTESIAN_POINT('Ctrl Pts',(6.30823535587315,605.274837711021,78.593093022985));
#105204=CARTESIAN_POINT('Ctrl Pts',(6.6081803457824,605.149000144447,78.4575104256217));
#105205=CARTESIAN_POINT('Ctrl Pts',(6.90074477299936,605.018887494591,78.3137274985418));
#105206=CARTESIAN_POINT('Ctrl Pts',(7.18661418705821,604.885610576882,78.1619208948199));
#105207=CARTESIAN_POINT('Ctrl Pts',(7.33667046294114,604.81565192811,78.0822357921518));
#105208=CARTESIAN_POINT('Ctrl Pts',(7.48488204463535,604.744821534827,78.0003406744257));
#105209=CARTESIAN_POINT('Ctrl Pts',(7.63134808340531,604.673280035404,77.9162670025649));
#105210=CARTESIAN_POINT('Ctrl Pts',(7.91723728695995,604.533637136183,77.7521623726448));
#105211=CARTESIAN_POINT('Ctrl Pts',(8.19655198248917,604.391360677278,77.5798506235828));
#105212=CARTESIAN_POINT('Ctrl Pts',(8.46960770404473,604.247250255253,77.3991233565012));
#105213=CARTESIAN_POINT('Ctrl Pts',(8.73947522321079,604.104822468513,77.220506263495));
#105214=CARTESIAN_POINT('Ctrl Pts',(9.00322907485539,603.960603546486,77.0336684769913));
#105215=CARTESIAN_POINT('Ctrl Pts',(9.26117386903771,603.815407551738,76.8384370553757));
#105216=CARTESIAN_POINT('Ctrl Pts',(9.51911866322004,603.67021155699,76.6432056337602));
#105217=CARTESIAN_POINT('Ctrl Pts',(9.7712543999401,603.524038705004,76.4395799971655));
#105218=CARTESIAN_POINT('Ctrl Pts',(10.0178856892571,603.377742099661,76.2274241122124));
#105219=CARTESIAN_POINT('Ctrl Pts',(10.203587578906,603.267587560322,76.0676805985445));
#105220=CARTESIAN_POINT('Ctrl Pts',(10.3856411221024,603.157580684183,75.9034085015199));
#105221=CARTESIAN_POINT('Ctrl Pts',(10.5636740062097,603.048302838395,75.7349637390157));
#105222=CARTESIAN_POINT('Ctrl Pts',(10.7417068903169,602.939024992607,75.5665189765115));
#105223=CARTESIAN_POINT('Ctrl Pts',(10.9157191153351,602.830476606266,75.3939015342058));
#105224=CARTESIAN_POINT('Ctrl Pts',(11.0853383686276,602.723200323969,75.2175106218));
#105225=CARTESIAN_POINT('Ctrl Pts',(11.2982866914204,602.588520422088,74.9960608263106));
#105226=CARTESIAN_POINT('Ctrl Pts',(11.5047763502688,602.455585063299,74.7682551816903));
#105227=CARTESIAN_POINT('Ctrl Pts',(11.7048608093102,602.324863862536,74.5338690056311));
#105228=CARTESIAN_POINT('Ctrl Pts',(11.8235220073649,602.247338929476,74.39486498407));
#105229=CARTESIAN_POINT('Ctrl Pts',(11.9399304013359,602.170593652194,74.2535467954905));
#105230=CARTESIAN_POINT('Ctrl Pts',(12.0540971431182,602.094734098787,74.1098707468977));
#105231=CARTESIAN_POINT('Ctrl Pts',(12.2247846330108,601.981318610587,73.8950647209996));
#105232=CARTESIAN_POINT('Ctrl Pts',(12.3904618758627,601.869880815692,73.6749899685042));
#105233=CARTESIAN_POINT('Ctrl Pts',(12.5510400004671,601.760743347098,73.4493816921722));
#105234=CARTESIAN_POINT('Ctrl Pts',(12.6789711937227,601.673794476444,73.2696415434402));
#105235=CARTESIAN_POINT('Ctrl Pts',(12.8036658898818,601.588306560693,73.0863892070135));
#105236=CARTESIAN_POINT('Ctrl Pts',(12.9250791491289,601.504466168008,72.899494722766));
#105237=CARTESIAN_POINT('Ctrl Pts',(13.0388387824065,601.425910890068,72.724381657509));
#105238=CARTESIAN_POINT('Ctrl Pts',(13.1495772962539,601.348869677579,72.5462085445997));
#105239=CARTESIAN_POINT('Ctrl Pts',(13.2569702277637,601.273706826003,72.3654131529255));
#105240=CARTESIAN_POINT('Ctrl Pts',(13.3632468260221,601.19932528088,72.1864971019544));
#105241=CARTESIAN_POINT('Ctrl Pts',(13.466247034086,601.126783414445,72.0050131874339));
#105242=CARTESIAN_POINT('Ctrl Pts',(13.565656402463,601.056390585734,71.8214121376375));
#105243=CARTESIAN_POINT('Ctrl Pts',(13.6075769852419,601.026706176194,71.7439882174182));
#105244=CARTESIAN_POINT('Ctrl Pts',(13.6488590164011,600.997403375317,71.6661881202247));
#105245=CARTESIAN_POINT('Ctrl Pts',(13.6894789155558,600.96850291657,71.5880469506538));
#105246=CARTESIAN_POINT('Ctrl Pts',(13.8286010750813,600.869519553345,71.320415359124));
#105247=CARTESIAN_POINT('Ctrl Pts',(13.9605180227581,600.774973302884,71.0480331379636));
#105248=CARTESIAN_POINT('Ctrl Pts',(14.0849573496678,600.685214684286,70.7707639855925));
#105249=CARTESIAN_POINT('Ctrl Pts',(14.2077624538311,600.596634837542,70.4971361222487));
#105250=CARTESIAN_POINT('Ctrl Pts',(14.3232850500889,600.512717686243,70.21874852948));
#105251=CARTESIAN_POINT('Ctrl Pts',(14.431263321578,600.433847155292,69.9354880623801));
#105252=CARTESIAN_POINT('Ctrl Pts',(14.53713756658,600.356513467671,69.6577471087649));
#105253=CARTESIAN_POINT('Ctrl Pts',(14.6357586344046,600.284031700042,69.3753210477071));
#105254=CARTESIAN_POINT('Ctrl Pts',(14.7268797169107,600.216808888376,69.0881248582872));
#105255=CARTESIAN_POINT('Ctrl Pts',(14.7658178500568,600.188083035706,68.9653993247979));
#105256=CARTESIAN_POINT('Ctrl Pts',(14.8033864488703,600.160318058013,68.8418030398932));
#105257=CARTESIAN_POINT('Ctrl Pts',(14.8395662545944,600.133548262682,68.7173308130521));
#105258=CARTESIAN_POINT('Ctrl Pts',(14.9306676469207,600.066141443377,68.4039075388196));
#105259=CARTESIAN_POINT('Ctrl Pts',(15.0120041807907,600.0057505978,68.0882301956629));
#105260=CARTESIAN_POINT('Ctrl Pts',(15.0834994605404,599.952495015445,67.7702592069415));
#105261=CARTESIAN_POINT('Ctrl Pts',(15.1544872250668,599.899617472296,67.4545453618789));
#105262=CARTESIAN_POINT('Ctrl Pts',(15.2157729575042,599.853774233935,67.1365698743685));
#105263=CARTESIAN_POINT('Ctrl Pts',(15.26728187757,599.815132996122,66.8162990868483));
#105264=CARTESIAN_POINT('Ctrl Pts',(15.3181640307096,599.776961949682,66.4999253939824));
#105265=CARTESIAN_POINT('Ctrl Pts',(15.3595058548215,599.74581874709,66.1813114971069));
#105266=CARTESIAN_POINT('Ctrl Pts',(15.3912352663485,599.721914626943,65.8604363424684));
#105267=CARTESIAN_POINT('Ctrl Pts',(15.3996803499289,599.715552318824,65.7750323790987));
#105268=CARTESIAN_POINT('Ctrl Pts',(15.4074444818654,599.709703106282,65.6894683089235));
#105269=CARTESIAN_POINT('Ctrl Pts',(15.414526303025,599.704371567147,65.6037439326523));
#105270=CARTESIAN_POINT('Ctrl Pts',(15.4364643525561,599.687855537305,65.3381871542066));
#105271=CARTESIAN_POINT('Ctrl Pts',(15.4517893452765,599.676303804616,65.0710724250625));
#105272=CARTESIAN_POINT('Ctrl Pts',(15.4603232031337,599.669870597506,64.8023554757184));
#105273=CARTESIAN_POINT('Ctrl Pts',(15.4648538948456,599.666455157663,64.6596915509595));
#105274=CARTESIAN_POINT('Ctrl Pts',(15.4674510190573,599.664486012478,64.5165142301009));
#105275=CARTESIAN_POINT('Ctrl Pts',(15.4681203454456,599.663982203095,64.3734851808145));
#105276=CARTESIAN_POINT('Ctrl Pts',(15.4687117396317,599.663537054144,64.2471095445311));
#105277=CARTESIAN_POINT('Ctrl Pts',(15.4677981227552,599.664235122814,64.1208497755974));
#105278=CARTESIAN_POINT('Ctrl Pts',(15.465383474685,599.66605565863,63.9951622171671));
#105279=CARTESIAN_POINT('Ctrl Pts',(15.459452342433,599.670527465029,63.6864341914551));
#105280=CARTESIAN_POINT('Ctrl Pts',(15.4445576266959,599.681772011648,63.3797508309674));
#105281=CARTESIAN_POINT('Ctrl Pts',(15.4209342345178,599.699557577838,63.0750606401227));
#105282=CARTESIAN_POINT('Ctrl Pts',(15.4035532438902,599.712643368266,62.8508838025442));
#105283=CARTESIAN_POINT('Ctrl Pts',(15.381447132351,599.72927106591,62.6277854531142));
#105284=CARTESIAN_POINT('Ctrl Pts',(15.3547094604652,599.749365484678,62.4057395605387));
#105285=CARTESIAN_POINT('Ctrl Pts',(15.3159115020454,599.778523686152,62.0835377119923));
#105286=CARTESIAN_POINT('Ctrl Pts',(15.2673586125687,599.814979310381,61.7635549646558));
#105287=CARTESIAN_POINT('Ctrl Pts',(15.2091365971295,599.858544359385,61.4457630820266));
#105288=CARTESIAN_POINT('Ctrl Pts',(15.1727005295032,599.885807913552,61.2468849353461));
#105289=CARTESIAN_POINT('Ctrl Pts',(15.1324776324204,599.915856841564,61.0488645460237));
#105290=CARTESIAN_POINT('Ctrl Pts',(15.0884889362004,599.948655262748,60.8516931877506));
#105291=CARTESIAN_POINT('Ctrl Pts',(15.0441618970613,599.981705955868,60.6530052686642));
#105292=CARTESIAN_POINT('Ctrl Pts',(14.99587961035,600.017618426599,60.4547901096127));
#105293=CARTESIAN_POINT('Ctrl Pts',(14.9437846854305,600.056282502727,60.2575526976988));
#105294=CARTESIAN_POINT('Ctrl Pts',(14.891515090916,600.095076216022,60.0596539664928));
#105295=CARTESIAN_POINT('Ctrl Pts',(14.8354072484661,600.136639957072,59.8627397875043));
#105296=CARTESIAN_POINT('Ctrl Pts',(14.7756052067288,600.180811300144,59.6673080308479));
#105297=CARTESIAN_POINT('Ctrl Pts',(14.7413494348752,600.206113503994,59.5553609221124));
#105298=CARTESIAN_POINT('Ctrl Pts',(14.7058815145681,600.232270383962,59.4438999846864));
#105299=CARTESIAN_POINT('Ctrl Pts',(14.6692285204308,600.259244049245,59.3330165540887));
#105300=CARTESIAN_POINT('Ctrl Pts',(14.5803938226727,600.324619265082,59.0642719051074));
#105301=CARTESIAN_POINT('Ctrl Pts',(14.4851858741709,600.394481384538,58.8001708828506));
#105302=CARTESIAN_POINT('Ctrl Pts',(14.3837715170904,600.468473187238,58.5405486633614));
#105303=CARTESIAN_POINT('Ctrl Pts',(14.2810607054499,600.54341088175,58.2776075014656));
#105304=CARTESIAN_POINT('Ctrl Pts',(14.1719837887536,600.622584561164,58.0192600662296));
#105305=CARTESIAN_POINT('Ctrl Pts',(14.0567140899125,600.705674919426,57.7653191294322));
#105306=CARTESIAN_POINT('Ctrl Pts',(13.9392204614059,600.79036836258,57.5064788410421));
#105307=CARTESIAN_POINT('Ctrl Pts',(13.8152927875511,600.879131076811,57.2522164161193));
#105308=CARTESIAN_POINT('Ctrl Pts',(13.6851146179499,600.971678122617,57.0023218326902));
#105309=CARTESIAN_POINT('Ctrl Pts',(13.6023354929409,601.0305279551,56.8434161188971));
#105310=CARTESIAN_POINT('Ctrl Pts',(13.5170289340367,601.09090908028,56.6862763549344));
#105311=CARTESIAN_POINT('Ctrl Pts',(13.4292421368317,601.152759033305,56.5308469864961));
#105312=CARTESIAN_POINT('Ctrl Pts',(13.2697747250477,601.265111371492,56.2485047677433));
#105313=CARTESIAN_POINT('Ctrl Pts',(13.101898661713,601.382367267854,55.9716775249368));
#105314=CARTESIAN_POINT('Ctrl Pts',(12.9258526145729,601.503935650737,55.7006361645003));
#105315=CARTESIAN_POINT('Ctrl Pts',(12.8286620255447,601.571050493311,55.5510010553925));
#105316=CARTESIAN_POINT('Ctrl Pts',(12.728981334913,601.639479369392,55.4031285395231));
#105317=CARTESIAN_POINT('Ctrl Pts',(12.6268507021078,601.709120557677,55.257057802576));
#105318=CARTESIAN_POINT('Ctrl Pts',(12.469345250969,601.81652091815,55.0317880995584));
#105319=CARTESIAN_POINT('Ctrl Pts',(12.3071295901563,601.926054873237,54.8123661471076));
#105320=CARTESIAN_POINT('Ctrl Pts',(12.140284433182,602.037364111905,54.5985128380187));
#105321=CARTESIAN_POINT('Ctrl Pts',(12.0029789361845,602.128966233374,54.4225219047395));
#105322=CARTESIAN_POINT('Ctrl Pts',(11.8625381156151,602.221771720644,54.2503020731634));
#105323=CARTESIAN_POINT('Ctrl Pts',(11.7190069566274,602.315607074176,54.0816944827994));
#105324=CARTESIAN_POINT('Ctrl Pts',(11.5129986901234,602.450287645658,53.8396943648089));
#105325=CARTESIAN_POINT('Ctrl Pts',(11.300702240442,602.587133145572,53.6050605705711));
#105326=CARTESIAN_POINT('Ctrl Pts',(11.0819551471639,602.725518054895,53.3776274956182));
#105327=CARTESIAN_POINT('Ctrl Pts',(10.8537269626199,602.869900940856,53.140336855437));
#105328=CARTESIAN_POINT('Ctrl Pts',(10.6184768396464,603.015959261177,52.9108844662551));
#105329=CARTESIAN_POINT('Ctrl Pts',(10.3760202645829,603.163032449609,52.6890496920733));
#105330=CARTESIAN_POINT('Ctrl Pts',(10.1335636895193,603.310105638041,52.4672149178915));
#105331=CARTESIAN_POINT('Ctrl Pts',(9.88390066236575,603.458193761935,52.2529973474516));
#105332=CARTESIAN_POINT('Ctrl Pts',(9.62684666946167,603.60668640386,52.0461494466168));
#105333=CARTESIAN_POINT('Ctrl Pts',(9.46346234489243,603.701068793063,51.914676271722));
#105334=CARTESIAN_POINT('Ctrl Pts',(9.29686479132284,603.79566622951,51.7861174759939));
#105335=CARTESIAN_POINT('Ctrl Pts',(9.1275807697144,603.889945916815,51.6609035615386));
#105336=CARTESIAN_POINT('Ctrl Pts',(8.95353419621665,603.98687802163,51.5321669415191));
#105337=CARTESIAN_POINT('Ctrl Pts',(8.77664786886439,604.083473998631,51.4069661381686));
#105338=CARTESIAN_POINT('Ctrl Pts',(8.59749427002016,604.179117051247,51.28572876114));
#105339=CARTESIAN_POINT('Ctrl Pts',(8.54536693177707,604.206945784727,51.2504529877208));
#105340=CARTESIAN_POINT('Ctrl Pts',(8.49304764555114,604.234693619584,51.2155125022191));
#105341=CARTESIAN_POINT('Ctrl Pts',(8.44055051338909,604.2623448376,51.1809172151338));
#105342=CARTESIAN_POINT('Ctrl Pts',(8.16409659561211,604.407958268986,50.9987357843119));
#105343=CARTESIAN_POINT('Ctrl Pts',(7.88203506759103,604.551352521409,50.8255502039239));
#105344=CARTESIAN_POINT('Ctrl Pts',(7.59396676189712,604.691519497847,50.661275681908));
#105345=CARTESIAN_POINT('Ctrl Pts',(7.45646787271816,604.758423086957,50.5828652360132));
#105346=CARTESIAN_POINT('Ctrl Pts',(7.31760047037148,604.824591914183,50.5064843721725));
#105347=CARTESIAN_POINT('Ctrl Pts',(7.1773211472115,604.889919348387,50.4321209931153));
#105348=CARTESIAN_POINT('Ctrl Pts',(6.8801828412943,605.028295287847,50.2746052026366));
#105349=CARTESIAN_POINT('Ctrl Pts',(6.57671769730194,605.162903406008,50.1261374141598));
#105350=CARTESIAN_POINT('Ctrl Pts',(6.26623698972573,605.292427418651,49.9869266312457));
#105351=CARTESIAN_POINT('Ctrl Pts',(6.12304923299768,605.352161412939,49.9227252840077));
#105352=CARTESIAN_POINT('Ctrl Pts',(5.97836935164866,605.410814201732,49.8604919927748));
#105353=CARTESIAN_POINT('Ctrl Pts',(5.83212979029488,605.468257827998,49.8002438368876));
#105354=CARTESIAN_POINT('Ctrl Pts',(5.60046097050222,605.559258491419,49.7048003123046));
#105355=CARTESIAN_POINT('Ctrl Pts',(5.36486309244537,605.647207349457,49.6143579168885));
#105356=CARTESIAN_POINT('Ctrl Pts',(5.12496004470658,605.731474628392,49.5291006468632));
#105357=CARTESIAN_POINT('Ctrl Pts',(4.92336015567768,605.802287709935,49.4574556371894));
#105358=CARTESIAN_POINT('Ctrl Pts',(4.71807804538495,605.870685385895,49.3892915169508));
#105359=CARTESIAN_POINT('Ctrl Pts',(4.51111271505955,605.935569889985,49.3254220404912));
#105360=CARTESIAN_POINT('Ctrl Pts',(4.47179014433253,605.947897681781,49.3132870998157));
#105361=CARTESIAN_POINT('Ctrl Pts',(4.4324068119646,605.960098558052,49.3013070706584));
#105362=CARTESIAN_POINT('Ctrl Pts',(4.39297642822443,605.972164865804,49.2894873770812));
#105363=CARTESIAN_POINT('Ctrl Pts',(4.12486075126134,606.054212413018,49.209116737885));
#105364=CARTESIAN_POINT('Ctrl Pts',(3.8544403326532,606.130209721402,49.1359860390462));
#105365=CARTESIAN_POINT('Ctrl Pts',(3.58156371892322,606.199404405331,49.0702139584696));
#105366=CARTESIAN_POINT('Ctrl Pts',(3.32312890924601,606.264937008978,49.0079228192858));
#105367=CARTESIAN_POINT('Ctrl Pts',(3.06249100950961,606.324367834277,48.9522313546321));
#105368=CARTESIAN_POINT('Ctrl Pts',(2.7995213627417,606.377094055612,48.9032651277793));
#105369=CARTESIAN_POINT('Ctrl Pts',(2.55448969638108,606.426223656816,48.8576390400973));
#105370=CARTESIAN_POINT('Ctrl Pts',(2.30743354478633,606.469532170608,48.8178516695855));
#105371=CARTESIAN_POINT('Ctrl Pts',(2.0582488241673,606.50656489739,48.7840331252817));
#105372=CARTESIAN_POINT('Ctrl Pts',(1.81685586891249,606.542439646599,48.7512720541711));
#105373=CARTESIAN_POINT('Ctrl Pts',(1.57346538001183,606.572424798898,48.7241119998907));
#105374=CARTESIAN_POINT('Ctrl Pts',(1.32798273535137,606.596140220963,48.7027040439557));
#105375=CARTESIAN_POINT('Ctrl Pts',(1.09319241853544,606.618822685819,48.6822285404295));
#105376=CARTESIAN_POINT('Ctrl Pts',(0.855738997648291,606.635677081802,
48.6670981287456));
#105377=CARTESIAN_POINT('Ctrl Pts',(0.616984794800867,606.646416089399,
48.6574665592193));
#105378=CARTESIAN_POINT('Ctrl Pts',(0.386532831296134,606.65678166771,48.6481699098514));
#105379=CARTESIAN_POINT('Ctrl Pts',(0.154868977572705,606.661449696049,
48.6439961961589));
#105380=CARTESIAN_POINT('Ctrl Pts',(-0.0767816764458722,606.66019457572,
48.6451198922309));
#105381=CARTESIAN_POINT('Ctrl Pts',(-0.145864683309471,606.659820272929,
48.6454550015954));
#105382=CARTESIAN_POINT('Ctrl Pts',(-0.214946516250035,606.658919423718,
48.6462614978511));
#105383=CARTESIAN_POINT('Ctrl Pts',(-0.283994682921353,606.65748665381,
48.6475446883329));
#105384=CARTESIAN_POINT('Ctrl Pts',(-0.520075952304776,606.652587897551,
48.6519320204289));
#105385=CARTESIAN_POINT('Ctrl Pts',(-0.755839055281912,606.641499149446,
48.6618612476739));
#105386=CARTESIAN_POINT('Ctrl Pts',(-0.990327191987344,606.624559493982,
48.6770968260201));
#105387=CARTESIAN_POINT('Ctrl Pts',(-1.23740315666562,606.606710481345,
48.6931502830105));
#105388=CARTESIAN_POINT('Ctrl Pts',(-1.48306359503986,606.582365636056,
48.7150953295273));
#105389=CARTESIAN_POINT('Ctrl Pts',(-1.72618919815674,606.551960679876,
48.7426988494953));
#105390=CARTESIAN_POINT('Ctrl Pts',(-1.78055170454703,606.545162179005,
48.7488709535905));
#105391=CARTESIAN_POINT('Ctrl Pts',(-1.83478747864495,606.538060838178,
48.7553261113013));
#105392=CARTESIAN_POINT('Ctrl Pts',(-1.8888840075986,606.53066176659,48.7620619651123));
#105393=CARTESIAN_POINT('Ctrl Pts',(-0.252645464510396,603.935273498433,
76.9980210944396));
#105394=CARTESIAN_POINT('Ctrl Pts',(-1.11302381605652,603.921973867958,
76.980488604498));
#105395=CARTESIAN_POINT('Ctrl Pts',(-1.94758251680077,603.841082066435,
76.8749778358584));
#105396=CARTESIAN_POINT('Ctrl Pts',(-3.16572559796507,603.638181713665,
76.5970874596841));
#105397=CARTESIAN_POINT('Ctrl Pts',(-3.56612249316459,603.556968056736,
76.4843247054231));
#105398=CARTESIAN_POINT('Ctrl Pts',(-4.35605342916383,603.370767324989,
76.2184083741727));
#105399=CARTESIAN_POINT('Ctrl Pts',(-4.74439125163809,603.265908061918,
76.0653418396745));
#105400=CARTESIAN_POINT('Ctrl Pts',(-5.86615041872897,602.93028205798,75.5582538330123));
#105401=CARTESIAN_POINT('Ctrl Pts',(-6.56690401319744,602.676475086324,
75.153793775975));
#105402=CARTESIAN_POINT('Ctrl Pts',(-7.55642794248227,602.275508918443,
74.4484723523538));
#105403=CARTESIAN_POINT('Ctrl Pts',(-7.87639888507424,602.138112496026,
74.1960774136137));
#105404=CARTESIAN_POINT('Ctrl Pts',(-8.48513868812207,601.864970166375,
73.6665189366011));
#105405=CARTESIAN_POINT('Ctrl Pts',(-8.77540631388641,601.728639986729,
73.3883947993268));
#105406=CARTESIAN_POINT('Ctrl Pts',(-9.32889245043522,601.459703714202,
72.8050737176796));
#105407=CARTESIAN_POINT('Ctrl Pts',(-9.59210827130408,601.327088572554,
72.4998783443379));
#105408=CARTESIAN_POINT('Ctrl Pts',(-10.0915350771624,601.068618464298,
71.8610821467425));
#105409=CARTESIAN_POINT('Ctrl Pts',(-10.3287739497107,600.94218925709,71.525776856965));
#105410=CARTESIAN_POINT('Ctrl Pts',(-10.9894725080146,600.582618362532,
70.4882632613146));
#105411=CARTESIAN_POINT('Ctrl Pts',(-11.3625914305347,600.369242850061,
69.7564109606946));
#105412=CARTESIAN_POINT('Ctrl Pts',(-11.818404938002,600.103341108961,68.5929331071031));
#105413=CARTESIAN_POINT('Ctrl Pts',(-11.9534576443998,600.023405036002,
68.1916750120165));
#105414=CARTESIAN_POINT('Ctrl Pts',(-12.182174157639,599.886968972313,67.3809131335881));
#105415=CARTESIAN_POINT('Ctrl Pts',(-12.276307508626,599.830205075246,66.9709644805429));
#105416=CARTESIAN_POINT('Ctrl Pts',(-12.4242394369779,599.740627853341,
66.1418454500847));
#105417=CARTESIAN_POINT('Ctrl Pts',(-12.4780399075043,599.707811059001,
65.7226757432849));
#105418=CARTESIAN_POINT('Ctrl Pts',(-12.5441585218638,599.667441869139,
64.8747881241364));
#105419=CARTESIAN_POINT('Ctrl Pts',(-12.5562467120334,599.660031095258,
64.4432644779558));
#105420=CARTESIAN_POINT('Ctrl Pts',(-12.5282315834883,599.677167021141,
63.1661747786782));
#105421=CARTESIAN_POINT('Ctrl Pts',(-12.4261421803805,599.739908403138,
62.3315318096105));
#105422=CARTESIAN_POINT('Ctrl Pts',(-12.1532157238051,599.904257995604,
61.1033176255798));
#105423=CARTESIAN_POINT('Ctrl Pts',(-12.0418922330986,599.970921904931,
60.6972107540752));
#105424=CARTESIAN_POINT('Ctrl Pts',(-11.7789498235242,600.126430608746,
59.8958888312612));
#105425=CARTESIAN_POINT('Ctrl Pts',(-11.6297082784345,600.213861256789,
59.5076325746472));
#105426=CARTESIAN_POINT('Ctrl Pts',(-11.1319937919119,600.50080901643,58.3769969850098));
#105427=CARTESIAN_POINT('Ctrl Pts',(-10.7340829199422,600.724949402545,
57.6684452447755));
#105428=CARTESIAN_POINT('Ctrl Pts',(-10.040023576069,601.095528882733,56.6679468437341));
#105429=CARTESIAN_POINT('Ctrl Pts',(-9.79091798691913,601.225505664081,
56.3433436698442));
#105430=CARTESIAN_POINT('Ctrl Pts',(-9.26667744604236,601.490365329661,
55.7243454178727));
#105431=CARTESIAN_POINT('Ctrl Pts',(-8.99185892776024,601.62513172368,55.4299091303579));
#105432=CARTESIAN_POINT('Ctrl Pts',(-8.1292937094432,602.031691427434,54.5894500217195));
#105433=CARTESIAN_POINT('Ctrl Pts',(-7.5038764230366,602.306079133985,54.0856572853192));
#105434=CARTESIAN_POINT('Ctrl Pts',(-6.14010017594243,602.832368541163,
53.1918099095666));
#105435=CARTESIAN_POINT('Ctrl Pts',(-5.42038031899213,603.076911552827,
52.8139552665562));
#105436=CARTESIAN_POINT('Ctrl Pts',(-4.27629107737484,603.390777156775,
52.3511891253608));
#105437=CARTESIAN_POINT('Ctrl Pts',(-3.88308899204296,603.486721140176,
52.2141438459509));
#105438=CARTESIAN_POINT('Ctrl Pts',(-3.07656099875632,603.654779445314,
51.9785830844804));
#105439=CARTESIAN_POINT('Ctrl Pts',(-2.66897700762064,603.725715944193,
51.8816585325753));
#105440=CARTESIAN_POINT('Ctrl Pts',(-1.84491113503772,603.838478649151,
51.7291914233704));
#105441=CARTESIAN_POINT('Ctrl Pts',(-1.42842899531872,603.880302055858,
51.67364863131));
#105442=CARTESIAN_POINT('Ctrl Pts',(-0.586133086793797,603.932122442854,
51.6050092571627));
#105443=CARTESIAN_POINT('Ctrl Pts',(-0.159088542674411,603.942089849916,
51.5919408760206));
#105444=CARTESIAN_POINT('Ctrl Pts',(0.270210553101167,603.934992543017,
51.6012974652903));
#105445=CARTESIAN_POINT('Ctrl Pts',(0.414276434602871,604.1309994978,52.0064418924366));
#105446=CARTESIAN_POINT('Ctrl Pts',(0.401375821343561,603.627974829126,
52.0060233138142));
#105447=CARTESIAN_POINT('Ctrl Pts',(0.422698891923292,603.931797866792,
51.6054949190725));
#105448=CARTESIAN_POINT('Ctrl Pts',(-0.476010708148196,604.154247142527,
51.9765750164054));
#105449=CARTESIAN_POINT('Ctrl Pts',(-0.464187114939955,603.647961634232,
51.9782978993827));
#105450=CARTESIAN_POINT('Ctrl Pts',(-0.485687802955836,603.955325698529,
51.5746539347127));
#105451=CARTESIAN_POINT('Ctrl Pts',(-1.34607093138357,604.101792845088,
52.0427987467341));
#105452=CARTESIAN_POINT('Ctrl Pts',(-1.28833508015367,603.604877677947,
52.0370249713265));
#105453=CARTESIAN_POINT('Ctrl Pts',(-1.37343881349918,603.902239020726,
51.6430377951326));
#105454=CARTESIAN_POINT('Ctrl Pts',(-2.59867283526968,603.930134794704,
52.2701959516384));
#105455=CARTESIAN_POINT('Ctrl Pts',(-2.52264148011035,603.452464870403,
52.2542948909666));
#105456=CARTESIAN_POINT('Ctrl Pts',(-2.65150548283938,603.728512385852,
51.877851247912));
#105457=CARTESIAN_POINT('Ctrl Pts',(-2.99609991422878,603.860843085546,
52.3629416887653));
#105458=CARTESIAN_POINT('Ctrl Pts',(-2.91049927803752,603.391724854142,
52.3416256351175));
#105459=CARTESIAN_POINT('Ctrl Pts',(-3.0570124876458,603.658385567216,51.9736219146518));
#105460=CARTESIAN_POINT('Ctrl Pts',(-3.78275735662804,603.69656200522,52.5884464824649));
#105461=CARTESIAN_POINT('Ctrl Pts',(-3.68456306759805,603.245201656458,
52.5572384796229));
#105462=CARTESIAN_POINT('Ctrl Pts',(-3.85966274491753,603.492124712842,
52.2064814361353));
#105463=CARTESIAN_POINT('Ctrl Pts',(-4.166979050703,603.602583843386,52.7198758782938));
#105464=CARTESIAN_POINT('Ctrl Pts',(-4.06360822860178,603.161272646565,
52.6827304516184));
#105465=CARTESIAN_POINT('Ctrl Pts',(-4.25169570801719,603.397013975051,
52.3421974164091));
#105466=CARTESIAN_POINT('Ctrl Pts',(-5.28507434996358,603.294921011766,
53.1638902156519));
#105467=CARTESIAN_POINT('Ctrl Pts',(-5.15820380454859,602.88639304024,53.1061439864781));
#105468=CARTESIAN_POINT('Ctrl Pts',(-5.39252319671762,603.085643146509,
52.8006937061186));
#105469=CARTESIAN_POINT('Ctrl Pts',(-5.98934985904857,603.054777055807,
53.5268853366489));
#105470=CARTESIAN_POINT('Ctrl Pts',(-5.86221724771992,602.668457299349,
53.4546201335385));
#105471=CARTESIAN_POINT('Ctrl Pts',(-6.11111639604364,602.842605065308,
53.1755283868843));
#105472=CARTESIAN_POINT('Ctrl Pts',(-7.32522403708878,602.536950700174,
54.3867510931747));
#105473=CARTESIAN_POINT('Ctrl Pts',(-7.20845486530068,602.185965192888,
54.3026771532069));
#105474=CARTESIAN_POINT('Ctrl Pts',(-7.47414788157401,602.318538853386,
54.0634384892156));
#105475=CARTESIAN_POINT('Ctrl Pts',(-7.93969011684976,602.266026556923,
54.8727462625326));
#105476=CARTESIAN_POINT('Ctrl Pts',(-7.83452284189274,601.930968312689,
54.7821223431411));
#105477=CARTESIAN_POINT('Ctrl Pts',(-8.10110508190108,602.044350104051,
54.5652847276252));
#105478=CARTESIAN_POINT('Ctrl Pts',(-8.78734281065214,601.864192931754,
55.6840474437808));
#105479=CARTESIAN_POINT('Ctrl Pts',(-8.70809531403379,601.544148406847,
55.6034482729444));
#105480=CARTESIAN_POINT('Ctrl Pts',(-8.96598822614471,601.637675177026,
55.4030453263832));
#105481=CARTESIAN_POINT('Ctrl Pts',(-9.05757910582421,601.730875564529,
55.9684328676932));
#105482=CARTESIAN_POINT('Ctrl Pts',(-8.98356312241737,601.41706748909,55.887647513816));
#105483=CARTESIAN_POINT('Ctrl Pts',(-9.24171805717351,601.502751403766,
55.6967061098111));
#105484=CARTESIAN_POINT('Ctrl Pts',(-9.57338818638589,601.468639030487,
56.5666721248706));
#105485=CARTESIAN_POINT('Ctrl Pts',(-9.50901929974679,601.166550377569,
56.4871657754348));
#105486=CARTESIAN_POINT('Ctrl Pts',(-9.7680129251863,601.237355039028,56.3144572329125));
#105487=CARTESIAN_POINT('Ctrl Pts',(-9.8188879556435,601.339710422266,56.8808632052432));
#105488=CARTESIAN_POINT('Ctrl Pts',(-9.7600322735385,601.042792865819,56.8025965430298));
#105489=CARTESIAN_POINT('Ctrl Pts',(-10.0185033274999,601.106872936661,
56.6388958448344));
#105490=CARTESIAN_POINT('Ctrl Pts',(-10.5031997469232,600.97186684951,57.8498081873022));
#105491=CARTESIAN_POINT('Ctrl Pts',(-10.4506899105479,600.693498726088,
57.7657813921744));
#105492=CARTESIAN_POINT('Ctrl Pts',(-10.716727326934,600.734596513586,57.6394451240119));
#105493=CARTESIAN_POINT('Ctrl Pts',(-10.8960080548356,600.749008832054,
58.5366905083561));
#105494=CARTESIAN_POINT('Ctrl Pts',(-10.8571731765776,600.476229578782,
58.4602774988305));
#105495=CARTESIAN_POINT('Ctrl Pts',(-11.1175203099313,600.509053487703,
58.3487305133394));
#105496=CARTESIAN_POINT('Ctrl Pts',(-11.3878836354649,600.463303690855,
59.6339866130622));
#105497=CARTESIAN_POINT('Ctrl Pts',(-11.3646047806954,600.197611540251,
59.5771443494444));
#105498=CARTESIAN_POINT('Ctrl Pts',(-11.619394535175,600.219906090563,59.481815015771));
#105499=CARTESIAN_POINT('Ctrl Pts',(-11.5354834909803,600.376174041301,
60.0109905179452));
#105500=CARTESIAN_POINT('Ctrl Pts',(-11.5161693648167,600.112969570056,
59.9583961633857));
#105501=CARTESIAN_POINT('Ctrl Pts',(-11.7699948379489,600.131726620416,
59.8711153341678));
#105502=CARTESIAN_POINT('Ctrl Pts',(-11.7957168424692,600.221073652832,
60.7895545484208));
#105503=CARTESIAN_POINT('Ctrl Pts',(-11.7825939140218,599.962624089532,
60.7452930450769));
#105504=CARTESIAN_POINT('Ctrl Pts',(-12.0355183921278,599.974757370073,
60.6750733074951));
#105505=CARTESIAN_POINT('Ctrl Pts',(-11.9061244276539,600.15443670383,61.1848355228865));
#105506=CARTESIAN_POINT('Ctrl Pts',(-11.8961009417762,599.897716948639,
61.145720101883));
#105507=CARTESIAN_POINT('Ctrl Pts',(-12.1481703593011,599.90731752364,61.0832468504235));
#105508=CARTESIAN_POINT('Ctrl Pts',(-12.1766841067953,599.990213528446,
62.3797203320405));
#105509=CARTESIAN_POINT('Ctrl Pts',(-12.1719915811263,599.738982030972,
62.3490805674734));
#105510=CARTESIAN_POINT('Ctrl Pts',(-12.4242303319733,599.741115461546,
62.3171054077186));
#105511=CARTESIAN_POINT('Ctrl Pts',(-12.2780801673297,599.927387168324,
63.1920557640221));
#105512=CARTESIAN_POINT('Ctrl Pts',(-12.2775058411409,599.676950745045,
63.1776792731061));
#105513=CARTESIAN_POINT('Ctrl Pts',(-12.5276874182952,599.677532219236,
63.1559355922065));
#105514=CARTESIAN_POINT('Ctrl Pts',(-12.3062333905587,599.910025891942,
64.4355871579955));
#105515=CARTESIAN_POINT('Ctrl Pts',(-12.3063643128568,599.660064767427,
64.4370638410256));
#105516=CARTESIAN_POINT('Ctrl Pts',(-12.5564129571305,599.659961751212,
64.4400267385226));
#105517=CARTESIAN_POINT('Ctrl Pts',(-12.2943819383328,599.917351224494,
64.8559276849426));
#105518=CARTESIAN_POINT('Ctrl Pts',(-12.2941718209377,599.667216361877,
64.8634434416355));
#105519=CARTESIAN_POINT('Ctrl Pts',(-12.5443205872794,599.667375345166,
64.8740772469317));
#105520=CARTESIAN_POINT('Ctrl Pts',(-12.2291210200655,599.957522719545,
65.6815257693199));
#105521=CARTESIAN_POINT('Ctrl Pts',(-12.2273094971991,599.706264077721,
65.6991136324248));
#105522=CARTESIAN_POINT('Ctrl Pts',(-12.4777330003822,599.708030881358,
65.7266035670265));
#105523=CARTESIAN_POINT('Ctrl Pts',(-12.1759469061432,599.990222710175,
66.0895695514285));
#105524=CARTESIAN_POINT('Ctrl Pts',(-12.1726163502219,599.738171023279,
66.1128812981191));
#105525=CARTESIAN_POINT('Ctrl Pts',(-12.4234779559463,599.741124867619,
66.1479562446186));
#105526=CARTESIAN_POINT('Ctrl Pts',(-12.0296993061205,600.079498308535,
66.896483765114));
#105527=CARTESIAN_POINT('Ctrl Pts',(-12.0228067561347,599.824887950255,
66.9293351464561));
#105528=CARTESIAN_POINT('Ctrl Pts',(-12.2742573339491,599.831476180105,
66.9811892328191));
#105529=CARTESIAN_POINT('Ctrl Pts',(-11.9366237554634,600.136077491239,
67.2953533735953));
#105530=CARTESIAN_POINT('Ctrl Pts',(-11.9271007354986,599.880035230897,
67.3335484589463));
#105531=CARTESIAN_POINT('Ctrl Pts',(-12.1792897304192,599.888737075378,
67.393068477219));
#105532=CARTESIAN_POINT('Ctrl Pts',(-11.7104894329877,600.272048636011,
68.0840105657425));
#105533=CARTESIAN_POINT('Ctrl Pts',(-11.6955378132595,600.0119385886,68.130976713246));
#105534=CARTESIAN_POINT('Ctrl Pts',(-11.9485583932798,600.02634658594,68.20744886739));
#105535=CARTESIAN_POINT('Ctrl Pts',(-11.5770111802493,600.351676170637,
68.474072058525));
#105536=CARTESIAN_POINT('Ctrl Pts',(-11.5583984649845,600.089389930813,
68.5257596552219));
#105537=CARTESIAN_POINT('Ctrl Pts',(-11.8123667673947,600.10693354451,68.6102326743058));
#105538=CARTESIAN_POINT('Ctrl Pts',(-11.1268371472754,600.616328116227,
69.6043131395056));
#105539=CARTESIAN_POINT('Ctrl Pts',(-11.094177851908,600.347564341289,69.6760041353329));
#105540=CARTESIAN_POINT('Ctrl Pts',(-11.3530417450548,600.374774111955,
69.7773368489012));
#105541=CARTESIAN_POINT('Ctrl Pts',(-10.7586237260962,600.828487779737,
70.3144690681693));
#105542=CARTESIAN_POINT('Ctrl Pts',(-10.7127265394219,600.554881645438,
70.3951256963503));
#105543=CARTESIAN_POINT('Ctrl Pts',(-10.977343637448,600.589489857249,70.5106549236237));
#105544=CARTESIAN_POINT('Ctrl Pts',(-10.1073211782066,601.185491883109,
71.3202714227271));
#105545=CARTESIAN_POINT('Ctrl Pts',(-10.0546064812974,600.894682176268,
71.3965629016389));
#105546=CARTESIAN_POINT('Ctrl Pts',(-10.3128000119404,600.950796158203,
71.5492638109212));
#105547=CARTESIAN_POINT('Ctrl Pts',(-9.87372685329524,601.310849208256,
71.6449099002616));
#105548=CARTESIAN_POINT('Ctrl Pts',(-9.81559960598111,601.015263109716,
71.7228833856819));
#105549=CARTESIAN_POINT('Ctrl Pts',(-10.0744570782856,601.077663941176,
71.8844906020682));
#105550=CARTESIAN_POINT('Ctrl Pts',(-9.38227834633797,601.566923442202,
72.2630638437438));
#105551=CARTESIAN_POINT('Ctrl Pts',(-9.3145103182014,601.260463878945,72.3432405042314));
#105552=CARTESIAN_POINT('Ctrl Pts',(-9.57301801983148,601.336823742793,
72.5228060041743));
#105553=CARTESIAN_POINT('Ctrl Pts',(-9.12341151926098,601.698209069844,
72.5582161648588));
#105554=CARTESIAN_POINT('Ctrl Pts',(-9.05028270509329,601.385990165768,
72.6387917490736));
#105555=CARTESIAN_POINT('Ctrl Pts',(-9.3088888014544,601.469691282284,72.827584871394));
#105556=CARTESIAN_POINT('Ctrl Pts',(-8.57939679683925,601.964234737923,
73.1220252238533));
#105557=CARTESIAN_POINT('Ctrl Pts',(-8.49692150109579,601.639184717617,
73.2025036527718));
#105558=CARTESIAN_POINT('Ctrl Pts',(-8.7538148761466,601.738922456514,73.4097827545099));
#105559=CARTESIAN_POINT('Ctrl Pts',(-8.29425119061942,602.098983695525,
73.3906801363316));
#105560=CARTESIAN_POINT('Ctrl Pts',(-8.20674465006721,601.767076389366,
73.4702530911213));
#105561=CARTESIAN_POINT('Ctrl Pts',(-8.46287263080745,601.87529508383,73.6871999316855));
#105562=CARTESIAN_POINT('Ctrl Pts',(-7.69661684926344,602.368731641435,
73.9019070495361));
#105563=CARTESIAN_POINT('Ctrl Pts',(-7.60084562786787,602.021848838989,
73.978892784628));
#105564=CARTESIAN_POINT('Ctrl Pts',(-7.85308898859088,602.148293430223,
74.2151005589185));
#105565=CARTESIAN_POINT('Ctrl Pts',(-7.3826036898993,602.504320561377,74.1454188990161));
#105566=CARTESIAN_POINT('Ctrl Pts',(-7.2827409284724,602.14927957797,74.2199817961026));
#105567=CARTESIAN_POINT('Ctrl Pts',(-7.53269227808984,602.285516183211,
74.4665545912257));
#105568=CARTESIAN_POINT('Ctrl Pts',(-6.41396819947268,602.898960048218,
74.8243434255003));
#105569=CARTESIAN_POINT('Ctrl Pts',(-6.28966522125246,602.524247689671,
74.9017755309047));
#105570=CARTESIAN_POINT('Ctrl Pts',(-6.54436688094673,602.684910409883,
75.1676209958109));
#105571=CARTESIAN_POINT('Ctrl Pts',(-5.73027341984355,603.147668316788,
75.2121345157478));
#105572=CARTESIAN_POINT('Ctrl Pts',(-5.60308614276544,602.751935967381,
75.2765310704285));
#105573=CARTESIAN_POINT('Ctrl Pts',(-5.84677300034353,602.936615919209,
75.5680603372252));
#105574=CARTESIAN_POINT('Ctrl Pts',(-4.64077478504796,603.475567974207,
75.6973360141623));
#105575=CARTESIAN_POINT('Ctrl Pts',(-4.53330991520826,603.046616580981,
75.7410809439269));
#105576=CARTESIAN_POINT('Ctrl Pts',(-4.73512363414398,603.268467444644,
76.0690872002211));
#105577=CARTESIAN_POINT('Ctrl Pts',(-4.26685720707408,603.577288002825,
75.8428419591479));
#105578=CARTESIAN_POINT('Ctrl Pts',(-4.16281829720207,603.138168004403,
75.8808099165903));
#105579=CARTESIAN_POINT('Ctrl Pts',(-4.35360434329437,603.371413324949,
76.2193388306527));
#105580=CARTESIAN_POINT('Ctrl Pts',(-3.49499057985149,603.760663649314,
76.0994932686235));
#105581=CARTESIAN_POINT('Ctrl Pts',(-3.40047115190971,603.302798678709,
76.127370335997));
#105582=CARTESIAN_POINT('Ctrl Pts',(-3.56604570114687,603.556998827382,
76.4843606975452));
#105583=CARTESIAN_POINT('Ctrl Pts',(-3.09852828926658,603.841732331683,
76.209817468087));
#105584=CARTESIAN_POINT('Ctrl Pts',(-3.01184896420214,603.374403504358,
76.2318455359098));
#105585=CARTESIAN_POINT('Ctrl Pts',(-3.16152317445561,603.639044536767,
76.5982831453344));
#105586=CARTESIAN_POINT('Ctrl Pts',(-1.85454421888672,604.050252953775,
76.4896756819632));
#105587=CARTESIAN_POINT('Ctrl Pts',(-1.77973073553379,603.560927559414,
76.5008366075293));
#105588=CARTESIAN_POINT('Ctrl Pts',(-1.89224989736498,603.850077894776,
76.8872684979557));
#105589=CARTESIAN_POINT('Ctrl Pts',(-0.988247314630766,604.13061698373,
76.5918392124698));
#105590=CARTESIAN_POINT('Ctrl Pts',(-0.956219519859947,603.627396775914,
76.5919508447176));
#105591=CARTESIAN_POINT('Ctrl Pts',(-1.00833932243225,603.931410759391,
76.9927644491201));
#105592=CARTESIAN_POINT('Ctrl Pts',(-0.0982453008758767,604.136097666981,
76.5990932436933));
#105593=CARTESIAN_POINT('Ctrl Pts',(-0.0952647792021157,603.632400531367,
76.599098861278));
#105594=CARTESIAN_POINT('Ctrl Pts',(-0.100242643564831,603.936957478099,
77.0002550481944));
#105595=CARTESIAN_POINT('Ctrl Pts',(-3.19988829303768,606.469280540506,
48.9136642374327));
#105596=CARTESIAN_POINT('Ctrl Pts',(-3.17805581403023,606.368972937512,
48.9095429260867));
#105597=CARTESIAN_POINT('Ctrl Pts',(-3.14894350373811,606.298042353055,
48.9762189002942));
#105598=CARTESIAN_POINT('Ctrl Pts',(-2.29881116825274,606.675089727992,
48.7191843933304));
#105599=CARTESIAN_POINT('Ctrl Pts',(-2.2887449963298,606.576903980715,48.7179545736899));
#105600=CARTESIAN_POINT('Ctrl Pts',(-2.26217542629362,606.506333644761,
48.7825198374689));
#105601=CARTESIAN_POINT('Ctrl Pts',(-1.29934864768706,606.803120537005,
48.6030696395544));
#105602=CARTESIAN_POINT('Ctrl Pts',(-1.29103235676735,606.707136696867,
48.60278157187));
#105603=CARTESIAN_POINT('Ctrl Pts',(-1.27865210531907,606.635902859048,
48.6668762936877));
#105604=CARTESIAN_POINT('Ctrl Pts',(0.24604904762521,606.835470312073,48.5736280341214));
#105605=CARTESIAN_POINT('Ctrl Pts',(0.244224674588171,606.73987097646,48.5737334451187));
#105606=CARTESIAN_POINT('Ctrl Pts',(0.242130489444806,606.668642047065,
48.6375535275709));
#105607=CARTESIAN_POINT('Ctrl Pts',(0.793683375382584,606.815063542801,
48.5920594319863));
#105608=CARTESIAN_POINT('Ctrl Pts',(0.788931574693909,606.719170048466,
48.5919652205538));
#105609=CARTESIAN_POINT('Ctrl Pts',(0.781040459010405,606.64798975616,48.6559104137992));
#105610=CARTESIAN_POINT('Ctrl Pts',(2.39693158170349,606.666816236979,48.7280101254697));
#105611=CARTESIAN_POINT('Ctrl Pts',(2.38338099377126,606.568997554172,48.7262413336859));
#105612=CARTESIAN_POINT('Ctrl Pts',(2.35874810817502,606.497958314614,48.7913119902478));
#105613=CARTESIAN_POINT('Ctrl Pts',(3.42759398731837,606.453238126653,48.9240904248496));
#105614=CARTESIAN_POINT('Ctrl Pts',(3.41253860309944,606.350806509426,48.9217203889832));
#105615=CARTESIAN_POINT('Ctrl Pts',(3.37298184661566,606.281814298726,48.9865958531241));
#105616=CARTESIAN_POINT('Ctrl Pts',(4.67730317816144,606.08414261949,49.2909483904667));
#105617=CARTESIAN_POINT('Ctrl Pts',(4.64765158093344,605.979218089358,49.2817265518851));
#105618=CARTESIAN_POINT('Ctrl Pts',(4.60280256700888,605.908271263799,49.3519775736338));
#105619=CARTESIAN_POINT('Ctrl Pts',(4.92564398215479,606.005058421566,49.3706595461052));
#105620=CARTESIAN_POINT('Ctrl Pts',(4.89464885506363,605.899071341731,49.3604691881233));
#105621=CARTESIAN_POINT('Ctrl Pts',(4.84718746008084,605.828235404484,49.4313666860679));
#105622=CARTESIAN_POINT('Ctrl Pts',(5.41204506061927,605.840019435411,49.5400282810896));
#105623=CARTESIAN_POINT('Ctrl Pts',(5.37840998526052,605.731861424371,49.5277111330022));
#105624=CARTESIAN_POINT('Ctrl Pts',(5.32584062015217,605.661210311973,49.6000512954549));
#105625=CARTESIAN_POINT('Ctrl Pts',(5.65096311005464,605.753831257063,49.6299136263926));
#105626=CARTESIAN_POINT('Ctrl Pts',(5.61612178002961,605.644482421254,49.6165277399625));
#105627=CARTESIAN_POINT('Ctrl Pts',(5.560952773411,605.573985070646,49.6895734166024));
#105628=CARTESIAN_POINT('Ctrl Pts',(6.35597407519104,605.486109076522,49.914631946893));
#105629=CARTESIAN_POINT('Ctrl Pts',(6.3194193662171,605.37241162902,49.8984892971421));
#105630=CARTESIAN_POINT('Ctrl Pts',(6.25472898600277,605.303043055918,49.9731396605117));
#105631=CARTESIAN_POINT('Ctrl Pts',(6.81038188975856,605.295478966058,50.1244671165347));
#105632=CARTESIAN_POINT('Ctrl Pts',(6.77205222396561,605.178792243254,50.1062416227097));
#105633=CARTESIAN_POINT('Ctrl Pts',(6.701897426018,605.110120024701,50.182125854026));
#105634=CARTESIAN_POINT('Ctrl Pts',(7.69221803306948,604.897969035652,50.5829910891641));
#105635=CARTESIAN_POINT('Ctrl Pts',(7.65049736475128,604.775365019841,50.5595723308578));
#105636=CARTESIAN_POINT('Ctrl Pts',(7.56968515550792,604.707828059185,50.6387960920346));
#105637=CARTESIAN_POINT('Ctrl Pts',(8.11963001506569,604.691064632854,50.831690360471));
#105638=CARTESIAN_POINT('Ctrl Pts',(8.07671976444598,604.564987929527,50.8060183026104));
#105639=CARTESIAN_POINT('Ctrl Pts',(7.99028738530161,604.498435512279,50.8864885495719));
#105640=CARTESIAN_POINT('Ctrl Pts',(8.94997490797288,604.267311159281,51.3685986628816));
#105641=CARTESIAN_POINT('Ctrl Pts',(8.90504619960583,604.134272431812,51.3374439703381));
#105642=CARTESIAN_POINT('Ctrl Pts',(8.80740286369077,604.069585786612,51.421224612497));
#105643=CARTESIAN_POINT('Ctrl Pts',(9.35449918700437,604.049511398749,51.658191408593));
#105644=CARTESIAN_POINT('Ctrl Pts',(9.30897039084129,603.912530603342,51.6247044118638));
#105645=CARTESIAN_POINT('Ctrl Pts',(9.20548162083417,603.849167476194,51.7096442401454));
#105646=CARTESIAN_POINT('Ctrl Pts',(10.5163351536716,603.398718287281,52.575739049541));
#105647=CARTESIAN_POINT('Ctrl Pts',(10.4792441450532,603.244538433826,52.5413915053251));
#105648=CARTESIAN_POINT('Ctrl Pts',(10.3487844505051,603.190561862117,52.6234603889828));
#105649=CARTESIAN_POINT('Ctrl Pts',(11.2257713012345,602.967318439238,53.2528256613287));
#105650=CARTESIAN_POINT('Ctrl Pts',(11.1886816147119,602.804026308938,53.2166715576217));
#105651=CARTESIAN_POINT('Ctrl Pts',(11.0469172883132,602.753977824126,53.2977962975316));
#105652=CARTESIAN_POINT('Ctrl Pts',(12.1992715391054,602.349475145027,54.3753501795627));
#105653=CARTESIAN_POINT('Ctrl Pts',(12.1575997879903,602.177212631392,54.3239043685375));
#105654=CARTESIAN_POINT('Ctrl Pts',(12.0049188841794,602.128700822412,54.4157870888978));
#105655=CARTESIAN_POINT('Ctrl Pts',(12.5084759793438,602.148334979507,54.7674817836186));
#105656=CARTESIAN_POINT('Ctrl Pts',(12.468217693647,601.971160873214,54.7148446167709));
#105657=CARTESIAN_POINT('Ctrl Pts',(12.3091950227289,601.925144767952,54.8063260024276));
#105658=CARTESIAN_POINT('Ctrl Pts',(13.0952716020131,601.759739638709,55.5911613762021));
#105659=CARTESIAN_POINT('Ctrl Pts',(13.0590920906578,601.57224116281,55.5364326108686));
#105660=CARTESIAN_POINT('Ctrl Pts',(12.8866359918322,601.531883514801,55.6266595150127));
#105661=CARTESIAN_POINT('Ctrl Pts',(13.3695604686926,601.574466672933,56.0182814407224));
#105662=CARTESIAN_POINT('Ctrl Pts',(13.3352634364091,601.381993339191,55.9630634399456));
#105663=CARTESIAN_POINT('Ctrl Pts',(13.1565527246595,601.344385932193,56.0520433785379));
#105664=CARTESIAN_POINT('Ctrl Pts',(14.1299035774209,601.054020239008,57.3393334951756));
#105665=CARTESIAN_POINT('Ctrl Pts',(14.1102991866389,600.8410628099,57.2962949053191));
#105666=CARTESIAN_POINT('Ctrl Pts',(13.9047588183333,600.817702811084,57.3676988812898));
#105667=CARTESIAN_POINT('Ctrl Pts',(14.5566498549489,600.752285916186,58.2756573376281));
#105668=CARTESIAN_POINT('Ctrl Pts',(14.5388220217875,600.531827565967,58.2336812825481));
#105669=CARTESIAN_POINT('Ctrl Pts',(14.3247076934254,600.512343480275,58.3002140367116));
#105670=CARTESIAN_POINT('Ctrl Pts',(14.9788110762547,600.450302189345,59.5276607666015));
#105671=CARTESIAN_POINT('Ctrl Pts',(14.9637997646997,600.221753346202,59.4803694808452));
#105672=CARTESIAN_POINT('Ctrl Pts',(14.7401433929711,600.206732629765,59.5471387316693));
#105673=CARTESIAN_POINT('Ctrl Pts',(15.0576058396701,600.393695366213,59.7823928247067));
#105674=CARTESIAN_POINT('Ctrl Pts',(15.0439529783748,600.163016122539,59.7367889937232));
#105675=CARTESIAN_POINT('Ctrl Pts',(14.817681362334,600.149447045719,59.8008321998986));
#105676=CARTESIAN_POINT('Ctrl Pts',(15.2014471033479,600.290045047794,60.2930389236187));
#105677=CARTESIAN_POINT('Ctrl Pts',(15.1905205855739,600.055282853514,60.251366404023));
#105678=CARTESIAN_POINT('Ctrl Pts',(14.9592279732983,600.044554175989,60.3093954217729));
#105679=CARTESIAN_POINT('Ctrl Pts',(15.2668116417703,600.242774489,60.5498362104747));
#105680=CARTESIAN_POINT('Ctrl Pts',(15.2571084270983,600.006159201186,60.5101927719224));
#105681=CARTESIAN_POINT('Ctrl Pts',(15.0235498579243,599.996716902792,60.565145240021));
#105682=CARTESIAN_POINT('Ctrl Pts',(15.4433255182961,600.114823816367,61.3246595339165));
#105683=CARTESIAN_POINT('Ctrl Pts',(15.4377062255518,599.87261425957,61.2940470335774));
#105684=CARTESIAN_POINT('Ctrl Pts',(15.1972467822461,599.867233281471,61.336802882892));
#105685=CARTESIAN_POINT('Ctrl Pts',(15.5349475887123,600.047983519335,61.8471069255291));
#105686=CARTESIAN_POINT('Ctrl Pts',(15.5309261439817,599.803232323736,61.8206844364526));
#105687=CARTESIAN_POINT('Ctrl Pts',(15.2874077780673,599.799591424263,61.8571195614638));
#105688=CARTESIAN_POINT('Ctrl Pts',(15.6652986681034,599.95273223585,62.9040820559312));
#105689=CARTESIAN_POINT('Ctrl Pts',(15.6642372322958,599.703849135545,62.8892513959474));
#105690=CARTESIAN_POINT('Ctrl Pts',(15.4156790030778,599.703198773326,62.9097786108428));
#105691=CARTESIAN_POINT('Ctrl Pts',(15.7040356606937,599.92431421945,63.4386078350693));
#105692=CARTESIAN_POINT('Ctrl Pts',(15.7037030786927,599.674309310564,63.4286901969925));
#105693=CARTESIAN_POINT('Ctrl Pts',(15.4537982322339,599.674440013257,63.4421236247391));
#105694=CARTESIAN_POINT('Ctrl Pts',(15.720555575138,599.912202987333,64.2499277579685));
#105695=CARTESIAN_POINT('Ctrl Pts',(15.720610340671,599.661663071146,64.2494068634906));
#105696=CARTESIAN_POINT('Ctrl Pts',(15.4700545523028,599.662183666258,64.2501300119848));
#105697=CARTESIAN_POINT('Ctrl Pts',(15.7190604657519,599.913299687284,64.5230557734976));
#105698=CARTESIAN_POINT('Ctrl Pts',(15.7190815934227,599.66280716433,64.5256053426526));
#105699=CARTESIAN_POINT('Ctrl Pts',(15.4685832963051,599.663293508665,64.5221427161502));
#105700=CARTESIAN_POINT('Ctrl Pts',(15.7019650213429,599.925831247008,65.0657280699177));
#105701=CARTESIAN_POINT('Ctrl Pts',(15.7015814327667,599.675895175684,65.0746869533344));
#105702=CARTESIAN_POINT('Ctrl Pts',(15.451760636994,599.675975214018,65.0625984317746));
#105703=CARTESIAN_POINT('Ctrl Pts',(15.6864384446807,599.937211941789,65.3354120618728));
#105704=CARTESIAN_POINT('Ctrl Pts',(15.685708149129,599.687765621734,65.3473542470335));
#105705=CARTESIAN_POINT('Ctrl Pts',(15.4364817742615,599.68749229307,65.3311812375999));
#105706=CARTESIAN_POINT('Ctrl Pts',(15.574852527381,600.01890054518,66.675805476863));
#105707=CARTESIAN_POINT('Ctrl Pts',(15.5718851336501,599.772777987196,66.6988378773207));
#105708=CARTESIAN_POINT('Ctrl Pts',(15.326675704598,599.770160170402,66.6661082158762));
#105709=CARTESIAN_POINT('Ctrl Pts',(15.3780196332794,600.163132045658,67.7226505757277));
#105710=CARTESIAN_POINT('Ctrl Pts',(15.3741355634771,599.920662093309,67.747428907255));
#105711=CARTESIAN_POINT('Ctrl Pts',(15.132976851256,599.916124774213,67.7086964322209));
#105712=CARTESIAN_POINT('Ctrl Pts',(14.7749830115725,600.596964732154,69.7677006850111));
#105713=CARTESIAN_POINT('Ctrl Pts',(14.7598045961286,600.371477433906,69.8078650818197));
#105714=CARTESIAN_POINT('Ctrl Pts',(14.5395600793771,600.355158450615,69.7454059551599));
#105715=CARTESIAN_POINT('Ctrl Pts',(14.3794203054433,600.878842159056,70.7298312303411));
#105716=CARTESIAN_POINT('Ctrl Pts',(14.3625245593818,600.660409929034,70.7712664447535));
#105717=CARTESIAN_POINT('Ctrl Pts',(14.1502976929657,600.640422389231,70.7036228750291));
#105718=CARTESIAN_POINT('Ctrl Pts',(13.6612091794102,601.375545247691,72.0904647072316));
#105719=CARTESIAN_POINT('Ctrl Pts',(13.6295943491115,601.177288380591,72.1457661580741));
#105720=CARTESIAN_POINT('Ctrl Pts',(13.443551570198,601.143076802614,72.0586962144295));
#105721=CARTESIAN_POINT('Ctrl Pts',(13.3993396267296,601.554487162714,72.5323553744969));
#105722=CARTESIAN_POINT('Ctrl Pts',(13.3656347598373,601.361245735362,72.5875774487108));
#105723=CARTESIAN_POINT('Ctrl Pts',(13.1858564258026,601.324166988977,72.4987899104211));
#105724=CARTESIAN_POINT('Ctrl Pts',(12.8404364611288,601.929557948488,73.3794426010547));
#105725=CARTESIAN_POINT('Ctrl Pts',(12.8021776094239,601.74676344862,73.4333645836814));
#105726=CARTESIAN_POINT('Ctrl Pts',(12.6358638843131,601.703740500343,73.3424344241913));
#105727=CARTESIAN_POINT('Ctrl Pts',(12.5440885772941,602.125255881405,73.7841389135551));
#105728=CARTESIAN_POINT('Ctrl Pts',(12.5042121997376,601.947423525011,73.8371312504687));
#105729=CARTESIAN_POINT('Ctrl Pts',(12.3442395607509,601.901788659894,73.7454864680693));
#105730=CARTESIAN_POINT('Ctrl Pts',(11.9187059559954,602.528995443253,74.5589805782249));
#105731=CARTESIAN_POINT('Ctrl Pts',(11.8756740810911,602.361062922652,74.608774052379));
#105732=CARTESIAN_POINT('Ctrl Pts',(11.7288256021108,602.310377386317,74.5171827762026));
#105733=CARTESIAN_POINT('Ctrl Pts',(11.5896694934917,602.737052077775,74.929116152772));
#105734=CARTESIAN_POINT('Ctrl Pts',(11.5456832679029,602.573835505882,74.9772519297626));
#105735=CARTESIAN_POINT('Ctrl Pts',(11.4050330289474,602.52093362206,74.8858160421481));
#105736=CARTESIAN_POINT('Ctrl Pts',(10.8985267731535,603.161627468999,75.6366626093528));
#105737=CARTESIAN_POINT('Ctrl Pts',(10.8529135843586,603.007589543647,75.6803058137441));
#105738=CARTESIAN_POINT('Ctrl Pts',(10.7249053554303,602.950610664589,75.5904935058699));
#105739=CARTESIAN_POINT('Ctrl Pts',(10.5350707806408,603.378936903845,75.9751917541415));
#105740=CARTESIAN_POINT('Ctrl Pts',(10.4891833026196,603.229336765336,76.0167162365071));
#105741=CARTESIAN_POINT('Ctrl Pts',(10.3672411512527,603.17053175624,75.9276498830206));
#105742=CARTESIAN_POINT('Ctrl Pts',(9.40196706845938,604.031564136161,76.9346610568732));
#105743=CARTESIAN_POINT('Ctrl Pts',(9.36501835682024,603.889166409255,76.9607377506827));
#105744=CARTESIAN_POINT('Ctrl Pts',(9.25217348404495,603.831015928072,76.88324984583));
#105745=CARTESIAN_POINT('Ctrl Pts',(8.59738601729796,604.464173010235,77.495276682365));
#105746=CARTESIAN_POINT('Ctrl Pts',(8.56117701294624,604.330686616535,77.5194907589741));
#105747=CARTESIAN_POINT('Ctrl Pts',(8.4604132495034,604.268823621313,77.441588613324));
#105748=CARTESIAN_POINT('Ctrl Pts',(7.30535316787382,605.076707446709,78.2257709379294));
#105749=CARTESIAN_POINT('Ctrl Pts',(7.26509469234165,604.956716878247,78.2466972418932));
#105750=CARTESIAN_POINT('Ctrl Pts',(7.18898333288885,604.88871679835,78.1691179476838));
#105751=CARTESIAN_POINT('Ctrl Pts',(6.86031993687873,605.274722637669,78.4506791819244));
#105752=CARTESIAN_POINT('Ctrl Pts',(6.82166576422317,605.157894830494,78.4694208274701));
#105753=CARTESIAN_POINT('Ctrl Pts',(6.75104020321707,605.08911360307,78.3931160864464));
#105754=CARTESIAN_POINT('Ctrl Pts',(5.93704365902223,605.650813351207,78.8621698493515));
#105755=CARTESIAN_POINT('Ctrl Pts',(5.90261839496408,605.539281559552,78.8760152018326));
#105756=CARTESIAN_POINT('Ctrl Pts',(5.84247174669302,605.469729402818,78.8029438408065));
#105757=CARTESIAN_POINT('Ctrl Pts',(5.45630243005711,605.829574494848,79.0493901878842));
#105758=CARTESIAN_POINT('Ctrl Pts',(5.4239784887906,605.720769173563,79.0613189453554));
#105759=CARTESIAN_POINT('Ctrl Pts',(5.3693892829349,605.650640892095,78.9894068856549));
#105760=CARTESIAN_POINT('Ctrl Pts',(3.58020877348986,606.444076927432,79.6742394973212));
#105761=CARTESIAN_POINT('Ctrl Pts',(3.57309729366402,606.338334356746,79.6733677985972));
#105762=CARTESIAN_POINT('Ctrl Pts',(3.52314404231912,606.27255059228,79.6117444882699));
#105763=CARTESIAN_POINT('Ctrl Pts',(2.11068986974404,606.758383033869,79.9525257968984));
#105764=CARTESIAN_POINT('Ctrl Pts',(2.10064307571136,606.662766022507,79.9545722314202));
#105765=CARTESIAN_POINT('Ctrl Pts',(2.07707015569879,606.59062346792,79.8888901782391));
#105766=CARTESIAN_POINT('Ctrl Pts',(0.520472181601657,606.818551326338,
80.0111755919482));
#105767=CARTESIAN_POINT('Ctrl Pts',(0.516051949937491,606.722294695726,
80.010640113492));
#105768=CARTESIAN_POINT('Ctrl Pts',(0.512173775986833,606.651521964532,
79.9473100409873));
#105769=CARTESIAN_POINT('Ctrl Pts',(3.96801791420419,607.866317116503,49.0902664690719));
#105770=CARTESIAN_POINT('Ctrl Pts',(4.14330398514067,608.4803723312,49.135784443382));
#105771=CARTESIAN_POINT('Ctrl Pts',(3.90492814046806,608.028944351104,49.5221152198147));
#105772=CARTESIAN_POINT('Ctrl Pts',(2.93755241708741,608.17547753474,48.8214432993782));
#105773=CARTESIAN_POINT('Ctrl Pts',(3.03742703523094,608.85281628291,48.8340694353193));
#105774=CARTESIAN_POINT('Ctrl Pts',(2.89083941502255,608.334185987686,49.2609200704409));
#105775=CARTESIAN_POINT('Ctrl Pts',(1.86937071966544,608.386087168575,48.6534581338969));
#105776=CARTESIAN_POINT('Ctrl Pts',(1.96126338871385,609.089531292228,48.6607567236558));
#105777=CARTESIAN_POINT('Ctrl Pts',(1.83964868601656,608.542122065273,49.0977046826072));
#105778=CARTESIAN_POINT('Ctrl Pts',(0.214693779414581,608.48610855861,48.5730542692393));
#105779=CARTESIAN_POINT('Ctrl Pts',(0.22416099289284,609.20948373918,48.5717336255605));
#105780=CARTESIAN_POINT('Ctrl Pts',(0.211280116816066,608.640874904755,
49.0195828117931));
#105781=CARTESIAN_POINT('Ctrl Pts',(-0.327665155014435,608.483177231892,
48.5753871894563));
#105782=CARTESIAN_POINT('Ctrl Pts',(-0.343446449653063,609.205974202863,
48.5743085001531));
#105783=CARTESIAN_POINT('Ctrl Pts',(-0.32245537920764,608.637980757633,
49.0218495189568));
#105784=CARTESIAN_POINT('Ctrl Pts',(-1.4014344262471,608.409659806134,48.6345369452367));
#105785=CARTESIAN_POINT('Ctrl Pts',(-1.47715237700547,609.117321616503,
48.64016712078));
#105786=CARTESIAN_POINT('Ctrl Pts',(-1.37915307127922,608.56539568904,49.0793205445456));
#105787=CARTESIAN_POINT('Ctrl Pts',(-1.93284944505609,608.339110567767,
48.6913595421491));
#105788=CARTESIAN_POINT('Ctrl Pts',(-2.0296182397685,609.034247951133,48.7019273602932));
#105789=CARTESIAN_POINT('Ctrl Pts',(-1.90211842335103,608.49574134848,49.1345303092449));
#105790=CARTESIAN_POINT('Ctrl Pts',(-2.98554566101708,608.137526014925,
48.858111903559));
#105791=CARTESIAN_POINT('Ctrl Pts',(-3.12573547424559,608.796071607189,
48.8844736999009));
#105792=CARTESIAN_POINT('Ctrl Pts',(-2.93807698482498,608.296713492016,
49.2965498576802));
#105793=CARTESIAN_POINT('Ctrl Pts',(-3.50954896370793,608.005382116136,
48.969093235558));
#105794=CARTESIAN_POINT('Ctrl Pts',(-3.66252614078184,608.644062322836,
49.0028670929732));
#105795=CARTESIAN_POINT('Ctrl Pts',(-3.45374791090643,608.166245890445,
49.4043809868049));
#105796=CARTESIAN_POINT('Ctrl Pts',(-4.51869902314397,607.699442312391,
49.2356474341197));
#105797=CARTESIAN_POINT('Ctrl Pts',(-4.69335204058046,608.293267867564,
49.2876872236527));
#105798=CARTESIAN_POINT('Ctrl Pts',(-4.4468510663278,607.864186714045,49.6633692434331));
#105799=CARTESIAN_POINT('Ctrl Pts',(-5.00754801428308,607.525295392799,
49.3915102529955));
#105800=CARTESIAN_POINT('Ctrl Pts',(-5.18656612683327,608.098169557262,
49.4506178691369));
#105801=CARTESIAN_POINT('Ctrl Pts',(-4.92792605251174,607.692249047515,
49.8148076425706));
#105802=CARTESIAN_POINT('Ctrl Pts',(-5.95917956692152,607.146457363669,
49.7457424205663));
#105803=CARTESIAN_POINT('Ctrl Pts',(-6.14248615971886,607.676200520949,
49.8207309756671));
#105804=CARTESIAN_POINT('Ctrl Pts',(-5.86442374504572,607.318216782459,
50.1589844638927));
#105805=CARTESIAN_POINT('Ctrl Pts',(-6.42237014149181,606.941534503285,
49.9443408012826));
#105806=CARTESIAN_POINT('Ctrl Pts',(-6.60402168968751,607.451986108322,
50.0247610850771));
#105807=CARTESIAN_POINT('Ctrl Pts',(-6.32024772390201,607.115893757345,
50.351944968455));
#105808=CARTESIAN_POINT('Ctrl Pts',(-7.32445419098543,606.511057101471,
50.382970765863));
#105809=CARTESIAN_POINT('Ctrl Pts',(-7.49937336947291,606.983731036464,
50.4751585816833));
#105810=CARTESIAN_POINT('Ctrl Pts',(-7.20798452548951,606.690877640335,
50.7781230179888));
#105811=CARTESIAN_POINT('Ctrl Pts',(-7.75780268783224,606.2882218126,50.6202380193044));
#105812=CARTESIAN_POINT('Ctrl Pts',(-7.92808282222848,606.744119548409,
50.7161247240279));
#105813=CARTESIAN_POINT('Ctrl Pts',(-7.63444059270741,606.47086953048,51.0086543329385));
#105814=CARTESIAN_POINT('Ctrl Pts',(-9.01263265026788,605.608324932273,
51.3844819472612));
#105815=CARTESIAN_POINT('Ctrl Pts',(-9.13407034427913,606.035261719809,
51.4724609662051));
#105816=CARTESIAN_POINT('Ctrl Pts',(-8.86930646895302,605.799601467611,
51.7511985187908));
#105817=CARTESIAN_POINT('Ctrl Pts',(-9.78960325654476,605.140274398618,
51.9632424341007));
#105818=CARTESIAN_POINT('Ctrl Pts',(-9.90255020916191,605.540902676885,
52.0496752501994));
#105819=CARTESIAN_POINT('Ctrl Pts',(-9.63391884695173,605.337489533059,
52.3135263786952));
#105820=CARTESIAN_POINT('Ctrl Pts',(-10.878441060838,604.447130009809,52.9432807545543));
#105821=CARTESIAN_POINT('Ctrl Pts',(-10.9910069155268,604.800649737504,
53.0515055379338));
#105822=CARTESIAN_POINT('Ctrl Pts',(-10.705439897833,604.653137356637,53.2657428837752));
#105823=CARTESIAN_POINT('Ctrl Pts',(-11.229472953103,604.216715305371,53.2899442539113));
#105824=CARTESIAN_POINT('Ctrl Pts',(-11.3347418937742,604.560585814078,
53.3968965258403));
#105825=CARTESIAN_POINT('Ctrl Pts',(-11.0508876799252,604.425646230675,
53.6025635511897));
#105826=CARTESIAN_POINT('Ctrl Pts',(-11.900792348141,603.766050073307,54.0193011734408));
#105827=CARTESIAN_POINT('Ctrl Pts',(-11.9901371105211,604.093157709212,
54.1232083059766));
#105828=CARTESIAN_POINT('Ctrl Pts',(-11.7115273981156,603.980699367114,
54.31121164042));
#105829=CARTESIAN_POINT('Ctrl Pts',(-12.218293964521,603.547715900985,54.3987594591597));
#105830=CARTESIAN_POINT('Ctrl Pts',(-12.3010560005085,603.866740147379,
54.5005517772709));
#105831=CARTESIAN_POINT('Ctrl Pts',(-12.0239781544445,603.765135486367,
54.679895712359));
#105832=CARTESIAN_POINT('Ctrl Pts',(-13.1176253793484,602.918861575623,
55.5830589493271));
#105833=CARTESIAN_POINT('Ctrl Pts',(-13.1641372034305,603.22841419151,55.657554710526));
#105834=CARTESIAN_POINT('Ctrl Pts',(-12.9089989609887,603.14426280659,55.8305641478284));
#105835=CARTESIAN_POINT('Ctrl Pts',(-13.6470291437565,602.534223643058,
56.4332097702865));
#105836=CARTESIAN_POINT('Ctrl Pts',(-13.6882441199942,602.827954606069,
56.502781818501));
#105837=CARTESIAN_POINT('Ctrl Pts',(-13.4299816943561,602.764504555706,
56.6565755853746));
#105838=CARTESIAN_POINT('Ctrl Pts',(-14.2141551453113,602.115068208418,
57.5846512128922));
#105839=CARTESIAN_POINT('Ctrl Pts',(-14.2513227291177,602.390507222111,
57.6633206048862));
#105840=CARTESIAN_POINT('Ctrl Pts',(-13.9880869203314,602.350666237017,
57.7753259736852));
#105841=CARTESIAN_POINT('Ctrl Pts',(-14.3227879338756,602.03433920249,57.8194266921124));
#105842=CARTESIAN_POINT('Ctrl Pts',(-14.3573300164066,602.307756077497,
57.895659279968));
#105843=CARTESIAN_POINT('Ctrl Pts',(-14.0949913651594,602.27096161042,58.0034349097068));
#105844=CARTESIAN_POINT('Ctrl Pts',(-14.5300235323771,601.879661641812,
58.298500421927));
#105845=CARTESIAN_POINT('Ctrl Pts',(-14.5593558255444,602.14943315443,58.3695243760315));
#105846=CARTESIAN_POINT('Ctrl Pts',(-14.2989297883243,602.118246805598,
58.4689050674605));
#105847=CARTESIAN_POINT('Ctrl Pts',(-14.628948992512,601.805469397078,58.5437030695108));
#105848=CARTESIAN_POINT('Ctrl Pts',(-14.655901579792,602.07345265176,58.6120969468063));
#105849=CARTESIAN_POINT('Ctrl Pts',(-14.3962813329383,602.044995995787,
58.707145038779));
#105850=CARTESIAN_POINT('Ctrl Pts',(-14.9068849327433,601.596250680114,
59.2865392357633));
#105851=CARTESIAN_POINT('Ctrl Pts',(-14.9255658148712,601.860526194702,
59.3430538394069));
#105852=CARTESIAN_POINT('Ctrl Pts',(-14.6697948864641,601.838432364643,
59.4288869888394));
#105853=CARTESIAN_POINT('Ctrl Pts',(-15.0672776140326,601.474447273842,
59.7911438168927));
#105854=CARTESIAN_POINT('Ctrl Pts',(-15.08273458312,601.73546949696,59.8429002079945));
#105855=CARTESIAN_POINT('Ctrl Pts',(-14.8276358084694,601.718174435246,
59.919163080231));
#105856=CARTESIAN_POINT('Ctrl Pts',(-15.3375077166812,601.268350349811,
60.8197103861867));
#105857=CARTESIAN_POINT('Ctrl Pts',(-15.3461975432605,601.525017568474,
60.8592543910126));
#105858=CARTESIAN_POINT('Ctrl Pts',(-15.0935663577189,601.514692768556,
60.9185223424128));
#105859=CARTESIAN_POINT('Ctrl Pts',(-15.4473524788766,601.184046572484,
61.3436679646832));
#105860=CARTESIAN_POINT('Ctrl Pts',(-15.4538492122169,601.438551451198,
61.3780952510847));
#105861=CARTESIAN_POINT('Ctrl Pts',(-15.2016635310883,601.431458661533,
61.427601771592));
#105862=CARTESIAN_POINT('Ctrl Pts',(-15.6139481543257,601.055914086478,
62.4121180900535));
#105863=CARTESIAN_POINT('Ctrl Pts',(-15.6162781423566,601.307834796045,
62.4334323880538));
#105864=CARTESIAN_POINT('Ctrl Pts',(-15.3656085202112,601.304952112143,
62.4657118072439));
#105865=CARTESIAN_POINT('Ctrl Pts',(-15.6706008816092,601.01216067731,62.9602003371774));
#105866=CARTESIAN_POINT('Ctrl Pts',(-15.6718168191366,601.262976710226,
62.9761672199096));
#105867=CARTESIAN_POINT('Ctrl Pts',(-15.4213599206253,601.261753856115,
62.9982308158159));
#105868=CARTESIAN_POINT('Ctrl Pts',(-15.7532581285021,600.948322914108,
64.5909241146122));
#105869=CARTESIAN_POINT('Ctrl Pts',(-15.7522976417821,601.19797092063,64.5843508815025));
#105870=CARTESIAN_POINT('Ctrl Pts',(-15.5027019825929,601.198726184824,
64.5826472633091));
#105871=CARTESIAN_POINT('Ctrl Pts',(-15.6959793937825,600.992833298029,
65.6707746519288));
#105872=CARTESIAN_POINT('Ctrl Pts',(-15.6952083223957,601.244324865898,
65.6625224224092));
#105873=CARTESIAN_POINT('Ctrl Pts',(-15.4463343132364,601.242671985787,
65.6318366328334));
#105874=CARTESIAN_POINT('Ctrl Pts',(-15.4849378554675,601.155135843631,
67.011585045083));
#105875=CARTESIAN_POINT('Ctrl Pts',(-15.490748159675,601.40885389153,66.9784967286438));
#105876=CARTESIAN_POINT('Ctrl Pts',(-15.2386509518819,601.402914747705,
66.9345709030678));
#105877=CARTESIAN_POINT('Ctrl Pts',(-15.4355195703926,601.193090402008,
67.2798756894921));
#105878=CARTESIAN_POINT('Ctrl Pts',(-15.442502106951,601.447631243458,67.2436796227911));
#105879=CARTESIAN_POINT('Ctrl Pts',(-15.1900189384783,601.440387693915,
67.1952431231479));
#105880=CARTESIAN_POINT('Ctrl Pts',(-15.3240490417368,601.278497889497,
67.8082600435595));
#105881=CARTESIAN_POINT('Ctrl Pts',(-15.3338238879868,601.534796371477,
67.7656619175894));
#105882=CARTESIAN_POINT('Ctrl Pts',(-15.0803219964504,601.524711405152,
67.7086233424261));
#105883=CARTESIAN_POINT('Ctrl Pts',(-15.2618976191312,601.326027371672,
68.0691914822996));
#105884=CARTESIAN_POINT('Ctrl Pts',(-15.2731532452161,601.58337490534,68.0236001703991));
#105885=CARTESIAN_POINT('Ctrl Pts',(-15.0191594320567,601.571637777113,
67.9621453552883));
#105886=CARTESIAN_POINT('Ctrl Pts',(-15.0568797539538,601.482352444088,
68.8426074874175));
#105887=CARTESIAN_POINT('Ctrl Pts',(-15.0725761726714,601.743561229684,
68.7904931957739));
#105888=CARTESIAN_POINT('Ctrl Pts',(-14.8174033801442,601.725979297202,
68.7135999647743));
#105889=CARTESIAN_POINT('Ctrl Pts',(-14.8955047156438,601.60485941836,69.3457386057789));
#105890=CARTESIAN_POINT('Ctrl Pts',(-14.9144766233915,601.86932000505,69.2887981194078));
#105891=CARTESIAN_POINT('Ctrl Pts',(-14.6585957360926,601.846931861818,
69.202444416695));
#105892=CARTESIAN_POINT('Ctrl Pts',(-14.5255384316863,601.883267821869,
70.3285351375797));
#105893=CARTESIAN_POINT('Ctrl Pts',(-14.5537819644499,602.154045228181,
70.2605787665699));
#105894=CARTESIAN_POINT('Ctrl Pts',(-14.2945157770192,602.12180743446,70.1573336769515));
#105895=CARTESIAN_POINT('Ctrl Pts',(-14.3158676780004,602.039971826645,
70.8102881691105));
#105896=CARTESIAN_POINT('Ctrl Pts',(-14.3484256804248,602.315139349457,
70.7379242119137));
#105897=CARTESIAN_POINT('Ctrl Pts',(-14.0881807313278,602.276523121392,
70.6254072326268));
#105898=CARTESIAN_POINT('Ctrl Pts',(-13.8549669417811,602.380456141554,
71.740888971284));
#105899=CARTESIAN_POINT('Ctrl Pts',(-13.8990584488247,602.664099473411,
71.6590019112753));
#105900=CARTESIAN_POINT('Ctrl Pts',(-13.6346129612246,602.612686934738,
71.5295833283864));
#105901=CARTESIAN_POINT('Ctrl Pts',(-13.6051205939733,602.563225484241,
72.1875975711325));
#105902=CARTESIAN_POINT('Ctrl Pts',(-13.6545221187428,602.852298832617,
72.1017559982508));
#105903=CARTESIAN_POINT('Ctrl Pts',(-13.3887414345827,602.793137212809,
71.9636076884644));
#105904=CARTESIAN_POINT('Ctrl Pts',(-13.0689457304277,602.94970593194,73.0472996885173));
#105905=CARTESIAN_POINT('Ctrl Pts',(-13.1316816038927,603.249565382686,
72.9538576019717));
#105906=CARTESIAN_POINT('Ctrl Pts',(-12.8610969146662,603.174713553808,
72.7988987818575));
#105907=CARTESIAN_POINT('Ctrl Pts',(-12.7826098802753,603.153433010245,
73.4602802768307));
#105908=CARTESIAN_POINT('Ctrl Pts',(-12.851407762716,603.459987836432,73.3637342809632));
#105909=CARTESIAN_POINT('Ctrl Pts',(-12.5793162792295,603.37585565731,73.2001530637705));
#105910=CARTESIAN_POINT('Ctrl Pts',(-12.1741279655269,603.578242135018,
74.2546782628821));
#105911=CARTESIAN_POINT('Ctrl Pts',(-12.2578204673371,603.898383996172,
74.1526852709296));
#105912=CARTESIAN_POINT('Ctrl Pts',(-11.9805147599271,603.795274395457,
73.9719948691702));
#105913=CARTESIAN_POINT('Ctrl Pts',(-11.850540933587,603.800285765725,74.6375141662316));
#105914=CARTESIAN_POINT('Ctrl Pts',(-11.9410485726768,604.128622252677,
74.5332916257023));
#105915=CARTESIAN_POINT('Ctrl Pts',(-11.6620754094574,604.014500653005,
74.3439606423759));
#105916=CARTESIAN_POINT('Ctrl Pts',(-10.8391421878638,604.47762194582,75.7257195228643));
#105917=CARTESIAN_POINT('Ctrl Pts',(-10.9336515194875,604.845559188827,
75.6390199582536));
#105918=CARTESIAN_POINT('Ctrl Pts',(-10.6667627124656,604.683244822595,
75.4012723114464));
#105919=CARTESIAN_POINT('Ctrl Pts',(-10.1104306891926,604.945290954641,
76.3742823947935));
#105920=CARTESIAN_POINT('Ctrl Pts',(-10.2135091666312,605.336742210894,
76.284404155343));
#105921=CARTESIAN_POINT('Ctrl Pts',(-9.94964215326505,605.144980207816,
76.0314203061157));
#105922=CARTESIAN_POINT('Ctrl Pts',(-8.53551476998559,605.87684896143,77.5345321156382));
#105923=CARTESIAN_POINT('Ctrl Pts',(-8.66654368556738,606.321456472146,
77.4536736233639));
#105924=CARTESIAN_POINT('Ctrl Pts',(-8.39977812395367,606.064718667719,
77.1587292660183));
#105925=CARTESIAN_POINT('Ctrl Pts',(-7.68270213057855,606.344199562926,
78.0484723196597));
#105926=CARTESIAN_POINT('Ctrl Pts',(-7.82150334606978,606.819174583438,
77.9681106439715));
#105927=CARTESIAN_POINT('Ctrl Pts',(-7.56052958968753,606.526139373993,
77.6580776200298));
#105928=CARTESIAN_POINT('Ctrl Pts',(-5.83592524215899,607.216625659669,
78.9319873742395));
#105929=CARTESIAN_POINT('Ctrl Pts',(-5.97772848588468,607.774450116446,
78.880974055968));
#105930=CARTESIAN_POINT('Ctrl Pts',(-5.7431239356697,607.387497786281,78.5165117385228));
#105931=CARTESIAN_POINT('Ctrl Pts',(-4.83278432844931,607.621416094013,
79.2978208896735));
#105932=CARTESIAN_POINT('Ctrl Pts',(-4.97553001277422,608.215369388646,
79.2506052240478));
#105933=CARTESIAN_POINT('Ctrl Pts',(-4.75593424033569,607.787152471388,
78.8719595177779));
#105934=CARTESIAN_POINT('Ctrl Pts',(-3.74709337812421,607.930942425638,
79.5646350434898));
#105935=CARTESIAN_POINT('Ctrl Pts',(-3.9174004512104,608.554632246293,79.5230579121762));
#105936=CARTESIAN_POINT('Ctrl Pts',(-3.68751695705033,608.09274982526,79.1311980167394));
#105937=CARTESIAN_POINT('Origin',(52.8776183915471,601.225373764374,90.6087118617898));
#105938=CARTESIAN_POINT('',(71.,639.125373764374,90.6087118617898));
#105939=CARTESIAN_POINT('',(62.6211772316338,639.125373764374,105.888887786568));
#105940=CARTESIAN_POINT('Origin',(52.8776183915471,639.125373764374,90.6087118617898));
#105941=CARTESIAN_POINT('',(62.6211772316338,602.225373764374,105.888887786568));
#105942=CARTESIAN_POINT('',(62.6211772316338,601.225373764374,105.888887786568));
#105943=CARTESIAN_POINT('',(71.,602.225373764374,90.6087118617898));
#105944=CARTESIAN_POINT('Origin',(52.8776183915471,602.225373764374,90.6087118617898));
#105945=CARTESIAN_POINT('',(71.,601.225373764374,90.6087118617898));
#105946=CARTESIAN_POINT('Origin',(0.,640.125373764374,0.));
#105947=CARTESIAN_POINT('',(62.3523505660608,640.125373764374,104.870738441723));
#105948=CARTESIAN_POINT('',(62.3523505660608,640.125373764374,105.190554486823));
#105949=CARTESIAN_POINT('',(70.,640.125373764374,90.6087118617898));
#105950=CARTESIAN_POINT('Origin',(52.8776183915471,640.125373764374,90.6087118617898));
#105951=CARTESIAN_POINT('',(70.,640.125373764374,64.2994740882088));
#105952=CARTESIAN_POINT('',(35.7552367830941,640.125373764374,90.6087118617898));
#105953=CARTESIAN_POINT('',(35.7552367830941,640.125373764374,-5.58390168977932E-15));
#105954=CARTESIAN_POINT('',(43.4028862170334,640.125373764374,104.870738441723));
#105955=CARTESIAN_POINT('Origin',(52.8776183915471,640.125373764374,90.6087118617898));
#105956=CARTESIAN_POINT('',(43.4028862170334,640.125373764374,0.));
#105957=CARTESIAN_POINT('Origin',(0.,601.225373764374,0.));
#105958=CARTESIAN_POINT('',(70.,601.225373764374,90.6087118617898));
#105959=CARTESIAN_POINT('',(62.3523505660608,601.225373764374,104.870738441723));
#105960=CARTESIAN_POINT('Origin',(52.8776183915471,601.225373764374,90.6087118617898));
#105961=CARTESIAN_POINT('',(62.3523505660608,601.225373764374,0.));
#105962=CARTESIAN_POINT('',(43.4028862170334,601.225373764374,104.870738441723));
#105963=CARTESIAN_POINT('',(43.4028862170334,601.225373764374,105.190554486823));
#105964=CARTESIAN_POINT('',(35.7552367830941,601.225373764374,90.6087118617898));
#105965=CARTESIAN_POINT('Origin',(52.8776183915471,601.225373764374,90.6087118617898));
#105966=CARTESIAN_POINT('',(35.7552367830941,601.225373764374,64.2994740882088));
#105967=CARTESIAN_POINT('',(70.,601.225373764374,0.));
#105968=CARTESIAN_POINT('Origin',(52.8776183915471,601.225373764374,90.6087118617898));
#105969=CARTESIAN_POINT('',(34.7552367830941,602.225373764374,90.6087118617898));
#105970=CARTESIAN_POINT('',(43.1340595514603,602.225373764374,105.888887786568));
#105971=CARTESIAN_POINT('Origin',(52.8776183915471,602.225373764374,90.6087118617898));
#105972=CARTESIAN_POINT('',(43.1340595514603,639.125373764374,105.888887786568));
#105973=CARTESIAN_POINT('',(43.1340595514603,601.225373764374,105.888887786568));
#105974=CARTESIAN_POINT('',(34.7552367830941,639.125373764374,90.6087118617898));
#105975=CARTESIAN_POINT('Origin',(52.8776183915471,639.125373764374,90.6087118617898));
#105976=CARTESIAN_POINT('',(34.7552367830941,640.125373764374,90.6087118617898));
#105977=CARTESIAN_POINT('Origin',(71.,620.675373764374,64.2994740882088));
#105978=CARTESIAN_POINT('',(71.,602.225373764374,64.2994740882088));
#105979=CARTESIAN_POINT('',(71.,639.125373764374,90.6087118617898));
#105980=CARTESIAN_POINT('Origin',(34.7552367830941,640.125373764374,64.2994740882088));
#105981=CARTESIAN_POINT('',(34.7552367830941,639.125373764374,73.1199049166885));
#105982=CARTESIAN_POINT('',(34.7552367830941,602.225373764374,73.1199049166887));
#105983=CARTESIAN_POINT('Origin',(34.7552367830941,620.675373764374,64.2994740882088));
#105984=CARTESIAN_POINT('',(34.7552367830941,602.225373764374,90.6087118617898));
#105985=CARTESIAN_POINT('',(34.7552367830941,639.125373764374,64.2994740882088));
#105986=CARTESIAN_POINT('Origin',(52.8776183915471,601.125373764374,90.6087118617898));
#105987=CARTESIAN_POINT('',(43.775613700608,601.125373764374,98.7473601281983));
#105988=CARTESIAN_POINT('',(61.9796230824862,601.125373764374,98.7473601281983));
#105989=CARTESIAN_POINT('Origin',(61.8523505660607,601.125373764374,0.));
#105990=CARTESIAN_POINT('',(61.8523505660607,639.125373764374,105.467304788954));
#105991=CARTESIAN_POINT('',(61.8523505660607,639.625373764374,104.870738441723));
#105992=CARTESIAN_POINT('Ctrl Pts',(61.8523505660607,639.125373764374,105.467304788954));
#105993=CARTESIAN_POINT('Ctrl Pts',(61.8523505660608,639.270789691535,105.467304788954));
#105994=CARTESIAN_POINT('Ctrl Pts',(61.8523505660608,639.406718012507,105.388349047246));
#105995=CARTESIAN_POINT('Ctrl Pts',(61.8523505660607,639.582389805433,105.159369804922));
#105996=CARTESIAN_POINT('Ctrl Pts',(61.8523505660608,639.625373764374,105.015531405683));
#105997=CARTESIAN_POINT('Ctrl Pts',(61.8523505660607,639.625373764374,104.870738441723));
#105998=CARTESIAN_POINT('',(61.8523505660607,639.625373764374,99.080638124754));
#105999=CARTESIAN_POINT('',(61.8523505660607,639.625373764374,98.8874960354436));
#106000=CARTESIAN_POINT('',(61.8523505660607,601.725373764374,99.080638124754));
#106001=CARTESIAN_POINT('',(61.8523505660607,601.225373764374,99.080638124754));
#106002=CARTESIAN_POINT('',(61.8523505660607,601.725373764374,104.870738441723));
#106003=CARTESIAN_POINT('',(61.8523505660607,601.725373764374,0.));
#106004=CARTESIAN_POINT('',(61.8523505660607,602.225373764374,105.467304788954));
#106005=CARTESIAN_POINT('Ctrl Pts',(61.8523505660607,601.725373764374,104.870738441723));
#106006=CARTESIAN_POINT('Ctrl Pts',(61.8523505660607,601.725373764374,104.934462686335));
#106007=CARTESIAN_POINT('Ctrl Pts',(61.8523505660607,601.733555001666,104.996692081853));
#106008=CARTESIAN_POINT('Ctrl Pts',(61.8523505660607,601.75024142028,105.057367425609));
#106009=CARTESIAN_POINT('Ctrl Pts',(61.8523505660607,601.752544915752,105.065743421852));
#106010=CARTESIAN_POINT('Ctrl Pts',(61.8523505660607,601.755010572306,105.074089788599));
#106011=CARTESIAN_POINT('Ctrl Pts',(61.8523505660607,601.757639320276,105.082406355946));
#106012=CARTESIAN_POINT('Ctrl Pts',(61.8523505660607,601.779310601466,105.150967766776));
#106013=CARTESIAN_POINT('Ctrl Pts',(61.8523505660608,601.811992484867,105.215987728384));
#106014=CARTESIAN_POINT('Ctrl Pts',(61.8523505660608,601.855441859262,105.272877360388));
#106015=CARTESIAN_POINT('Ctrl Pts',(61.8523505660607,601.898891233656,105.329766992393));
#106016=CARTESIAN_POINT('Ctrl Pts',(61.8523505660607,601.953782542618,105.379045945291));
#106017=CARTESIAN_POINT('Ctrl Pts',(61.8523505660607,602.017642969564,105.41367565036));
#106018=CARTESIAN_POINT('Ctrl Pts',(61.8523505660608,602.041337088189,105.426524301381));
#106019=CARTESIAN_POINT('Ctrl Pts',(61.8523505660608,602.065992574575,105.437249174374));
#106020=CARTESIAN_POINT('Ctrl Pts',(61.8523505660608,602.091368457776,105.445633434612));
#106021=CARTESIAN_POINT('Ctrl Pts',(61.8523505660608,602.115878069975,105.453731476576));
#106022=CARTESIAN_POINT('Ctrl Pts',(61.8523505660608,602.141059071268,105.459645696455));
#106023=CARTESIAN_POINT('Ctrl Pts',(61.8523505660608,602.166680666438,105.463226524911));
#106024=CARTESIAN_POINT('Ctrl Pts',(61.8523505660608,602.186027969902,105.465930469547));
#106025=CARTESIAN_POINT('Ctrl Pts',(61.8523505660608,602.205626172223,105.467304788954));
#106026=CARTESIAN_POINT('Ctrl Pts',(61.8523505660608,602.225373764374,105.467304788954));
#106027=CARTESIAN_POINT('',(61.8523505660607,601.125373764374,105.467304788954));
#106028=CARTESIAN_POINT('Origin',(43.9028862170334,601.125373764374,0.));
#106029=CARTESIAN_POINT('',(43.9028862170334,602.225373764374,105.467304788954));
#106030=CARTESIAN_POINT('',(43.9028862170334,601.725373764374,104.870738441723));
#106031=CARTESIAN_POINT('Ctrl Pts',(43.9028862170334,602.225373764374,105.467304788954));
#106032=CARTESIAN_POINT('Ctrl Pts',(43.9028862170334,602.199366036638,105.467304788954));
#106033=CARTESIAN_POINT('Ctrl Pts',(43.9028862170334,602.173617536014,105.464919144673));
#106034=CARTESIAN_POINT('Ctrl Pts',(43.9028862170334,602.148359776795,105.460256351402));
#106035=CARTESIAN_POINT('Ctrl Pts',(43.9028862170334,602.122200630188,105.455427154493));
#106036=CARTESIAN_POINT('Ctrl Pts',(43.9028862170334,602.096568531369,105.448155596141));
#106037=CARTESIAN_POINT('Ctrl Pts',(43.9028862170334,602.071712802132,105.438618445843));
#106038=CARTESIAN_POINT('Ctrl Pts',(43.9028862170334,602.053228082178,105.431525853598));
#106039=CARTESIAN_POINT('Ctrl Pts',(43.9028862170334,602.035172629463,105.423181489599));
#106040=CARTESIAN_POINT('Ctrl Pts',(43.9028862170334,602.017642969564,105.41367565036));
#106041=CARTESIAN_POINT('Ctrl Pts',(43.9028862170334,601.953782542618,105.37904594529));
#106042=CARTESIAN_POINT('Ctrl Pts',(43.9028862170334,601.898891233656,105.329766992393));
#106043=CARTESIAN_POINT('Ctrl Pts',(43.9028862170334,601.855441859261,105.272877360388));
#106044=CARTESIAN_POINT('Ctrl Pts',(43.9028862170334,601.811992484867,105.215987728384));
#106045=CARTESIAN_POINT('Ctrl Pts',(43.9028862170334,601.779310601467,105.150967766776));
#106046=CARTESIAN_POINT('Ctrl Pts',(43.9028862170334,601.757639320276,105.082406355946));
#106047=CARTESIAN_POINT('Ctrl Pts',(43.9028862170334,601.738596787043,105.022161512427));
#106048=CARTESIAN_POINT('Ctrl Pts',(43.9028862170334,601.72810819572,104.960353720503));
#106049=CARTESIAN_POINT('Ctrl Pts',(43.9028862170334,601.725842518628,104.897043449009));
#106050=CARTESIAN_POINT('Ctrl Pts',(43.9028862170334,601.725529750681,104.888303711238));
#106051=CARTESIAN_POINT('Ctrl Pts',(43.9028862170334,601.725373764374,104.879535326884));
#106052=CARTESIAN_POINT('Ctrl Pts',(43.9028862170334,601.725373764374,104.870738441723));
#106053=CARTESIAN_POINT('',(43.9028862170334,601.725373764374,99.080638124754));
#106054=CARTESIAN_POINT('',(43.9028862170334,601.725373764374,98.8874960354436));
#106055=CARTESIAN_POINT('',(43.9028862170334,639.625373764374,99.080638124754));
#106056=CARTESIAN_POINT('',(43.9028862170334,601.125373764374,99.080638124754));
#106057=CARTESIAN_POINT('',(43.9028862170334,639.625373764374,104.870738441723));
#106058=CARTESIAN_POINT('',(43.9028862170334,639.625373764374,0.));
#106059=CARTESIAN_POINT('',(43.9028862170334,639.125373764374,105.467304788954));
#106060=CARTESIAN_POINT('Ctrl Pts',(43.9028862170334,639.625373764374,104.870738441723));
#106061=CARTESIAN_POINT('Ctrl Pts',(43.9028862170334,639.625373764374,105.015531405683));
#106062=CARTESIAN_POINT('Ctrl Pts',(43.9028862170334,639.582389805433,105.159369804922));
#106063=CARTESIAN_POINT('Ctrl Pts',(43.9028862170334,639.406718012507,105.388349047246));
#106064=CARTESIAN_POINT('Ctrl Pts',(43.9028862170334,639.270789691535,105.467304788954));
#106065=CARTESIAN_POINT('Ctrl Pts',(43.9028862170334,639.125373764374,105.467304788954));
#106066=CARTESIAN_POINT('',(43.9028862170334,602.225373764374,105.467304788954));
#106067=CARTESIAN_POINT('Origin',(52.8776183915471,639.125373764374,90.6087118617898));
#106068=CARTESIAN_POINT('Ctrl Pts',(43.1340595514603,639.125373764374,105.888887786568));
#106069=CARTESIAN_POINT('Ctrl Pts',(43.1340595514603,639.183634335595,105.888887786568));
#106070=CARTESIAN_POINT('Ctrl Pts',(43.1353749199127,639.241023457001,105.883765013252));
#106071=CARTESIAN_POINT('Ctrl Pts',(43.1379705232213,639.297646653191,105.873657394149));
#106072=CARTESIAN_POINT('Ctrl Pts',(43.1385991820447,639.311360872069,105.871209314385));
#106073=CARTESIAN_POINT('Ctrl Pts',(43.139303000641,639.325030102463,105.868468588626));
#106074=CARTESIAN_POINT('Ctrl Pts',(43.1400815900552,639.338655734907,105.865436756047));
#106075=CARTESIAN_POINT('Ctrl Pts',(43.1425184881117,639.381302445243,105.855947458114));
#106076=CARTESIAN_POINT('Ctrl Pts',(43.1457204641877,639.423585630974,105.843480262565));
#106077=CARTESIAN_POINT('Ctrl Pts',(43.149600304955,639.464673649675,105.82838734085));
#106078=CARTESIAN_POINT('Ctrl Pts',(43.1512777614199,639.482438131966,105.821861887712));
#106079=CARTESIAN_POINT('Ctrl Pts',(43.1530819274064,639.499978593913,105.814845638027));
#106080=CARTESIAN_POINT('Ctrl Pts',(43.1550057044128,639.51722471474,105.807367331575));
#106081=CARTESIAN_POINT('Ctrl Pts',(43.155836125878,639.524669210063,105.804139230719));
#106082=CARTESIAN_POINT('Ctrl Pts',(43.1566894887349,639.532063578086,105.800823057735));
#106083=CARTESIAN_POINT('Ctrl Pts',(43.1575652792992,639.539401572236,105.797420942698));
#106084=CARTESIAN_POINT('Ctrl Pts',(43.1620564698277,639.577031950051,105.779974366481));
#106085=CARTESIAN_POINT('Ctrl Pts',(43.1671922663579,639.613728245051,105.760055341059));
#106086=CARTESIAN_POINT('Ctrl Pts',(43.1729063844078,639.649034910278,105.737944045788));
#106087=CARTESIAN_POINT('Ctrl Pts',(43.1766524913453,639.672181534551,105.723448147052));
#106088=CARTESIAN_POINT('Ctrl Pts',(43.1806469908836,639.694730149313,105.708010711998));
#106089=CARTESIAN_POINT('Ctrl Pts',(43.184869232144,639.716543554195,105.69171884283));
#106090=CARTESIAN_POINT('Ctrl Pts',(43.193616403455,639.761734147912,105.657967154616));
#106091=CARTESIAN_POINT('Ctrl Pts',(43.2032702988599,639.803594208621,105.620819562242));
#106092=CARTESIAN_POINT('Ctrl Pts',(43.213825446355,639.842208965498,105.580362184908));
#106093=CARTESIAN_POINT('Ctrl Pts',(43.2158189162106,639.849501838843,105.572721309952));
#106094=CARTESIAN_POINT('Ctrl Pts',(43.2178438267247,639.856676746876,105.564964855412));
#106095=CARTESIAN_POINT('Ctrl Pts',(43.2199001658011,639.86373494426,105.557093372208));
#106096=CARTESIAN_POINT('Ctrl Pts',(43.2306831409574,639.900746528542,105.515817101766));
#106097=CARTESIAN_POINT('Ctrl Pts',(43.2422060359435,639.934106550084,105.47185885015));
#106098=CARTESIAN_POINT('Ctrl Pts',(43.2543899245646,639.963675367698,105.425575864041));
#106099=CARTESIAN_POINT('Ctrl Pts',(43.2659229308836,639.991664573032,105.381765387119));
#106100=CARTESIAN_POINT('Ctrl Pts',(43.2780483172813,640.016256574864,105.33587144162));
#106101=CARTESIAN_POINT('Ctrl Pts',(43.2906914506057,640.03730213598,105.288231896121));
#106102=CARTESIAN_POINT('Ctrl Pts',(43.294007829138,640.042822527586,105.275735724332));
#106103=CARTESIAN_POINT('Ctrl Pts',(43.2973597827178,640.048098745172,105.263119663155));
#106104=CARTESIAN_POINT('Ctrl Pts',(43.3007458539078,640.053127748537,105.250390301448));
#106105=CARTESIAN_POINT('Ctrl Pts',(43.3024790201449,640.055701852373,105.243874756236));
#106106=CARTESIAN_POINT('Ctrl Pts',(43.3042190431903,640.058208132244,105.237337246198));
#106107=CARTESIAN_POINT('Ctrl Pts',(43.3059656934663,640.060646673368,105.23077875602));
#106108=CARTESIAN_POINT('Ctrl Pts',(43.3194716366484,640.079502650615,105.180065343653));
#106109=CARTESIAN_POINT('Ctrl Pts',(43.3331997567824,640.094186237523,105.128744628145));
#106110=CARTESIAN_POINT('Ctrl Pts',(43.3471728225631,640.104775540729,105.076754341906));
#106111=CARTESIAN_POINT('Ctrl Pts',(43.3613724966737,640.115536576062,105.023920902695));
#106112=CARTESIAN_POINT('Ctrl Pts',(43.3758251265072,640.122069386147,104.970395944298));
#106113=CARTESIAN_POINT('Ctrl Pts',(43.3905572354151,640.124402582393,104.916108237801));
#106114=CARTESIAN_POINT('Ctrl Pts',(43.3946451609367,640.125050007181,104.901044264117));
#106115=CARTESIAN_POINT('Ctrl Pts',(43.3987546209328,640.125373764374,104.885921529213));
#106116=CARTESIAN_POINT('Ctrl Pts',(43.4028862170334,640.125373764374,104.870738441723));
#106117=CARTESIAN_POINT('Origin',(35.7552367830941,639.125373764374,90.6087118617898));
#106118=CARTESIAN_POINT('Origin',(35.7552367830941,639.125373764374,-5.58390168977932E-15));
#106119=CARTESIAN_POINT('Ctrl Pts',(34.7552367830941,639.125373764374,73.1199049166885));
#106120=CARTESIAN_POINT('Ctrl Pts',(34.7552367830941,639.200884802411,72.8040068203705));
#106121=CARTESIAN_POINT('Ctrl Pts',(34.7636376301548,639.271491652081,72.4878072684));
#106122=CARTESIAN_POINT('Ctrl Pts',(34.7779932599735,639.337516912742,72.1711663955806));
#106123=CARTESIAN_POINT('Ctrl Pts',(34.7798305566038,639.345967115935,72.1306413043105));
#106124=CARTESIAN_POINT('Ctrl Pts',(34.7817654544466,639.354342292342,72.090109013267));
#106125=CARTESIAN_POINT('Ctrl Pts',(34.7837928855838,639.362643134571,72.0495692558948));
#106126=CARTESIAN_POINT('Ctrl Pts',(34.8004726967557,639.43093471716,71.7160459684573));
#106127=CARTESIAN_POINT('Ctrl Pts',(34.8234784568466,639.494189531026,71.3820173166586));
#106128=CARTESIAN_POINT('Ctrl Pts',(34.851116807566,639.552654661099,71.0475114120635));
#106129=CARTESIAN_POINT('Ctrl Pts',(34.8533204597638,639.557316184273,71.0208406935639));
#106130=CARTESIAN_POINT('Ctrl Pts',(34.8555535843187,639.56194726855,70.9941669549191));
#106131=CARTESIAN_POINT('Ctrl Pts',(34.8578153353241,639.566548044146,70.967490217716));
#106132=CARTESIAN_POINT('Ctrl Pts',(34.8588927099961,639.568739602406,70.954782876843));
#106133=CARTESIAN_POINT('Ctrl Pts',(34.8599766633094,639.570924412863,70.9420737239539));
#106134=CARTESIAN_POINT('Ctrl Pts',(34.8610671285686,639.573102474715,70.9293628456683));
#106135=CARTESIAN_POINT('Ctrl Pts',(34.8816001688782,639.614114539466,70.6900219093161));
#106136=CARTESIAN_POINT('Ctrl Pts',(34.9044201141224,639.652698786736,70.4502744546756));
#106137=CARTESIAN_POINT('Ctrl Pts',(34.9291259895506,639.688922550039,70.2102707123723));
#106138=CARTESIAN_POINT('Ctrl Pts',(34.956169125434,639.728573205448,69.9475617938197));
#106139=CARTESIAN_POINT('Ctrl Pts',(34.9854722230115,639.765396145449,69.6845451902924));
#106140=CARTESIAN_POINT('Ctrl Pts',(35.0165561203898,639.799447393656,69.4213836553411));
#106141=CARTESIAN_POINT('Ctrl Pts',(35.0424690442426,639.827834033566,69.2020004572428));
#106142=CARTESIAN_POINT('Ctrl Pts',(35.0696207330031,639.85429387261,68.9825155527574));
#106143=CARTESIAN_POINT('Ctrl Pts',(35.0977513325307,639.878841004738,68.7630133520805));
#106144=CARTESIAN_POINT('Ctrl Pts',(35.0994093669033,639.880287827398,68.7500757609986));
#106145=CARTESIAN_POINT('Ctrl Pts',(35.1010708214122,639.881728095368,68.7371380738301));
#106146=CARTESIAN_POINT('Ctrl Pts',(35.1027356711041,639.883161820044,68.7242002248716));
#106147=CARTESIAN_POINT('Ctrl Pts',(35.1578246869571,639.930603028578,68.2960934895558));
#106148=CARTESIAN_POINT('Ctrl Pts',(35.2166172729909,639.970862604241,67.8679097403797));
#106149=CARTESIAN_POINT('Ctrl Pts',(35.2779103319681,640.004140516552,67.4395068625554));
#106150=CARTESIAN_POINT('Ctrl Pts',(35.3208375199838,640.027447025027,67.1394707542299));
#106151=CARTESIAN_POINT('Ctrl Pts',(35.36499069794,640.047330100565,66.8393272423455));
#106152=CARTESIAN_POINT('Ctrl Pts',(35.4099554169091,640.063872980232,66.5390317516864));
#106153=CARTESIAN_POINT('Ctrl Pts',(35.4112107944409,640.064334843664,66.5306477515076));
#106154=CARTESIAN_POINT('Ctrl Pts',(35.4124668432853,640.06479408847,66.5222635016681));
#106155=CARTESIAN_POINT('Ctrl Pts',(35.4137235541889,640.065250715059,66.5138790148404));
#106156=CARTESIAN_POINT('Ctrl Pts',(35.4873122291016,640.091989200063,66.0229122589214));
#106157=CARTESIAN_POINT('Ctrl Pts',(35.563215136994,640.109769754558,65.5307970571815));
#106158=CARTESIAN_POINT('Ctrl Pts',(35.6397290728435,640.118672316601,65.0392629090769));
#106159=CARTESIAN_POINT('Ctrl Pts',(35.6781489588635,640.123142553495,64.7924492308175));
#106160=CARTESIAN_POINT('Ctrl Pts',(35.7167231407543,640.125373764374,64.5457813055128));
#106161=CARTESIAN_POINT('Ctrl Pts',(35.7552367830941,640.125373764374,64.2994740882088));
#106162=CARTESIAN_POINT('Ctrl Pts',(33.7552367830941,638.223173275376,72.6885880057604));
#106163=CARTESIAN_POINT('Ctrl Pts',(34.7552367830941,638.223173275376,72.6885880057604));
#106164=CARTESIAN_POINT('Ctrl Pts',(34.7552367830941,639.125373764374,73.1199049166885));
#106165=CARTESIAN_POINT('Ctrl Pts',(33.7552367874537,638.384664659928,72.3507908955142));
#106166=CARTESIAN_POINT('Ctrl Pts',(34.6814263287167,638.363575572785,72.3949036703327));
#106167=CARTESIAN_POINT('Ctrl Pts',(34.7552367830941,639.210271619968,72.7647373589289));
#106168=CARTESIAN_POINT('Ctrl Pts',(33.7764837682833,638.534848672552,72.0116381428428));
#106169=CARTESIAN_POINT('Ctrl Pts',(34.6339372270254,638.50739702657,72.0748761014097));
#106170=CARTESIAN_POINT('Ctrl Pts',(34.7658602751036,639.289223684062,72.4081504335284));
#106171=CARTESIAN_POINT('Ctrl Pts',(33.8482184555667,638.814182242514,71.3295484402176));
#106172=CARTESIAN_POINT('Ctrl Pts',(34.5852404580364,638.77802067215,71.4214334883314));
#106173=CARTESIAN_POINT('Ctrl Pts',(34.8017276199155,639.436071280424,71.690991851673));
#106174=CARTESIAN_POINT('Ctrl Pts',(33.8988585801114,638.943324593884,70.9866109201948));
#106175=CARTESIAN_POINT('Ctrl Pts',(34.5812439461558,638.907206976171,71.085350352821));
#106176=CARTESIAN_POINT('Ctrl Pts',(34.8270476812808,639.503962311126,71.3304225824941));
#106177=CARTESIAN_POINT('Ctrl Pts',(34.0834772923341,639.30050117458,69.9510610361466));
#106178=CARTESIAN_POINT('Ctrl Pts',(34.6170246837339,639.258114901121,70.0851505103093));
#106179=CARTESIAN_POINT('Ctrl Pts',(34.919357038358,639.691732518317,70.2416310592042));
#106180=CARTESIAN_POINT('Ctrl Pts',(34.2506966542608,639.499087923712,69.2481994911169));
#106181=CARTESIAN_POINT('Ctrl Pts',(34.7001850449893,639.468602714415,69.3679973198037));
#106182=CARTESIAN_POINT('Ctrl Pts',(35.0029667184136,639.796130951156,69.5026326737362));
#106183=CARTESIAN_POINT('Ctrl Pts',(34.6298396352898,639.813753889154,67.841296227345));
#106184=CARTESIAN_POINT('Ctrl Pts',(34.9323200255037,639.794711368262,67.9421363496405));
#106185=CARTESIAN_POINT('Ctrl Pts',(35.1925382094558,639.961553032868,68.0233950520287));
#106186=CARTESIAN_POINT('Ctrl Pts',(34.8418678006974,639.930423294367,67.1371463181171));
#106187=CARTESIAN_POINT('Ctrl Pts',(35.0803796729177,639.919899379557,67.2146858539356));
#106188=CARTESIAN_POINT('Ctrl Pts',(35.2985522918458,640.022886949265,67.2830420625807));
#106189=CARTESIAN_POINT('Ctrl Pts',(35.2874823657224,640.086351313611,65.7218898747875));
#106190=CARTESIAN_POINT('Ctrl Pts',(35.4025374070644,640.083346941915,65.7667284931679));
#106191=CARTESIAN_POINT('Ctrl Pts',(35.5213595744583,640.104859391058,65.79502179184));
#106192=CARTESIAN_POINT('Ctrl Pts',(35.5216787611567,640.125373764374,65.0097934141342));
#106193=CARTESIAN_POINT('Ctrl Pts',(35.5800722057109,640.125373764374,65.0280371672288));
#106194=CARTESIAN_POINT('Ctrl Pts',(35.6384569650295,640.125373764374,65.0463188496307));
#106195=CARTESIAN_POINT('Ctrl Pts',(35.7552367830941,640.125373764374,64.2994740882088));
#106196=CARTESIAN_POINT('Ctrl Pts',(35.7552367830941,640.125373764374,64.2994740882088));
#106197=CARTESIAN_POINT('Ctrl Pts',(35.7552367830941,640.125373764374,64.2994740882088));
#106198=CARTESIAN_POINT('Origin',(33.7552367830941,639.125373764374,73.1199049166885));
#106199=CARTESIAN_POINT('Origin',(33.7552367830941,620.675373764374,64.2994740882088));
#106200=CARTESIAN_POINT('Origin',(33.7552367830941,602.225373764374,73.1199049166887));
#106201=CARTESIAN_POINT('Ctrl Pts',(34.7552367830941,602.225373764374,73.1199049166888));
#106202=CARTESIAN_POINT('Ctrl Pts',(34.7552367830941,603.127574253371,72.6885880057606));
#106203=CARTESIAN_POINT('Ctrl Pts',(33.7552367830941,603.127574253371,72.6885880057606));
#106204=CARTESIAN_POINT('Ctrl Pts',(34.7552367830941,602.140475908865,72.764737358909));
#106205=CARTESIAN_POINT('Ctrl Pts',(34.6814263286416,602.98717195596,72.3949036703512));
#106206=CARTESIAN_POINT('Ctrl Pts',(33.7552367874592,602.966082868819,72.3507908955145));
#106207=CARTESIAN_POINT('Ctrl Pts',(34.7658602751036,602.061523844686,72.4081504335286));
#106208=CARTESIAN_POINT('Ctrl Pts',(34.6339372270254,602.843350502178,72.0748761014127));
#106209=CARTESIAN_POINT('Ctrl Pts',(33.7764837682833,602.815898856196,72.011638142843));
#106210=CARTESIAN_POINT('Ctrl Pts',(34.8017276199155,601.914676248324,71.6909918516732));
#106211=CARTESIAN_POINT('Ctrl Pts',(34.5852404580363,602.572726856598,71.4214334883289));
#106212=CARTESIAN_POINT('Ctrl Pts',(33.8482184555667,602.536565286233,71.3295484402178));
#106213=CARTESIAN_POINT('Ctrl Pts',(34.8270476812803,601.846785217622,71.3304225825078));
#106214=CARTESIAN_POINT('Ctrl Pts',(34.5812439461531,602.443540552576,71.0853503528376));
#106215=CARTESIAN_POINT('Ctrl Pts',(33.8988585801101,602.407422934868,70.9866109202095));
#106216=CARTESIAN_POINT('Ctrl Pts',(34.919357038359,601.659015010429,70.2416310591774));
#106217=CARTESIAN_POINT('Ctrl Pts',(34.6170246837392,602.092632627626,70.0851505102782));
#106218=CARTESIAN_POINT('Ctrl Pts',(34.0834772923369,602.050246354158,69.9510610361178));
#106219=CARTESIAN_POINT('Ctrl Pts',(35.0029667184137,601.554616577592,69.5026326737309));
#106220=CARTESIAN_POINT('Ctrl Pts',(34.7001850449893,601.882144814288,69.3679973197988));
#106221=CARTESIAN_POINT('Ctrl Pts',(34.2506966542582,601.851659605033,69.2481994911067));
#106222=CARTESIAN_POINT('Ctrl Pts',(35.1925382094559,601.38919449588,68.0233950520342));
#106223=CARTESIAN_POINT('Ctrl Pts',(34.9323200255037,601.556036160528,67.9421363496463));
#106224=CARTESIAN_POINT('Ctrl Pts',(34.6298396352926,601.536993639596,67.8412962273554));
#106225=CARTESIAN_POINT('Ctrl Pts',(35.2985522918459,601.327860579483,67.2830420625863));
#106226=CARTESIAN_POINT('Ctrl Pts',(35.0803796729178,601.43084814919,67.2146858539412));
#106227=CARTESIAN_POINT('Ctrl Pts',(34.8418678006976,601.420324234381,67.1371463181226));
#106228=CARTESIAN_POINT('Ctrl Pts',(35.5213595744584,601.24588813769,65.7950217918347));
#106229=CARTESIAN_POINT('Ctrl Pts',(35.4025374070644,601.267400586833,65.7667284931627));
#106230=CARTESIAN_POINT('Ctrl Pts',(35.2874823657227,601.264396215136,65.7218898747823));
#106231=CARTESIAN_POINT('Ctrl Pts',(35.6384569653697,601.225373764374,65.0463188496885));
#106232=CARTESIAN_POINT('Ctrl Pts',(35.580072206224,601.225373764374,65.0280371673566));
#106233=CARTESIAN_POINT('Ctrl Pts',(35.5216787617927,601.225373764374,65.0097934143472));
#106234=CARTESIAN_POINT('Ctrl Pts',(35.7552367830941,601.225373764374,64.2994740882088));
#106235=CARTESIAN_POINT('Ctrl Pts',(35.7552367830941,601.225373764374,64.2994740882088));
#106236=CARTESIAN_POINT('Ctrl Pts',(35.7552367830941,601.225373764374,64.2994740882088));
#106237=CARTESIAN_POINT('Ctrl Pts',(34.7552367830941,602.225373764374,73.1199049166888));
#106238=CARTESIAN_POINT('Ctrl Pts',(34.7552367830941,602.149862727759,72.8040068259897));
#106239=CARTESIAN_POINT('Ctrl Pts',(34.7636376298549,602.079255879206,72.4878072796902));
#106240=CARTESIAN_POINT('Ctrl Pts',(34.7779932592036,602.013230619549,72.1711664125558));
#106241=CARTESIAN_POINT('Ctrl Pts',(34.7798305560632,602.004780415154,72.1306413156293));
#106242=CARTESIAN_POINT('Ctrl Pts',(34.7817654541633,601.996405237566,72.0901090189274));
#106243=CARTESIAN_POINT('Ctrl Pts',(34.7837928855835,601.988104394178,72.0495692558945));
#106244=CARTESIAN_POINT('Ctrl Pts',(34.8004726966809,601.919812811894,71.7160459699422));
#106245=CARTESIAN_POINT('Ctrl Pts',(34.8234784566402,601.85655799829,71.3820173196514));
#106246=CARTESIAN_POINT('Ctrl Pts',(34.8511168071947,601.798092868435,71.0475114165508));
#106247=CARTESIAN_POINT('Ctrl Pts',(34.8533204595128,601.793431344995,71.0208406965558));
#106248=CARTESIAN_POINT('Ctrl Pts',(34.8555535841913,601.788800260457,70.9941669564151));
#106249=CARTESIAN_POINT('Ctrl Pts',(34.8578153353235,601.784199484603,70.9674902177157));
#106250=CARTESIAN_POINT('Ctrl Pts',(34.8588927099955,601.782007926342,70.9547828768427));
#106251=CARTESIAN_POINT('Ctrl Pts',(34.8599766633088,601.779823115886,70.9420737239535));
#106252=CARTESIAN_POINT('Ctrl Pts',(34.861067128568,601.777645054033,70.9293628456679));
#106253=CARTESIAN_POINT('Ctrl Pts',(34.8816001689142,601.73663298921,70.6900219088858));
#106254=CARTESIAN_POINT('Ctrl Pts',(34.9044201142034,601.698048741874,70.4502744538141));
#106255=CARTESIAN_POINT('Ctrl Pts',(34.9291259896828,601.661824978515,70.210270711079));
#106256=CARTESIAN_POINT('Ctrl Pts',(34.9561691256169,601.622174323051,69.9475617921052));
#106257=CARTESIAN_POINT('Ctrl Pts',(34.9854722232518,601.585351383005,69.6845451881559));
#106258=CARTESIAN_POINT('Ctrl Pts',(35.0165561206916,601.551300134761,69.4213836527824));
#106259=CARTESIAN_POINT('Ctrl Pts',(35.0424690444536,601.522913494976,69.2020004555364));
#106260=CARTESIAN_POINT('Ctrl Pts',(35.0696207331126,601.496453656042,68.9825155519043));
#106261=CARTESIAN_POINT('Ctrl Pts',(35.097751332531,601.471906524009,68.7630133520807));
#106262=CARTESIAN_POINT('Ctrl Pts',(35.0994093669035,601.47045970135,68.7500757609988));
#106263=CARTESIAN_POINT('Ctrl Pts',(35.1010708214125,601.46901943338,68.7371380738303));
#106264=CARTESIAN_POINT('Ctrl Pts',(35.1027356711043,601.467585708703,68.7242002248718));
#106265=CARTESIAN_POINT('Ctrl Pts',(35.1578246853299,601.420144501571,68.296093502205));
#106266=CARTESIAN_POINT('Ctrl Pts',(35.2166172695204,601.379884926883,67.8679097656832));
#106267=CARTESIAN_POINT('Ctrl Pts',(35.2779103265398,601.346607015144,67.4395069005296));
#106268=CARTESIAN_POINT('Ctrl Pts',(35.3208375162637,601.323300505397,67.1394707795558));
#106269=CARTESIAN_POINT('Ctrl Pts',(35.364990696048,601.303417428879,66.8393272550155));
#106270=CARTESIAN_POINT('Ctrl Pts',(35.4099554169122,601.286874548515,66.5390317516875));
#106271=CARTESIAN_POINT('Ctrl Pts',(35.411210794444,601.286412685082,66.5306477515087));
#106272=CARTESIAN_POINT('Ctrl Pts',(35.4124668432884,601.285953440277,66.5222635016692));
#106273=CARTESIAN_POINT('Ctrl Pts',(35.413723554192,601.285496813687,66.5138790148415));
#106274=CARTESIAN_POINT('Ctrl Pts',(35.4873122167619,601.258758333171,66.0229123412839));
#106275=CARTESIAN_POINT('Ctrl Pts',(35.5632151116575,601.24097778016,65.5307972223043));
#106276=CARTESIAN_POINT('Ctrl Pts',(35.6397290344742,601.232075216629,65.0392631564647));
#106277=CARTESIAN_POINT('Ctrl Pts',(35.6781489332305,601.227604976743,64.7924493956532));
#106278=CARTESIAN_POINT('Ctrl Pts',(35.716723128,601.225373764374,64.5457813878173));
#106279=CARTESIAN_POINT('Ctrl Pts',(35.7552367830941,601.225373764374,64.2994740882088));
#106280=CARTESIAN_POINT('Origin',(52.8776183915471,602.225373764374,90.6087118617898));
#106281=CARTESIAN_POINT('Ctrl Pts',(43.4028862170334,601.225373764374,104.870738441723));
#106282=CARTESIAN_POINT('Ctrl Pts',(43.3929635135731,601.225373764374,104.907203108541));
#106283=CARTESIAN_POINT('Ctrl Pts',(43.3830997768354,601.227246441777,104.943571896842));
#106284=CARTESIAN_POINT('Ctrl Pts',(43.3733309369751,601.231039696142,104.979707661265));
#106285=CARTESIAN_POINT('Ctrl Pts',(43.3636271064666,601.234807707283,105.015602950601));
#106286=CARTESIAN_POINT('Ctrl Pts',(43.3540169147645,601.24047088985,105.051268273045));
#106287=CARTESIAN_POINT('Ctrl Pts',(43.3445328457605,601.248025482688,105.086576105327));
#106288=CARTESIAN_POINT('Ctrl Pts',(43.3350946628853,601.25554352465,105.121713110115));
#106289=CARTESIAN_POINT('Ctrl Pts',(43.3257813836885,601.264934744555,105.156496049068));
#106290=CARTESIAN_POINT('Ctrl Pts',(43.3166223112608,601.276144301285,105.190806555502));
#106291=CARTESIAN_POINT('Ctrl Pts',(43.3130932278474,601.280463457078,105.204026741293));
#106292=CARTESIAN_POINT('Ctrl Pts',(43.3095870100482,601.285052028013,105.217176867284));
#106293=CARTESIAN_POINT('Ctrl Pts',(43.3061052272023,601.28990483431,105.23025046543));
#106294=CARTESIAN_POINT('Ctrl Pts',(43.304133024549,601.292653632233,105.237655805192));
#106295=CARTESIAN_POINT('Ctrl Pts',(43.3021714197628,601.295486654525,105.245026401512));
#106296=CARTESIAN_POINT('Ctrl Pts',(43.3002211472687,601.298402436799,105.252359276489));
#106297=CARTESIAN_POINT('Ctrl Pts',(43.2895700950561,601.314326441949,105.292406415793));
#106298=CARTESIAN_POINT('Ctrl Pts',(43.2792549047321,601.332717916753,105.33133652796));
#106299=CARTESIAN_POINT('Ctrl Pts',(43.2693167278587,601.353472222818,105.368963065964));
#106300=CARTESIAN_POINT('Ctrl Pts',(43.259184556759,601.374631655054,105.407324077827));
#106301=CARTESIAN_POINT('Ctrl Pts',(43.2494440091227,601.398247078674,105.444331157281));
#106302=CARTESIAN_POINT('Ctrl Pts',(43.2401379297371,601.424261011787,105.479794260594));
#106303=CARTESIAN_POINT('Ctrl Pts',(43.2332977787152,601.443381763264,105.505860337652));
#106304=CARTESIAN_POINT('Ctrl Pts',(43.2266923194162,601.46379943899,105.531092498743));
#106305=CARTESIAN_POINT('Ctrl Pts',(43.2203395080143,601.485508985179,105.555412940236));
#106306=CARTESIAN_POINT('Ctrl Pts',(43.2180660612489,601.493278064795,105.564116367042));
#106307=CARTESIAN_POINT('Ctrl Pts',(43.2158231146049,601.501223507163,105.572710082201));
#106308=CARTESIAN_POINT('Ctrl Pts',(43.2136122722059,601.509342317478,105.581187290618));
#106309=CARTESIAN_POINT('Ctrl Pts',(43.2064137894534,601.535777090056,105.608789004159));
#106310=CARTESIAN_POINT('Ctrl Pts',(43.1996287034623,601.563766590648,105.634860742575));
#106311=CARTESIAN_POINT('Ctrl Pts',(43.1932901049922,601.593131983422,105.659265244783));
#106312=CARTESIAN_POINT('Ctrl Pts',(43.1895319638322,601.610542660528,105.67373462073));
#106313=CARTESIAN_POINT('Ctrl Pts',(43.185930708089,601.628438044517,105.687618274192));
#106314=CARTESIAN_POINT('Ctrl Pts',(43.1824929871301,601.646789202091,105.700889266621));
#106315=CARTESIAN_POINT('Ctrl Pts',(43.1777050796575,601.672347892144,105.719372524738));
#106316=CARTESIAN_POINT('Ctrl Pts',(43.1732335162674,601.698788718341,105.736663826652));
#106317=CARTESIAN_POINT('Ctrl Pts',(43.1690998968992,601.726006943104,105.752668960234));
#106318=CARTESIAN_POINT('Ctrl Pts',(43.1665477254134,601.742811968179,105.76255081967));
#106319=CARTESIAN_POINT('Ctrl Pts',(43.1641243233116,601.759913496151,105.771942622967));
#106320=CARTESIAN_POINT('Ctrl Pts',(43.1618342559007,601.777288313322,105.780824375912));
#106321=CARTESIAN_POINT('Ctrl Pts',(43.1604152202763,601.788054583525,105.786327936101));
#106322=CARTESIAN_POINT('Ctrl Pts',(43.1590471800471,601.798926909346,105.791636433213));
#106323=CARTESIAN_POINT('Ctrl Pts',(43.157729864875,601.809912196874,105.796750406581));
#106324=CARTESIAN_POINT('Ctrl Pts',(43.1548317951143,601.83407963248,105.808001056302));
#106325=CARTESIAN_POINT('Ctrl Pts',(43.1521935219777,601.85861883404,105.818251934007));
#106326=CARTESIAN_POINT('Ctrl Pts',(43.1498084920379,601.88360920051,105.827525146265));
#106327=CARTESIAN_POINT('Ctrl Pts',(43.1459272965156,601.924276404232,105.842615585714));
#106328=CARTESIAN_POINT('Ctrl Pts',(43.1427359349044,601.965977548306,105.855042406237));
#106329=CARTESIAN_POINT('Ctrl Pts',(43.1402686261021,602.008411386523,105.864658408952));
#106330=CARTESIAN_POINT('Ctrl Pts',(43.1378679784102,602.049698758287,105.874014608995));
#106331=CARTESIAN_POINT('Ctrl Pts',(43.1361528128068,602.091679257314,105.880709694516));
#106332=CARTESIAN_POINT('Ctrl Pts',(43.1351426655521,602.134070837637,105.884655190318));
#106333=CARTESIAN_POINT('Ctrl Pts',(43.1344216259734,602.164329799462,105.887471471427));
#106334=CARTESIAN_POINT('Ctrl Pts',(43.1340595514603,602.194798103695,105.888887786568));
#106335=CARTESIAN_POINT('Ctrl Pts',(43.1340595514603,602.225373764374,105.888887786568));
#106336=CARTESIAN_POINT('Origin',(35.7552367830941,602.225373764374,90.6087118617898));
#106337=CARTESIAN_POINT('Origin',(35.7552367830941,602.225373764374,64.2994740882088));
#106338=CARTESIAN_POINT('Origin',(52.8776183915471,639.125373764374,90.6087118617898));
#106339=CARTESIAN_POINT('Ctrl Pts',(62.3523505660607,640.125373764374,104.870738441723));
#106340=CARTESIAN_POINT('Ctrl Pts',(62.3672566615477,640.125373764374,104.925516437054));
#106341=CARTESIAN_POINT('Ctrl Pts',(62.3818748211232,640.12116355199,104.979509244738));
#106342=CARTESIAN_POINT('Ctrl Pts',(62.3962323728286,640.112728812014,105.032789790483));
#106343=CARTESIAN_POINT('Ctrl Pts',(62.4103590117932,640.104429728099,105.085213424333));
#106344=CARTESIAN_POINT('Ctrl Pts',(62.4242333587675,640.092040971772,105.136947576151));
#106345=CARTESIAN_POINT('Ctrl Pts',(62.4378789602574,640.075498690852,105.18805636452));
#106346=CARTESIAN_POINT('Ctrl Pts',(62.4416940728365,640.07087370865,105.202345641658));
#106347=CARTESIAN_POINT('Ctrl Pts',(62.445491289658,640.065923744451,105.216586000138));
#106348=CARTESIAN_POINT('Ctrl Pts',(62.4492710896279,640.060646673367,105.23077875602));
#106349=CARTESIAN_POINT('Ctrl Pts',(62.4510177399038,640.058208132244,105.237337246198));
#106350=CARTESIAN_POINT('Ctrl Pts',(62.4527577629492,640.055701852373,105.243874756236));
#106351=CARTESIAN_POINT('Ctrl Pts',(62.4544909291863,640.053127748537,105.250390301448));
#106352=CARTESIAN_POINT('Ctrl Pts',(62.4673673952944,640.034003581395,105.29879719705));
#106353=CARTESIAN_POINT('Ctrl Pts',(62.4797497248421,640.01130676641,105.34556227519));
#106354=CARTESIAN_POINT('Ctrl Pts',(62.4915614193837,639.985193361949,105.390339388072));
#106355=CARTESIAN_POINT('Ctrl Pts',(62.5040208719223,639.957647888065,105.437572095522));
#106356=CARTESIAN_POINT('Ctrl Pts',(62.5158455201389,639.926301077701,105.482593345719));
#106357=CARTESIAN_POINT('Ctrl Pts',(62.5269553724346,639.891300137618,105.525040935468));
#106358=CARTESIAN_POINT('Ctrl Pts',(62.5297962366821,639.882350160907,105.535895070779));
#106359=CARTESIAN_POINT('Ctrl Pts',(62.5325904047578,639.873161069724,105.546581114723));
#106360=CARTESIAN_POINT('Ctrl Pts',(62.5353366172931,639.86373494426,105.557093372208));
#106361=CARTESIAN_POINT('Ctrl Pts',(62.5373929563694,639.856676746876,105.564964855412));
#106362=CARTESIAN_POINT('Ctrl Pts',(62.5394178668836,639.849501838843,105.572721309952));
#106363=CARTESIAN_POINT('Ctrl Pts',(62.5414113367392,639.842208965498,105.580362184908));
#106364=CARTESIAN_POINT('Ctrl Pts',(62.5519664842342,639.803594208621,105.620819562242));
#106365=CARTESIAN_POINT('Ctrl Pts',(62.5616203796391,639.761734147913,105.657967154616));
#106366=CARTESIAN_POINT('Ctrl Pts',(62.5703675509501,639.716543554195,105.69171884283));
#106367=CARTESIAN_POINT('Ctrl Pts',(62.5768079397057,639.683270512969,105.716569618644));
#106368=CARTESIAN_POINT('Ctrl Pts',(62.5827180384413,639.648288685124,105.739430714702));
#106369=CARTESIAN_POINT('Ctrl Pts',(62.588026029441,639.612078409095,105.759999089233));
#106370=CARTESIAN_POINT('Ctrl Pts',(62.5915058843782,639.588339388471,105.773483467722));
#106371=CARTESIAN_POINT('Ctrl Pts',(62.594727133404,639.564071594478,105.785983177564));
#106372=CARTESIAN_POINT('Ctrl Pts',(62.5976715037949,639.539401572236,105.797420942698));
#106373=CARTESIAN_POINT('Ctrl Pts',(62.5985472943592,639.532063578086,105.800823057735));
#106374=CARTESIAN_POINT('Ctrl Pts',(62.599400657216,639.524669210063,105.804139230719));
#106375=CARTESIAN_POINT('Ctrl Pts',(62.6002310786813,639.51722471474,105.807367331575));
#106376=CARTESIAN_POINT('Ctrl Pts',(62.6046806418219,639.477335630251,105.824664137095));
#106377=CARTESIAN_POINT('Ctrl Pts',(62.6084902505575,639.435875719075,105.839488697653));
#106378=CARTESIAN_POINT('Ctrl Pts',(62.6115724087117,639.393699090601,105.851487144451));
#106379=CARTESIAN_POINT('Ctrl Pts',(62.6129049855962,639.375463945823,105.856674695529));
#106380=CARTESIAN_POINT('Ctrl Pts',(62.6141015955733,639.357094120464,105.861334040209));
#106381=CARTESIAN_POINT('Ctrl Pts',(62.615155193039,639.338655734907,105.865436756047));
#106382=CARTESIAN_POINT('Ctrl Pts',(62.6183698289984,639.282398293922,105.877954570768));
#106383=CARTESIAN_POINT('Ctrl Pts',(62.6203108230594,639.225398602282,105.885513606456));
#106384=CARTESIAN_POINT('Ctrl Pts',(62.6209461358816,639.167554174569,105.887987792193));
#106385=CARTESIAN_POINT('Ctrl Pts',(62.6211000095532,639.153544171681,105.888587043507));
#106386=CARTESIAN_POINT('Ctrl Pts',(62.6211772316339,639.139484557814,105.888887786568));
#106387=CARTESIAN_POINT('Ctrl Pts',(62.6211772316339,639.125373764374,105.888887786568));
#106388=CARTESIAN_POINT('Origin',(70.,639.125373764374,90.6087118617898));
#106389=CARTESIAN_POINT('Origin',(70.,639.125373764374,0.));
#106390=CARTESIAN_POINT('Origin',(70.,602.225373764374,64.2994740882088));
#106391=CARTESIAN_POINT('Origin',(70.,602.225373764374,90.6087118617898));
#106392=CARTESIAN_POINT('Origin',(52.8776183915471,602.225373764374,90.6087118617898));
#106393=CARTESIAN_POINT('Ctrl Pts',(62.6211772316338,602.225373764374,105.888887786568));
#106394=CARTESIAN_POINT('Ctrl Pts',(62.6211772316338,602.089770025929,105.888887786568));
#106395=CARTESIAN_POINT('Ctrl Pts',(62.6140693717759,601.957352722376,105.861084706529));
#106396=CARTESIAN_POINT('Ctrl Pts',(62.5864687826938,601.710190425818,105.753868890961));
#106397=CARTESIAN_POINT('Ctrl Pts',(62.5663210244106,601.599765986676,105.675841090715));
#106398=CARTESIAN_POINT('Ctrl Pts',(62.5166193069308,601.417736746075,105.485314668297));
#106399=CARTESIAN_POINT('Ctrl Pts',(62.4870014923168,601.346042473617,105.372610356784));
#106400=CARTESIAN_POINT('Ctrl Pts',(62.4224093356835,601.249834603749,105.129772481131));
#106401=CARTESIAN_POINT('Ctrl Pts',(62.3879065652659,601.225373764374,105.001402189963));
#106402=CARTESIAN_POINT('Ctrl Pts',(62.3523505660608,601.225373764374,104.870738441723));
#106403=CARTESIAN_POINT('Ctrl Pts',(43.9028862170334,601.725373764374,104.870738441723));
#106404=CARTESIAN_POINT('Ctrl Pts',(43.9028862170334,601.225373764374,104.870738441723));
#106405=CARTESIAN_POINT('Ctrl Pts',(43.4028862170334,601.225373764374,104.870738441723));
#106406=CARTESIAN_POINT('Ctrl Pts',(43.9028862170334,601.72537378749,104.943235299706));
#106407=CARTESIAN_POINT('Ctrl Pts',(43.9028862170334,601.190801415598,104.997787302213));
#106408=CARTESIAN_POINT('Ctrl Pts',(43.3694713913988,601.225373764374,104.993533654581));
#106409=CARTESIAN_POINT('Ctrl Pts',(43.9028862170334,601.73596803839,105.013844943794));
#106410=CARTESIAN_POINT('Ctrl Pts',(43.9028862170334,601.173966762123,105.128551144522));
#106411=CARTESIAN_POINT('Ctrl Pts',(43.3372020726836,601.246562349658,105.113484360187));
#106412=CARTESIAN_POINT('Ctrl Pts',(43.9028862170334,601.779310621476,105.150967761993));
#106413=CARTESIAN_POINT('Ctrl Pts',(43.9028862170334,601.181604534533,105.413925765979));
#106414=CARTESIAN_POINT('Ctrl Pts',(43.2750077312619,601.333247441326,105.347016531996));
#106415=CARTESIAN_POINT('Ctrl Pts',(43.9028862170334,601.811992484093,105.215987727826));
#106416=CARTESIAN_POINT('Ctrl Pts',(43.9028862170332,601.21008627854,105.567638910342));
#106417=CARTESIAN_POINT('Ctrl Pts',(43.2457683931895,601.398611244944,105.45806492406));
#106418=CARTESIAN_POINT('Ctrl Pts',(43.9028862170334,601.898891258024,105.32976697493));
#106419=CARTESIAN_POINT('Ctrl Pts',(43.9028862170337,601.340706749462,105.880668070497));
#106420=CARTESIAN_POINT('Ctrl Pts',(43.194904253426,601.572408710543,105.652759440274));
#106421=CARTESIAN_POINT('Ctrl Pts',(43.9028862170334,601.953782539583,105.379045943916));
#106422=CARTESIAN_POINT('Ctrl Pts',(43.9028862170334,601.450221684901,106.040501254842));
#106423=CARTESIAN_POINT('Ctrl Pts',(43.1730456780328,601.68219134858,105.737292607677));
#106424=CARTESIAN_POINT('Ctrl Pts',(43.9028862170334,602.081503421665,105.448305316015));
#106425=CARTESIAN_POINT('Ctrl Pts',(43.9028862170334,601.779838730324,106.297756031046));
#106426=CARTESIAN_POINT('Ctrl Pts',(43.1424140517172,601.937633045168,105.856208205485));
#106427=CARTESIAN_POINT('Ctrl Pts',(43.9028862170334,602.151908862397,105.467304770256));
#106428=CARTESIAN_POINT('Ctrl Pts',(43.9028862170334,601.99123573158,106.379137803783));
#106429=CARTESIAN_POINT('Ctrl Pts',(43.1340595427293,602.078443985827,105.888887781));
#106430=CARTESIAN_POINT('Ctrl Pts',(43.9028862170334,602.225373764374,105.467304788954));
#106431=CARTESIAN_POINT('Ctrl Pts',(43.9028862170334,602.225373764374,106.379137891718));
#106432=CARTESIAN_POINT('Ctrl Pts',(43.1340595514603,602.225373764374,105.888887786568));
#106433=CARTESIAN_POINT('Origin',(43.4028862170334,602.225373764374,105.467304788954));
#106434=CARTESIAN_POINT('Origin',(43.4028862170334,601.725373764374,104.870738441723));
#106435=CARTESIAN_POINT('Origin',(43.4028862170334,601.725373764374,0.));
#106436=CARTESIAN_POINT('Origin',(43.4028862170334,601.725373764374,99.080638124754));
#106437=CARTESIAN_POINT('Origin',(43.4028862170334,601.225373764374,105.467304788954));
#106438=CARTESIAN_POINT('Origin',(43.4028862170334,639.125373764374,105.467304788954));
#106439=CARTESIAN_POINT('Origin',(43.4028862170334,601.725373764374,99.080638124754));
#106440=CARTESIAN_POINT('Origin',(43.4028862170334,601.725373764374,99.080638124754));
#106441=CARTESIAN_POINT('Ctrl Pts',(43.9028849796099,639.036778038132,105.45715096646));
#106442=CARTESIAN_POINT('Ctrl Pts',(43.9048962221699,638.846637779719,106.341172765461));
#106443=CARTESIAN_POINT('Ctrl Pts',(43.1380480521351,638.94771437284,105.873295625316));
#106444=CARTESIAN_POINT('Ctrl Pts',(43.9028849698754,639.104429949246,105.470819015702));
#106445=CARTESIAN_POINT('Ctrl Pts',(43.9049389572813,639.057960777493,106.401099978679));
#106446=CARTESIAN_POINT('Ctrl Pts',(43.1320188140359,639.083373273735,105.896877360038));
#106447=CARTESIAN_POINT('Ctrl Pts',(43.9028849713453,639.169333962302,105.468738411503));
#106448=CARTESIAN_POINT('Ctrl Pts',(43.9049320498006,639.266412765078,106.390924409249));
#106449=CARTESIAN_POINT('Ctrl Pts',(43.1329294306683,639.213530456068,105.893276648178));
#106450=CARTESIAN_POINT('Ctrl Pts',(43.9028849892889,639.266404183712,105.443607670973));
#106451=CARTESIAN_POINT('Ctrl Pts',(43.9048555577325,639.560609042325,106.285968855676));
#106452=CARTESIAN_POINT('Ctrl Pts',(43.1440423040929,639.40816781027,105.84996254853));
#106453=CARTESIAN_POINT('Ctrl Pts',(43.902884998944,639.300380640497,105.430093200578));
#106454=CARTESIAN_POINT('Ctrl Pts',(43.9048160471508,639.656569714094,106.231993523399));
#106455=CARTESIAN_POINT('Ctrl Pts',(43.1500216005741,639.476286250348,105.826675971902));
#106456=CARTESIAN_POINT('Ctrl Pts',(43.9028850232857,639.363350391771,105.396101801474));
#106457=CARTESIAN_POINT('Ctrl Pts',(43.904722123573,639.819653222097,106.105164437961));
#106458=CARTESIAN_POINT('Ctrl Pts',(43.1650945293205,639.602513033697,105.768158764631));
#106459=CARTESIAN_POINT('Ctrl Pts',(43.9028850382186,639.393109422988,105.375281527712));
#106460=CARTESIAN_POINT('Ctrl Pts',(43.9046677648458,639.888724247457,106.032369901576));
#106461=CARTESIAN_POINT('Ctrl Pts',(43.1743404473524,639.662155988573,105.732338549014));
#106462=CARTESIAN_POINT('Ctrl Pts',(43.9028850722291,639.447392783658,105.328007499781));
#106463=CARTESIAN_POINT('Ctrl Pts',(43.9045527207096,640.00043915945,105.879788807098));
#106464=CARTESIAN_POINT('Ctrl Pts',(43.1953957620866,639.770930402132,105.651098312915));
#106465=CARTESIAN_POINT('Ctrl Pts',(43.9028850911418,639.471794258301,105.301782188552));
#106466=CARTESIAN_POINT('Ctrl Pts',(43.9044931551193,640.043577922308,105.801414716341));
#106467=CARTESIAN_POINT('Ctrl Pts',(43.2071028495104,639.819816105116,105.606071364224));
#106468=CARTESIAN_POINT('Ctrl Pts',(43.9028851531601,639.537574714346,105.216089189308));
#106469=CARTESIAN_POINT('Ctrl Pts',(43.9043159644082,640.14086522548,105.569416826768));
#106470=CARTESIAN_POINT('Ctrl Pts',(43.2454862343439,639.951569950465,105.459135338167));
#106471=CARTESIAN_POINT('Ctrl Pts',(43.9028852004078,639.570271688884,105.151191462665));
#106472=CARTESIAN_POINT('Ctrl Pts',(43.9041973830617,640.169349769983,105.41549399436));
#106473=CARTESIAN_POINT('Ctrl Pts',(43.2747212509798,640.01702622273,105.348095923453));
#106474=CARTESIAN_POINT('Ctrl Pts',(43.9028853216263,639.622599458369,104.986125028804));
#106475=CARTESIAN_POINT('Ctrl Pts',(43.9039388064658,640.178380909355,105.076238171418));
#106476=CARTESIAN_POINT('Ctrl Pts',(43.3497043955024,640.121714641666,105.066534511823));
#106477=CARTESIAN_POINT('Ctrl Pts',(43.9028853957751,639.631100186342,104.886222171346));
#106478=CARTESIAN_POINT('Ctrl Pts',(43.9038057069545,640.143976851776,104.898778370354));
#106479=CARTESIAN_POINT('Ctrl Pts',(43.3955564977506,640.138657441274,104.896768194163));
#106480=CARTESIAN_POINT('Ctrl Pts',(43.9028854731814,639.619496306592,104.783210498779));
#106481=CARTESIAN_POINT('Ctrl Pts',(43.9036820200741,640.078232214502,104.726934492466));
#106482=CARTESIAN_POINT('Ctrl Pts',(43.4434121618144,640.115332282487,104.722478050627));
#106483=CARTESIAN_POINT('Origin',(43.4028862170334,639.625373764374,104.870738441723));
#106484=CARTESIAN_POINT('Origin',(43.4028862170334,601.125373764374,99.080638124754));
#106485=CARTESIAN_POINT('Origin',(43.4028862170334,639.625373764374,99.080638124754));
#106486=CARTESIAN_POINT('Origin',(43.4028862170334,639.625373764374,0.));
#106487=CARTESIAN_POINT('Origin',(43.4028862170334,639.625373764374,99.080638124754));
#106488=CARTESIAN_POINT('Origin',(62.3523505660608,601.725373764374,0.));
#106489=CARTESIAN_POINT('Origin',(62.3523505660608,601.725373764374,99.080638124754));
#106490=CARTESIAN_POINT('Origin',(62.3523505660608,601.725373764374,104.870738441723));
#106491=CARTESIAN_POINT('Origin',(62.3523505660608,601.725373764374,99.080638124754));
#106492=CARTESIAN_POINT('Origin',(62.3523505660608,601.725373764374,99.080638124754));
#106493=CARTESIAN_POINT('Origin',(43.4028862170334,639.625373764374,99.080638124754));
#106494=CARTESIAN_POINT('Ctrl Pts',(62.3523505660608,601.225373764374,104.870738441723));
#106495=CARTESIAN_POINT('Ctrl Pts',(61.8523505660607,601.225373764374,104.870738441723));
#106496=CARTESIAN_POINT('Ctrl Pts',(61.8523505660607,601.725373764374,104.870738441723));
#106497=CARTESIAN_POINT('Ctrl Pts',(62.3857653916954,601.225373764374,104.993533654581));
#106498=CARTESIAN_POINT('Ctrl Pts',(61.8523505660607,601.190801415598,104.997787302213));
#106499=CARTESIAN_POINT('Ctrl Pts',(61.8523505660607,601.72537378749,104.943235299706));
#106500=CARTESIAN_POINT('Ctrl Pts',(62.4180347104105,601.246562349658,105.113484360187));
#106501=CARTESIAN_POINT('Ctrl Pts',(61.8523505660608,601.173966762123,105.128551144522));
#106502=CARTESIAN_POINT('Ctrl Pts',(61.8523505660607,601.73596803839,105.013844943794));
#106503=CARTESIAN_POINT('Ctrl Pts',(62.4802290518323,601.333247441326,105.347016531996));
#106504=CARTESIAN_POINT('Ctrl Pts',(61.8523505660608,601.181604534533,105.413925765979));
#106505=CARTESIAN_POINT('Ctrl Pts',(61.8523505660607,601.779310621476,105.150967761993));
#106506=CARTESIAN_POINT('Ctrl Pts',(62.5094683899049,601.398611244944,105.45806492406));
#106507=CARTESIAN_POINT('Ctrl Pts',(61.8523505660608,601.21008627854,105.567638910342));
#106508=CARTESIAN_POINT('Ctrl Pts',(61.8523505660607,601.811992484093,105.215987727826));
#106509=CARTESIAN_POINT('Ctrl Pts',(62.560332529668,601.572408710543,105.652759440274));
#106510=CARTESIAN_POINT('Ctrl Pts',(61.8523505660607,601.340706749462,105.880668070497));
#106511=CARTESIAN_POINT('Ctrl Pts',(61.8523505660607,601.898891258024,105.32976697493));
#106512=CARTESIAN_POINT('Ctrl Pts',(62.582191105061,601.68219134858,105.737292607677));
#106513=CARTESIAN_POINT('Ctrl Pts',(61.8523505660607,601.450221684905,106.040501254842));
#106514=CARTESIAN_POINT('Ctrl Pts',(61.8523505660607,601.953782539583,105.379045943916));
#106515=CARTESIAN_POINT('Ctrl Pts',(62.6128227313773,601.937633045168,105.856208205485));
#106516=CARTESIAN_POINT('Ctrl Pts',(61.8523505660607,601.779838730321,106.297756031047));
#106517=CARTESIAN_POINT('Ctrl Pts',(61.8523505660607,602.081503421665,105.448305316015));
#106518=CARTESIAN_POINT('Ctrl Pts',(62.6211772403636,602.078443985827,105.888887781001));
#106519=CARTESIAN_POINT('Ctrl Pts',(61.8523505660605,601.991235731583,106.37913780378));
#106520=CARTESIAN_POINT('Ctrl Pts',(61.8523505660607,602.151908862397,105.467304770256));
#106521=CARTESIAN_POINT('Ctrl Pts',(62.6211772316338,602.225373764374,105.888887786568));
#106522=CARTESIAN_POINT('Ctrl Pts',(61.8523505660608,602.225373764374,106.379137891718));
#106523=CARTESIAN_POINT('Ctrl Pts',(61.8523505660607,602.225373764374,105.467304788954));
#106524=CARTESIAN_POINT('Origin',(62.3523505660608,602.225373764374,105.467304788954));
#106525=CARTESIAN_POINT('Origin',(62.3523505660608,601.125373764374,99.080638124754));
#106526=CARTESIAN_POINT('Origin',(62.3523505660608,639.625373764374,99.080638124754));
#106527=CARTESIAN_POINT('Origin',(62.3523505660608,601.225373764374,105.467304788954));
#106528=CARTESIAN_POINT('Origin',(62.3523505660608,639.125373764374,105.467304788954));
#106529=CARTESIAN_POINT('Origin',(62.3523505660608,639.625373764374,99.080638124754));
#106530=CARTESIAN_POINT('Origin',(62.3523505660608,639.625373764374,99.080638124754));
#106531=CARTESIAN_POINT('Ctrl Pts',(62.6171887309608,638.947714372838,105.873295625315));
#106532=CARTESIAN_POINT('Ctrl Pts',(61.8503235888569,638.846635542666,106.34118312063));
#106533=CARTESIAN_POINT('Ctrl Pts',(61.8523518244269,639.036780009716,105.457141799944));
#106534=CARTESIAN_POINT('Ctrl Pts',(62.6232179690577,639.083373273735,105.896877360039));
#106535=CARTESIAN_POINT('Ctrl Pts',(61.8502804923024,639.057960207594,106.401111286378));
#106536=CARTESIAN_POINT('Ctrl Pts',(61.852351834326,639.10443042477,105.470809496035));
#106537=CARTESIAN_POINT('Ctrl Pts',(62.6223073524257,639.213530456068,105.893276648178));
#106538=CARTESIAN_POINT('Ctrl Pts',(61.8502874582075,639.266413948424,106.390935545101));
#106539=CARTESIAN_POINT('Ctrl Pts',(61.8523518328312,639.169332966705,105.46872895397));
#106540=CARTESIAN_POINT('Ctrl Pts',(62.6111944790013,639.40816781027,105.84996254853));
#106541=CARTESIAN_POINT('Ctrl Pts',(61.8503645972132,639.560612374044,106.285978384924));
#106542=CARTESIAN_POINT('Ctrl Pts',(61.8523518145843,639.266401094432,105.443598825812));
#106543=CARTESIAN_POINT('Ctrl Pts',(62.6052151825202,639.476286250348,105.826675971902));
#106544=CARTESIAN_POINT('Ctrl Pts',(61.8504044419249,639.656573605937,106.232002273134));
#106545=CARTESIAN_POINT('Ctrl Pts',(61.852351804766,639.300376853797,105.430084675454));
#106546=CARTESIAN_POINT('Ctrl Pts',(62.5901422537736,639.602513033697,105.768158764631));
#106547=CARTESIAN_POINT('Ctrl Pts',(61.8504991596906,639.819657772544,106.10517150034));
#106548=CARTESIAN_POINT('Ctrl Pts',(61.8523517800127,639.36334539447,105.396094036019));
#106549=CARTESIAN_POINT('Ctrl Pts',(62.5808963357417,639.662155988573,105.732338549014));
#106550=CARTESIAN_POINT('Ctrl Pts',(61.850553977998,639.88872891337,106.032376080376));
#106551=CARTESIAN_POINT('Ctrl Pts',(61.8523517648272,639.393103899509,105.375274204658));
#106552=CARTESIAN_POINT('Ctrl Pts',(62.5598410210075,639.770930402132,105.651098312915));
#106553=CARTESIAN_POINT('Ctrl Pts',(61.8506699946354,640.00044371228,105.879793343696));
#106554=CARTESIAN_POINT('Ctrl Pts',(61.8523517302416,639.447386384734,105.328001115495));
#106555=CARTESIAN_POINT('Ctrl Pts',(62.5481339335838,639.819816105116,105.606071364224));
#106556=CARTESIAN_POINT('Ctrl Pts',(61.8507300636749,640.043582274495,105.801418515785));
#106557=CARTESIAN_POINT('Ctrl Pts',(61.8523517110091,639.471787510695,105.301776292401));
#106558=CARTESIAN_POINT('Ctrl Pts',(62.5097505487502,639.951569950465,105.459135338167));
#106559=CARTESIAN_POINT('Ctrl Pts',(61.8509087517028,640.140868692571,105.56941884666));
#106560=CARTESIAN_POINT('Ctrl Pts',(61.8523516479419,639.537567153372,105.216084761092));
#106561=CARTESIAN_POINT('Ctrl Pts',(62.4805155321142,640.01702622273,105.348095923452));
#106562=CARTESIAN_POINT('Ctrl Pts',(61.8510283348443,640.169352447589,105.41549517911));
#106563=CARTESIAN_POINT('Ctrl Pts',(61.852351599895,639.570263865268,105.151188011025));
#106564=CARTESIAN_POINT('Ctrl Pts',(62.4055323875921,640.121714641665,105.066534511825));
#106565=CARTESIAN_POINT('Ctrl Pts',(61.8512890952677,640.178381817406,105.076238326916));
#106566=CARTESIAN_POINT('Ctrl Pts',(61.8523514766257,639.622591495187,104.986123737673));
#106567=CARTESIAN_POINT('Ctrl Pts',(62.3596802853423,640.138657441275,104.896768194161));
#106568=CARTESIAN_POINT('Ctrl Pts',(61.8514233185298,640.143976932967,104.898778401034));
#106569=CARTESIAN_POINT('Ctrl Pts',(61.8523514012223,639.631092470791,104.886221982453));
#106570=CARTESIAN_POINT('Ctrl Pts',(62.311824621281,640.115332282486,104.722478050629));
#106571=CARTESIAN_POINT('Ctrl Pts',(61.8515480494827,640.078231673359,104.72693455747));
#106572=CARTESIAN_POINT('Ctrl Pts',(61.852351322506,639.619489084467,104.783211384763));
#106573=CARTESIAN_POINT('Origin',(62.3523505660608,639.625373764374,104.870738441723));
#106574=CARTESIAN_POINT('Origin',(62.3523505660608,639.625373764374,0.));
#130897=UNCERTAINTY_MEASURE_WITH_UNIT(LENGTH_MEASURE(0.01),#130911,
'DISTANCE_ACCURACY_VALUE',
'Maximum model space distance between geometric entities at asserted c
onnectivities');
#130900=UNCERTAINTY_MEASURE_WITH_UNIT(LENGTH_MEASURE(0.01),#130911,
'DISTANCE_ACCURACY_VALUE',
'Maximum model space distance between geometric entities at asserted c
onnectivities');
#130907=(
GEOMETRIC_REPRESENTATION_CONTEXT(3)
GLOBAL_UNCERTAINTY_ASSIGNED_CONTEXT((#130897))
GLOBAL_UNIT_ASSIGNED_CONTEXT((#130911,#130913,#130914))
REPRESENTATION_CONTEXT('','3D')
);
#130910=(
GEOMETRIC_REPRESENTATION_CONTEXT(3)
GLOBAL_UNCERTAINTY_ASSIGNED_CONTEXT((#130900))
GLOBAL_UNIT_ASSIGNED_CONTEXT((#130911,#130913,#130914))
REPRESENTATION_CONTEXT('','3D')
);
#130911=(
LENGTH_UNIT()
NAMED_UNIT(*)
SI_UNIT(.MILLI.,.METRE.)
);
#130913=(
NAMED_UNIT(*)
PLANE_ANGLE_UNIT()
SI_UNIT($,.RADIAN.)
);
#130914=(
NAMED_UNIT(*)
SI_UNIT($,.STERADIAN.)
SOLID_ANGLE_UNIT()
);
#130921=SHAPE_DEFINITION_REPRESENTATION(#130930,#130947);
#130930=PRODUCT_DEFINITION_SHAPE('',$,#130957);
#130947=SHAPE_REPRESENTATION('',(#48753),#130907);
#130950=PRODUCT_DEFINITION_CONTEXT('part definition',#130979,'design');
#130957=PRODUCT_DEFINITION('Component6','Component6',#130966,#130950);
#130966=PRODUCT_DEFINITION_FORMATION('',$,#130987);
#130979=APPLICATION_CONTEXT(
'Core Data for Automotive Mechanical Design Process');
#130980=PRODUCT_CONTEXT('part definition',#130979,'mechanical');
#130987=PRODUCT('Component6','Component6',$,(#130980));
#130991=PRESENTATION_STYLE_ASSIGNMENT((#130993));
#130993=SURFACE_STYLE_USAGE(.BOTH.,#130995);
#130995=SURFACE_SIDE_STYLE('',(#130997));
#130997=SURFACE_STYLE_FILL_AREA(#130999);
#130999=FILL_AREA_STYLE('Opaque(202,209,238)',(#131001));
#131001=FILL_AREA_STYLE_COLOUR('Opaque(202,209,238)',#131003);
#131003=COLOUR_RGB('Opaque(202,209,238)', 0.40784314, 0.44705882, 0.49803922);
ENDSEC;
END-ISO-10303-21;
